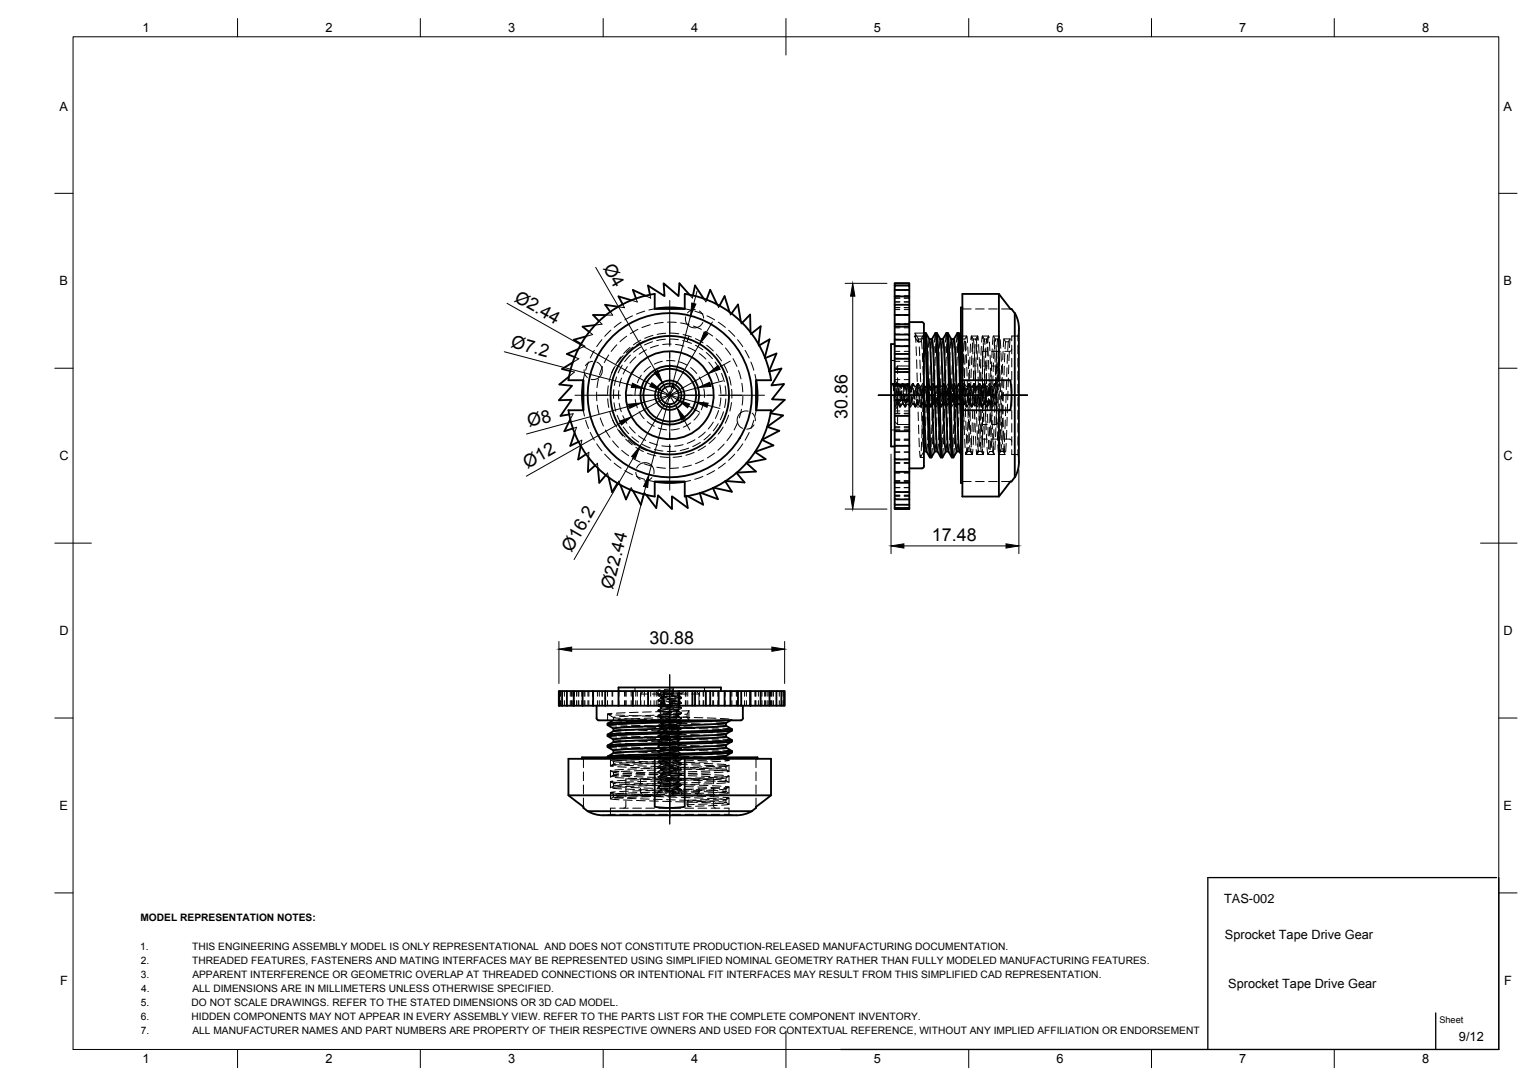
ISO-10303-21;
HEADER;
/* Generated by software containing ST-Developer
 * from STEP Tools, Inc. (www.steptools.com) 
 */

FILE_DESCRIPTION(
/* description */ ('STEP AP214'),
/* implementation_level */ '2;1');

FILE_NAME(
/* name */ 'Sprocket Tape Drive Gear.step',
/* time_stamp */ '2026-11-04T19:38:14-08:00',
/* author */ (''),
/* organization */ (''),
/* preprocessor_version */ 'ST-DEVELOPER v20.2',
/* originating_system */ 'Autodesk Translation Framework v15.17.0.0',
/* authorisation */ '');

FILE_SCHEMA (('AUTOMOTIVE_DESIGN { 1 0 10303 214 3 1 1 }'));
ENDSEC;

DATA;
#10=MECHANICAL_DESIGN_GEOMETRIC_PRESENTATION_REPRESENTATION('',(#476),#36668);
#59=(
BOUNDED_CURVE()
B_SPLINE_CURVE(2,(#28963,#28964,#28965,#28966,#28967,#28968,#28969),
 .UNSPECIFIED.,.F.,.F.)
B_SPLINE_CURVE_WITH_KNOTS((3,2,2,3),(0.975,0.983333333333333,0.991666666666667,
1.),.UNSPECIFIED.)
CURVE()
GEOMETRIC_REPRESENTATION_ITEM()
RATIONAL_B_SPLINE_CURVE((1.,0.866025403784439,1.,0.866025403784439,1.,0.866025403784439,
1.))
REPRESENTATION_ITEM('')
);
#60=(
BOUNDED_CURVE()
B_SPLINE_CURVE(2,(#28975,#28976,#28977,#28978,#28979,#28980,#28981),
 .UNSPECIFIED.,.F.,.F.)
B_SPLINE_CURVE_WITH_KNOTS((3,2,2,3),(0.975,0.983333333333333,0.991666666666667,
1.),.UNSPECIFIED.)
CURVE()
GEOMETRIC_REPRESENTATION_ITEM()
RATIONAL_B_SPLINE_CURVE((1.,0.866025403784439,1.,0.866025403784439,1.,0.866025403784439,
1.))
REPRESENTATION_ITEM('')
);
#61=(
BOUNDED_CURVE()
B_SPLINE_CURVE(2,(#28984,#28985,#28986,#28987,#28988,#28989,#28990),
 .UNSPECIFIED.,.F.,.F.)
B_SPLINE_CURVE_WITH_KNOTS((3,2,2,3),(0.975,0.983333333333333,0.991666666666667,
1.),.UNSPECIFIED.)
CURVE()
GEOMETRIC_REPRESENTATION_ITEM()
RATIONAL_B_SPLINE_CURVE((1.,0.866025403784439,1.,0.866025403784439,1.,0.866025403784439,
1.))
REPRESENTATION_ITEM('')
);
#62=(
BOUNDED_CURVE()
B_SPLINE_CURVE(2,(#28995,#28996,#28997,#28998,#28999,#29000,#29001,#29002,
#29003,#29004,#29005,#29006,#29007),.UNSPECIFIED.,.F.,.F.)
B_SPLINE_CURVE_WITH_KNOTS((3,2,2,2,2,2,3),(0.925,0.933333333333333,0.941666666666667,
0.95,0.958333333333333,0.966666666666667,0.975),.UNSPECIFIED.)
CURVE()
GEOMETRIC_REPRESENTATION_ITEM()
RATIONAL_B_SPLINE_CURVE((1.,0.866025403784439,1.,0.866025403784439,1.,0.866025403784439,
1.,0.866025403784439,1.,0.866025403784439,1.,0.866025403784439,1.))
REPRESENTATION_ITEM('')
);
#63=(
BOUNDED_CURVE()
B_SPLINE_CURVE(2,(#29008,#29009,#29010,#29011,#29012,#29013,#29014,#29015,
#29016,#29017,#29018,#29019,#29020),.UNSPECIFIED.,.F.,.F.)
B_SPLINE_CURVE_WITH_KNOTS((3,2,2,2,2,2,3),(0.925,0.933333333333333,0.941666666666667,
0.95,0.958333333333333,0.966666666666667,0.975),.UNSPECIFIED.)
CURVE()
GEOMETRIC_REPRESENTATION_ITEM()
RATIONAL_B_SPLINE_CURVE((1.,0.866025403784439,1.,0.866025403784439,1.,0.866025403784439,
1.,0.866025403784439,1.,0.866025403784439,1.,0.866025403784439,1.))
REPRESENTATION_ITEM('')
);
#64=(
BOUNDED_CURVE()
B_SPLINE_CURVE(2,(#29025,#29026,#29027,#29028,#29029,#29030,#29031,#29032,
#29033,#29034,#29035,#29036,#29037),.UNSPECIFIED.,.F.,.F.)
B_SPLINE_CURVE_WITH_KNOTS((3,2,2,2,2,2,3),(0.875,0.883333333333333,0.891666666666667,
0.9,0.908333333333333,0.916666666666667,0.925),.UNSPECIFIED.)
CURVE()
GEOMETRIC_REPRESENTATION_ITEM()
RATIONAL_B_SPLINE_CURVE((1.,0.866025403784439,1.,0.866025403784439,1.,0.866025403784439,
1.,0.866025403784439,1.,0.866025403784439,1.,0.866025403784439,1.))
REPRESENTATION_ITEM('')
);
#65=(
BOUNDED_CURVE()
B_SPLINE_CURVE(2,(#29038,#29039,#29040,#29041,#29042,#29043,#29044,#29045,
#29046,#29047,#29048,#29049,#29050),.UNSPECIFIED.,.F.,.F.)
B_SPLINE_CURVE_WITH_KNOTS((3,2,2,2,2,2,3),(0.875,0.883333333333333,0.891666666666667,
0.9,0.908333333333333,0.916666666666667,0.925),.UNSPECIFIED.)
CURVE()
GEOMETRIC_REPRESENTATION_ITEM()
RATIONAL_B_SPLINE_CURVE((1.,0.866025403784439,1.,0.866025403784439,1.,0.866025403784439,
1.,0.866025403784439,1.,0.866025403784439,1.,0.866025403784439,1.))
REPRESENTATION_ITEM('')
);
#66=(
BOUNDED_CURVE()
B_SPLINE_CURVE(2,(#29055,#29056,#29057,#29058,#29059,#29060,#29061,#29062,
#29063,#29064,#29065,#29066,#29067),.UNSPECIFIED.,.F.,.F.)
B_SPLINE_CURVE_WITH_KNOTS((3,2,2,2,2,2,3),(0.825,0.833333333333333,0.841666666666667,
0.85,0.858333333333333,0.866666666666667,0.875),.UNSPECIFIED.)
CURVE()
GEOMETRIC_REPRESENTATION_ITEM()
RATIONAL_B_SPLINE_CURVE((1.,0.866025403784439,1.,0.866025403784439,1.,0.866025403784439,
1.,0.866025403784439,1.,0.866025403784439,1.,0.866025403784439,1.))
REPRESENTATION_ITEM('')
);
#67=(
BOUNDED_CURVE()
B_SPLINE_CURVE(2,(#29068,#29069,#29070,#29071,#29072,#29073,#29074,#29075,
#29076,#29077,#29078,#29079,#29080),.UNSPECIFIED.,.F.,.F.)
B_SPLINE_CURVE_WITH_KNOTS((3,2,2,2,2,2,3),(0.825,0.833333333333333,0.841666666666667,
0.85,0.858333333333333,0.866666666666667,0.875),.UNSPECIFIED.)
CURVE()
GEOMETRIC_REPRESENTATION_ITEM()
RATIONAL_B_SPLINE_CURVE((1.,0.866025403784439,1.,0.866025403784439,1.,0.866025403784439,
1.,0.866025403784439,1.,0.866025403784439,1.,0.866025403784439,1.))
REPRESENTATION_ITEM('')
);
#68=(
BOUNDED_CURVE()
B_SPLINE_CURVE(2,(#29085,#29086,#29087,#29088,#29089,#29090,#29091,#29092,
#29093,#29094,#29095,#29096,#29097),.UNSPECIFIED.,.F.,.F.)
B_SPLINE_CURVE_WITH_KNOTS((3,2,2,2,2,2,3),(0.775,0.783333333333333,0.791666666666667,
0.8,0.808333333333333,0.816666666666667,0.825),.UNSPECIFIED.)
CURVE()
GEOMETRIC_REPRESENTATION_ITEM()
RATIONAL_B_SPLINE_CURVE((1.,0.866025403784439,1.,0.866025403784439,1.,0.866025403784439,
1.,0.866025403784439,1.,0.866025403784439,1.,0.866025403784439,1.))
REPRESENTATION_ITEM('')
);
#69=(
BOUNDED_CURVE()
B_SPLINE_CURVE(2,(#29098,#29099,#29100,#29101,#29102,#29103,#29104,#29105,
#29106,#29107,#29108,#29109,#29110),.UNSPECIFIED.,.F.,.F.)
B_SPLINE_CURVE_WITH_KNOTS((3,2,2,2,2,2,3),(0.775,0.783333333333333,0.791666666666667,
0.8,0.808333333333333,0.816666666666667,0.825),.UNSPECIFIED.)
CURVE()
GEOMETRIC_REPRESENTATION_ITEM()
RATIONAL_B_SPLINE_CURVE((1.,0.866025403784439,1.,0.866025403784439,1.,0.866025403784439,
1.,0.866025403784439,1.,0.866025403784439,1.,0.866025403784439,1.))
REPRESENTATION_ITEM('')
);
#70=(
BOUNDED_CURVE()
B_SPLINE_CURVE(2,(#29115,#29116,#29117,#29118,#29119,#29120,#29121,#29122,
#29123,#29124,#29125,#29126,#29127),.UNSPECIFIED.,.F.,.F.)
B_SPLINE_CURVE_WITH_KNOTS((3,2,2,2,2,2,3),(0.725,0.733333333333333,0.741666666666667,
0.75,0.758333333333333,0.766666666666667,0.775),.UNSPECIFIED.)
CURVE()
GEOMETRIC_REPRESENTATION_ITEM()
RATIONAL_B_SPLINE_CURVE((1.,0.866025403784439,1.,0.866025403784439,1.,0.866025403784439,
1.,0.866025403784439,1.,0.866025403784439,1.,0.866025403784439,1.))
REPRESENTATION_ITEM('')
);
#71=(
BOUNDED_CURVE()
B_SPLINE_CURVE(2,(#29128,#29129,#29130,#29131,#29132,#29133,#29134,#29135,
#29136,#29137,#29138,#29139,#29140),.UNSPECIFIED.,.F.,.F.)
B_SPLINE_CURVE_WITH_KNOTS((3,2,2,2,2,2,3),(0.725,0.733333333333333,0.741666666666667,
0.75,0.758333333333333,0.766666666666667,0.775),.UNSPECIFIED.)
CURVE()
GEOMETRIC_REPRESENTATION_ITEM()
RATIONAL_B_SPLINE_CURVE((1.,0.866025403784439,1.,0.866025403784439,1.,0.866025403784439,
1.,0.866025403784439,1.,0.866025403784439,1.,0.866025403784439,1.))
REPRESENTATION_ITEM('')
);
#72=(
BOUNDED_CURVE()
B_SPLINE_CURVE(2,(#29145,#29146,#29147,#29148,#29149,#29150,#29151,#29152,
#29153,#29154,#29155,#29156,#29157),.UNSPECIFIED.,.F.,.F.)
B_SPLINE_CURVE_WITH_KNOTS((3,2,2,2,2,2,3),(0.675,0.683333333333333,0.691666666666667,
0.7,0.708333333333333,0.716666666666667,0.725),.UNSPECIFIED.)
CURVE()
GEOMETRIC_REPRESENTATION_ITEM()
RATIONAL_B_SPLINE_CURVE((1.,0.866025403784439,1.,0.866025403784439,1.,0.866025403784439,
1.,0.866025403784439,1.,0.866025403784439,1.,0.866025403784439,1.))
REPRESENTATION_ITEM('')
);
#73=(
BOUNDED_CURVE()
B_SPLINE_CURVE(2,(#29158,#29159,#29160,#29161,#29162,#29163,#29164,#29165,
#29166,#29167,#29168,#29169,#29170),.UNSPECIFIED.,.F.,.F.)
B_SPLINE_CURVE_WITH_KNOTS((3,2,2,2,2,2,3),(0.675,0.683333333333333,0.691666666666667,
0.7,0.708333333333333,0.716666666666667,0.725),.UNSPECIFIED.)
CURVE()
GEOMETRIC_REPRESENTATION_ITEM()
RATIONAL_B_SPLINE_CURVE((1.,0.866025403784439,1.,0.866025403784439,1.,0.866025403784439,
1.,0.866025403784439,1.,0.866025403784439,1.,0.866025403784439,1.))
REPRESENTATION_ITEM('')
);
#74=(
BOUNDED_CURVE()
B_SPLINE_CURVE(2,(#29175,#29176,#29177,#29178,#29179,#29180,#29181,#29182,
#29183,#29184,#29185,#29186,#29187),.UNSPECIFIED.,.F.,.F.)
B_SPLINE_CURVE_WITH_KNOTS((3,2,2,2,2,2,3),(0.625,0.633333333333333,0.641666666666667,
0.65,0.658333333333333,0.666666666666667,0.675),.UNSPECIFIED.)
CURVE()
GEOMETRIC_REPRESENTATION_ITEM()
RATIONAL_B_SPLINE_CURVE((1.,0.866025403784439,1.,0.866025403784439,1.,0.866025403784439,
1.,0.866025403784439,1.,0.866025403784439,1.,0.866025403784439,1.))
REPRESENTATION_ITEM('')
);
#75=(
BOUNDED_CURVE()
B_SPLINE_CURVE(2,(#29188,#29189,#29190,#29191,#29192,#29193,#29194,#29195,
#29196,#29197,#29198,#29199,#29200),.UNSPECIFIED.,.F.,.F.)
B_SPLINE_CURVE_WITH_KNOTS((3,2,2,2,2,2,3),(0.625,0.633333333333333,0.641666666666667,
0.65,0.658333333333333,0.666666666666667,0.675),.UNSPECIFIED.)
CURVE()
GEOMETRIC_REPRESENTATION_ITEM()
RATIONAL_B_SPLINE_CURVE((1.,0.866025403784439,1.,0.866025403784439,1.,0.866025403784439,
1.,0.866025403784439,1.,0.866025403784439,1.,0.866025403784439,1.))
REPRESENTATION_ITEM('')
);
#76=(
BOUNDED_CURVE()
B_SPLINE_CURVE(2,(#29205,#29206,#29207,#29208,#29209,#29210,#29211,#29212,
#29213,#29214,#29215,#29216,#29217),.UNSPECIFIED.,.F.,.F.)
B_SPLINE_CURVE_WITH_KNOTS((3,2,2,2,2,2,3),(0.575,0.583333333333333,0.591666666666667,
0.6,0.608333333333333,0.616666666666667,0.625),.UNSPECIFIED.)
CURVE()
GEOMETRIC_REPRESENTATION_ITEM()
RATIONAL_B_SPLINE_CURVE((1.,0.866025403784439,1.,0.866025403784439,1.,0.866025403784439,
1.,0.866025403784439,1.,0.866025403784439,1.,0.866025403784439,1.))
REPRESENTATION_ITEM('')
);
#77=(
BOUNDED_CURVE()
B_SPLINE_CURVE(2,(#29218,#29219,#29220,#29221,#29222,#29223,#29224,#29225,
#29226,#29227,#29228,#29229,#29230),.UNSPECIFIED.,.F.,.F.)
B_SPLINE_CURVE_WITH_KNOTS((3,2,2,2,2,2,3),(0.575,0.583333333333333,0.591666666666667,
0.6,0.608333333333333,0.616666666666667,0.625),.UNSPECIFIED.)
CURVE()
GEOMETRIC_REPRESENTATION_ITEM()
RATIONAL_B_SPLINE_CURVE((1.,0.866025403784439,1.,0.866025403784439,1.,0.866025403784439,
1.,0.866025403784439,1.,0.866025403784439,1.,0.866025403784439,1.))
REPRESENTATION_ITEM('')
);
#78=(
BOUNDED_CURVE()
B_SPLINE_CURVE(2,(#29235,#29236,#29237,#29238,#29239,#29240,#29241,#29242,
#29243,#29244,#29245,#29246,#29247),.UNSPECIFIED.,.F.,.F.)
B_SPLINE_CURVE_WITH_KNOTS((3,2,2,2,2,2,3),(0.525,0.533333333333333,0.541666666666667,
0.55,0.558333333333333,0.566666666666667,0.575),.UNSPECIFIED.)
CURVE()
GEOMETRIC_REPRESENTATION_ITEM()
RATIONAL_B_SPLINE_CURVE((1.,0.866025403784439,1.,0.866025403784439,1.,0.866025403784439,
1.,0.866025403784439,1.,0.866025403784439,1.,0.866025403784439,1.))
REPRESENTATION_ITEM('')
);
#79=(
BOUNDED_CURVE()
B_SPLINE_CURVE(2,(#29248,#29249,#29250,#29251,#29252,#29253,#29254,#29255,
#29256,#29257,#29258,#29259,#29260),.UNSPECIFIED.,.F.,.F.)
B_SPLINE_CURVE_WITH_KNOTS((3,2,2,2,2,2,3),(0.525,0.533333333333333,0.541666666666667,
0.55,0.558333333333333,0.566666666666667,0.575),.UNSPECIFIED.)
CURVE()
GEOMETRIC_REPRESENTATION_ITEM()
RATIONAL_B_SPLINE_CURVE((1.,0.866025403784439,1.,0.866025403784439,1.,0.866025403784439,
1.,0.866025403784439,1.,0.866025403784439,1.,0.866025403784439,1.))
REPRESENTATION_ITEM('')
);
#80=(
BOUNDED_CURVE()
B_SPLINE_CURVE(2,(#29265,#29266,#29267,#29268,#29269,#29270,#29271,#29272,
#29273,#29274,#29275,#29276,#29277),.UNSPECIFIED.,.F.,.F.)
B_SPLINE_CURVE_WITH_KNOTS((3,2,2,2,2,2,3),(0.475,0.483333333333333,0.491666666666667,
0.5,0.508333333333333,0.516666666666667,0.525),.UNSPECIFIED.)
CURVE()
GEOMETRIC_REPRESENTATION_ITEM()
RATIONAL_B_SPLINE_CURVE((1.,0.866025403784439,1.,0.866025403784439,1.,0.866025403784439,
1.,0.866025403784439,1.,0.866025403784439,1.,0.866025403784439,1.))
REPRESENTATION_ITEM('')
);
#81=(
BOUNDED_CURVE()
B_SPLINE_CURVE(2,(#29278,#29279,#29280,#29281,#29282,#29283,#29284,#29285,
#29286,#29287,#29288,#29289,#29290),.UNSPECIFIED.,.F.,.F.)
B_SPLINE_CURVE_WITH_KNOTS((3,2,2,2,2,2,3),(0.475,0.483333333333333,0.491666666666667,
0.5,0.508333333333333,0.516666666666667,0.525),.UNSPECIFIED.)
CURVE()
GEOMETRIC_REPRESENTATION_ITEM()
RATIONAL_B_SPLINE_CURVE((1.,0.866025403784439,1.,0.866025403784439,1.,0.866025403784439,
1.,0.866025403784439,1.,0.866025403784439,1.,0.866025403784439,1.))
REPRESENTATION_ITEM('')
);
#82=(
BOUNDED_CURVE()
B_SPLINE_CURVE(2,(#29295,#29296,#29297,#29298,#29299,#29300,#29301,#29302,
#29303,#29304,#29305,#29306,#29307),.UNSPECIFIED.,.F.,.F.)
B_SPLINE_CURVE_WITH_KNOTS((3,2,2,2,2,2,3),(0.425,0.433333333333334,0.441666666666666,
0.45,0.458333333333333,0.466666666666667,0.475),.UNSPECIFIED.)
CURVE()
GEOMETRIC_REPRESENTATION_ITEM()
RATIONAL_B_SPLINE_CURVE((1.,0.866025403784439,1.,0.866025403784439,1.,0.866025403784439,
1.,0.866025403784439,1.,0.866025403784439,1.,0.866025403784439,1.))
REPRESENTATION_ITEM('')
);
#83=(
BOUNDED_CURVE()
B_SPLINE_CURVE(2,(#29308,#29309,#29310,#29311,#29312,#29313,#29314,#29315,
#29316,#29317,#29318,#29319,#29320),.UNSPECIFIED.,.F.,.F.)
B_SPLINE_CURVE_WITH_KNOTS((3,2,2,2,2,2,3),(0.425,0.433333333333334,0.441666666666666,
0.45,0.458333333333333,0.466666666666667,0.475),.UNSPECIFIED.)
CURVE()
GEOMETRIC_REPRESENTATION_ITEM()
RATIONAL_B_SPLINE_CURVE((1.,0.866025403784439,1.,0.866025403784439,1.,0.866025403784439,
1.,0.866025403784439,1.,0.866025403784439,1.,0.866025403784439,1.))
REPRESENTATION_ITEM('')
);
#84=(
BOUNDED_CURVE()
B_SPLINE_CURVE(2,(#29325,#29326,#29327,#29328,#29329,#29330,#29331,#29332,
#29333,#29334,#29335,#29336,#29337),.UNSPECIFIED.,.F.,.F.)
B_SPLINE_CURVE_WITH_KNOTS((3,2,2,2,2,2,3),(0.375,0.383333333333334,0.391666666666666,
0.4,0.408333333333334,0.416666666666667,0.425),.UNSPECIFIED.)
CURVE()
GEOMETRIC_REPRESENTATION_ITEM()
RATIONAL_B_SPLINE_CURVE((1.,0.866025403784439,1.,0.866025403784439,1.,0.866025403784439,
1.,0.866025403784439,1.,0.866025403784439,1.,0.866025403784439,1.))
REPRESENTATION_ITEM('')
);
#85=(
BOUNDED_CURVE()
B_SPLINE_CURVE(2,(#29338,#29339,#29340,#29341,#29342,#29343,#29344,#29345,
#29346,#29347,#29348,#29349,#29350),.UNSPECIFIED.,.F.,.F.)
B_SPLINE_CURVE_WITH_KNOTS((3,2,2,2,2,2,3),(0.375,0.383333333333334,0.391666666666666,
0.4,0.408333333333334,0.416666666666667,0.425),.UNSPECIFIED.)
CURVE()
GEOMETRIC_REPRESENTATION_ITEM()
RATIONAL_B_SPLINE_CURVE((1.,0.866025403784439,1.,0.866025403784439,1.,0.866025403784439,
1.,0.866025403784439,1.,0.866025403784439,1.,0.866025403784439,1.))
REPRESENTATION_ITEM('')
);
#86=(
BOUNDED_CURVE()
B_SPLINE_CURVE(2,(#29355,#29356,#29357,#29358,#29359,#29360,#29361,#29362,
#29363,#29364,#29365,#29366,#29367),.UNSPECIFIED.,.F.,.F.)
B_SPLINE_CURVE_WITH_KNOTS((3,2,2,2,2,2,3),(0.325,0.333333333333334,0.341666666666667,
0.35,0.358333333333334,0.366666666666666,0.375),.UNSPECIFIED.)
CURVE()
GEOMETRIC_REPRESENTATION_ITEM()
RATIONAL_B_SPLINE_CURVE((1.,0.866025403784439,1.,0.866025403784439,1.,0.866025403784439,
1.,0.866025403784439,1.,0.866025403784439,1.,0.866025403784439,1.))
REPRESENTATION_ITEM('')
);
#87=(
BOUNDED_CURVE()
B_SPLINE_CURVE(2,(#29368,#29369,#29370,#29371,#29372,#29373,#29374,#29375,
#29376,#29377,#29378,#29379,#29380),.UNSPECIFIED.,.F.,.F.)
B_SPLINE_CURVE_WITH_KNOTS((3,2,2,2,2,2,3),(0.325,0.333333333333334,0.341666666666667,
0.35,0.358333333333334,0.366666666666666,0.375),.UNSPECIFIED.)
CURVE()
GEOMETRIC_REPRESENTATION_ITEM()
RATIONAL_B_SPLINE_CURVE((1.,0.866025403784439,1.,0.866025403784439,1.,0.866025403784439,
1.,0.866025403784439,1.,0.866025403784439,1.,0.866025403784439,1.))
REPRESENTATION_ITEM('')
);
#88=(
BOUNDED_CURVE()
B_SPLINE_CURVE(2,(#29385,#29386,#29387,#29388,#29389,#29390,#29391,#29392,
#29393,#29394,#29395,#29396,#29397),.UNSPECIFIED.,.F.,.F.)
B_SPLINE_CURVE_WITH_KNOTS((3,2,2,2,2,2,3),(0.275,0.283333333333334,0.291666666666667,
0.3,0.308333333333334,0.316666666666666,0.325),.UNSPECIFIED.)
CURVE()
GEOMETRIC_REPRESENTATION_ITEM()
RATIONAL_B_SPLINE_CURVE((1.,0.866025403784439,1.,0.866025403784439,1.,0.866025403784439,
1.,0.866025403784439,1.,0.866025403784439,1.,0.866025403784439,1.))
REPRESENTATION_ITEM('')
);
#89=(
BOUNDED_CURVE()
B_SPLINE_CURVE(2,(#29398,#29399,#29400,#29401,#29402,#29403,#29404,#29405,
#29406,#29407,#29408,#29409,#29410),.UNSPECIFIED.,.F.,.F.)
B_SPLINE_CURVE_WITH_KNOTS((3,2,2,2,2,2,3),(0.275,0.283333333333334,0.291666666666667,
0.3,0.308333333333334,0.316666666666666,0.325),.UNSPECIFIED.)
CURVE()
GEOMETRIC_REPRESENTATION_ITEM()
RATIONAL_B_SPLINE_CURVE((1.,0.866025403784439,1.,0.866025403784439,1.,0.866025403784439,
1.,0.866025403784439,1.,0.866025403784439,1.,0.866025403784439,1.))
REPRESENTATION_ITEM('')
);
#90=(
BOUNDED_CURVE()
B_SPLINE_CURVE(2,(#29415,#29416,#29417,#29418,#29419,#29420,#29421,#29422,
#29423,#29424,#29425,#29426,#29427),.UNSPECIFIED.,.F.,.F.)
B_SPLINE_CURVE_WITH_KNOTS((3,2,2,2,2,2,3),(0.225,0.233333333333334,0.241666666666667,
0.25,0.258333333333334,0.266666666666666,0.275),.UNSPECIFIED.)
CURVE()
GEOMETRIC_REPRESENTATION_ITEM()
RATIONAL_B_SPLINE_CURVE((1.,0.866025403784439,1.,0.866025403784439,1.,0.866025403784439,
1.,0.866025403784439,1.,0.866025403784439,1.,0.866025403784439,1.))
REPRESENTATION_ITEM('')
);
#91=(
BOUNDED_CURVE()
B_SPLINE_CURVE(2,(#29428,#29429,#29430,#29431,#29432,#29433,#29434,#29435,
#29436,#29437,#29438,#29439,#29440),.UNSPECIFIED.,.F.,.F.)
B_SPLINE_CURVE_WITH_KNOTS((3,2,2,2,2,2,3),(0.225,0.233333333333334,0.241666666666667,
0.25,0.258333333333334,0.266666666666666,0.275),.UNSPECIFIED.)
CURVE()
GEOMETRIC_REPRESENTATION_ITEM()
RATIONAL_B_SPLINE_CURVE((1.,0.866025403784439,1.,0.866025403784439,1.,0.866025403784439,
1.,0.866025403784439,1.,0.866025403784439,1.,0.866025403784439,1.))
REPRESENTATION_ITEM('')
);
#92=(
BOUNDED_CURVE()
B_SPLINE_CURVE(2,(#29445,#29446,#29447,#29448,#29449,#29450,#29451,#29452,
#29453,#29454,#29455,#29456,#29457),.UNSPECIFIED.,.F.,.F.)
B_SPLINE_CURVE_WITH_KNOTS((3,2,2,2,2,2,3),(0.175,0.183333333333334,0.191666666666667,
0.2,0.208333333333334,0.216666666666667,0.225),.UNSPECIFIED.)
CURVE()
GEOMETRIC_REPRESENTATION_ITEM()
RATIONAL_B_SPLINE_CURVE((1.,0.866025403784439,1.,0.866025403784439,1.,0.866025403784439,
1.,0.866025403784439,1.,0.866025403784439,1.,0.866025403784439,1.))
REPRESENTATION_ITEM('')
);
#93=(
BOUNDED_CURVE()
B_SPLINE_CURVE(2,(#29458,#29459,#29460,#29461,#29462,#29463,#29464,#29465,
#29466,#29467,#29468,#29469,#29470),.UNSPECIFIED.,.F.,.F.)
B_SPLINE_CURVE_WITH_KNOTS((3,2,2,2,2,2,3),(0.175,0.183333333333334,0.191666666666667,
0.2,0.208333333333334,0.216666666666667,0.225),.UNSPECIFIED.)
CURVE()
GEOMETRIC_REPRESENTATION_ITEM()
RATIONAL_B_SPLINE_CURVE((1.,0.866025403784439,1.,0.866025403784439,1.,0.866025403784439,
1.,0.866025403784439,1.,0.866025403784439,1.,0.866025403784439,1.))
REPRESENTATION_ITEM('')
);
#94=(
BOUNDED_CURVE()
B_SPLINE_CURVE(2,(#29475,#29476,#29477,#29478,#29479,#29480,#29481,#29482,
#29483,#29484,#29485,#29486,#29487),.UNSPECIFIED.,.F.,.F.)
B_SPLINE_CURVE_WITH_KNOTS((3,2,2,2,2,2,3),(0.125,0.133333333333333,0.141666666666667,
0.15,0.158333333333333,0.166666666666667,0.175),.UNSPECIFIED.)
CURVE()
GEOMETRIC_REPRESENTATION_ITEM()
RATIONAL_B_SPLINE_CURVE((1.,0.866025403784439,1.,0.866025403784439,1.,0.866025403784439,
1.,0.866025403784439,1.,0.866025403784439,1.,0.866025403784439,1.))
REPRESENTATION_ITEM('')
);
#95=(
BOUNDED_CURVE()
B_SPLINE_CURVE(2,(#29488,#29489,#29490,#29491,#29492,#29493,#29494,#29495,
#29496,#29497,#29498,#29499,#29500),.UNSPECIFIED.,.F.,.F.)
B_SPLINE_CURVE_WITH_KNOTS((3,2,2,2,2,2,3),(0.125,0.133333333333333,0.141666666666667,
0.15,0.158333333333333,0.166666666666667,0.175),.UNSPECIFIED.)
CURVE()
GEOMETRIC_REPRESENTATION_ITEM()
RATIONAL_B_SPLINE_CURVE((1.,0.866025403784439,1.,0.866025403784439,1.,0.866025403784439,
1.,0.866025403784439,1.,0.866025403784439,1.,0.866025403784439,1.))
REPRESENTATION_ITEM('')
);
#96=(
BOUNDED_CURVE()
B_SPLINE_CURVE(2,(#29505,#29506,#29507,#29508,#29509,#29510,#29511,#29512,
#29513,#29514,#29515,#29516,#29517),.UNSPECIFIED.,.F.,.F.)
B_SPLINE_CURVE_WITH_KNOTS((3,2,2,2,2,2,3),(0.075,0.0833333333333333,0.0916666666666667,
0.1,0.108333333333333,0.116666666666667,0.125),.UNSPECIFIED.)
CURVE()
GEOMETRIC_REPRESENTATION_ITEM()
RATIONAL_B_SPLINE_CURVE((1.,0.866025403784439,1.,0.866025403784439,1.,0.866025403784439,
1.,0.866025403784439,1.,0.866025403784439,1.,0.866025403784439,1.))
REPRESENTATION_ITEM('')
);
#97=(
BOUNDED_CURVE()
B_SPLINE_CURVE(2,(#29518,#29519,#29520,#29521,#29522,#29523,#29524,#29525,
#29526,#29527,#29528,#29529,#29530),.UNSPECIFIED.,.F.,.F.)
B_SPLINE_CURVE_WITH_KNOTS((3,2,2,2,2,2,3),(0.075,0.0833333333333333,0.0916666666666667,
0.1,0.108333333333333,0.116666666666667,0.125),.UNSPECIFIED.)
CURVE()
GEOMETRIC_REPRESENTATION_ITEM()
RATIONAL_B_SPLINE_CURVE((1.,0.866025403784439,1.,0.866025403784439,1.,0.866025403784439,
1.,0.866025403784439,1.,0.866025403784439,1.,0.866025403784439,1.))
REPRESENTATION_ITEM('')
);
#98=(
BOUNDED_CURVE()
B_SPLINE_CURVE(2,(#29536,#29537,#29538,#29539,#29540,#29541,#29542),
 .UNSPECIFIED.,.F.,.F.)
B_SPLINE_CURVE_WITH_KNOTS((3,2,2,3),(0.,0.00833333333333333,0.0166666666666666,
0.025),.UNSPECIFIED.)
CURVE()
GEOMETRIC_REPRESENTATION_ITEM()
RATIONAL_B_SPLINE_CURVE((1.,0.866025403784439,1.,0.866025403784439,1.,0.866025403784439,
1.))
REPRESENTATION_ITEM('')
);
#99=(
BOUNDED_CURVE()
B_SPLINE_CURVE(2,(#29545,#29546,#29547,#29548,#29549,#29550,#29551),
 .UNSPECIFIED.,.F.,.F.)
B_SPLINE_CURVE_WITH_KNOTS((3,2,2,3),(0.,0.00833333333333333,0.0166666666666666,
0.025),.UNSPECIFIED.)
CURVE()
GEOMETRIC_REPRESENTATION_ITEM()
RATIONAL_B_SPLINE_CURVE((1.,0.866025403784439,1.,0.866025403784439,1.,0.866025403784439,
1.))
REPRESENTATION_ITEM('')
);
#100=(
BOUNDED_CURVE()
B_SPLINE_CURVE(2,(#29776,#29777,#29778,#29779,#29780,#29781,#29782,#29783,
#29784),.UNSPECIFIED.,.F.,.F.)
B_SPLINE_CURVE_WITH_KNOTS((3,2,2,2,3),(0.9375,0.953125,0.96875,0.984375,
1.),.UNSPECIFIED.)
CURVE()
GEOMETRIC_REPRESENTATION_ITEM()
RATIONAL_B_SPLINE_CURVE((1.,0.923879532511287,1.,0.923879532511287,1.,0.923879532511287,
1.,0.923879532511287,1.))
REPRESENTATION_ITEM('')
);
#101=(
BOUNDED_CURVE()
B_SPLINE_CURVE(2,(#29787,#29788,#29789,#29790,#29791,#29792,#29793,#29794,
#29795),.UNSPECIFIED.,.F.,.F.)
B_SPLINE_CURVE_WITH_KNOTS((3,2,2,2,3),(0.9375,0.953125,0.96875,0.984375,
1.),.UNSPECIFIED.)
CURVE()
GEOMETRIC_REPRESENTATION_ITEM()
RATIONAL_B_SPLINE_CURVE((1.,0.923879532511287,1.,0.923879532511287,1.,0.923879532511287,
1.,0.923879532511287,1.))
REPRESENTATION_ITEM('')
);
#102=(
BOUNDED_CURVE()
B_SPLINE_CURVE(2,(#29800,#29801,#29802,#29803,#29804,#29805,#29806,#29807,
#29808,#29809,#29810,#29811,#29812,#29813,#29814,#29815,#29816),
 .UNSPECIFIED.,.F.,.F.)
B_SPLINE_CURVE_WITH_KNOTS((3,2,2,2,2,2,2,2,3),(0.8125,0.828125,0.84375,
0.859375,0.875,0.890625,0.90625,0.921875,0.9375),.UNSPECIFIED.)
CURVE()
GEOMETRIC_REPRESENTATION_ITEM()
RATIONAL_B_SPLINE_CURVE((1.,0.923879532511287,1.,0.923879532511287,1.,0.923879532511287,
1.,0.923879532511287,1.,0.923879532511287,1.,0.923879532511287,1.,0.923879532511287,
1.,0.923879532511287,1.))
REPRESENTATION_ITEM('')
);
#103=(
BOUNDED_CURVE()
B_SPLINE_CURVE(2,(#29817,#29818,#29819,#29820,#29821,#29822,#29823,#29824,
#29825,#29826,#29827,#29828,#29829,#29830,#29831,#29832,#29833),
 .UNSPECIFIED.,.F.,.F.)
B_SPLINE_CURVE_WITH_KNOTS((3,2,2,2,2,2,2,2,3),(0.8125,0.828125,0.84375,
0.859375,0.875,0.890625,0.90625,0.921875,0.9375),.UNSPECIFIED.)
CURVE()
GEOMETRIC_REPRESENTATION_ITEM()
RATIONAL_B_SPLINE_CURVE((1.,0.923879532511287,1.,0.923879532511287,1.,0.923879532511287,
1.,0.923879532511287,1.,0.923879532511287,1.,0.923879532511287,1.,0.923879532511287,
1.,0.923879532511287,1.))
REPRESENTATION_ITEM('')
);
#104=(
BOUNDED_CURVE()
B_SPLINE_CURVE(2,(#29838,#29839,#29840,#29841,#29842,#29843,#29844,#29845,
#29846,#29847,#29848,#29849,#29850,#29851,#29852,#29853,#29854),
 .UNSPECIFIED.,.F.,.F.)
B_SPLINE_CURVE_WITH_KNOTS((3,2,2,2,2,2,2,2,3),(0.6875,0.703125,0.71875,
0.734375,0.75,0.765625,0.78125,0.796875,0.8125),.UNSPECIFIED.)
CURVE()
GEOMETRIC_REPRESENTATION_ITEM()
RATIONAL_B_SPLINE_CURVE((1.,0.923879532511287,1.,0.923879532511287,1.,0.923879532511287,
1.,0.923879532511287,1.,0.923879532511287,1.,0.923879532511287,1.,0.923879532511287,
1.,0.923879532511287,1.))
REPRESENTATION_ITEM('')
);
#105=(
BOUNDED_CURVE()
B_SPLINE_CURVE(2,(#29855,#29856,#29857,#29858,#29859,#29860,#29861,#29862,
#29863,#29864,#29865,#29866,#29867,#29868,#29869,#29870,#29871),
 .UNSPECIFIED.,.F.,.F.)
B_SPLINE_CURVE_WITH_KNOTS((3,2,2,2,2,2,2,2,3),(0.6875,0.703125,0.71875,
0.734375,0.75,0.765625,0.78125,0.796875,0.8125),.UNSPECIFIED.)
CURVE()
GEOMETRIC_REPRESENTATION_ITEM()
RATIONAL_B_SPLINE_CURVE((1.,0.923879532511287,1.,0.923879532511287,1.,0.923879532511287,
1.,0.923879532511287,1.,0.923879532511287,1.,0.923879532511287,1.,0.923879532511287,
1.,0.923879532511287,1.))
REPRESENTATION_ITEM('')
);
#106=(
BOUNDED_CURVE()
B_SPLINE_CURVE(2,(#29876,#29877,#29878,#29879,#29880,#29881,#29882,#29883,
#29884,#29885,#29886,#29887,#29888,#29889,#29890,#29891,#29892),
 .UNSPECIFIED.,.F.,.F.)
B_SPLINE_CURVE_WITH_KNOTS((3,2,2,2,2,2,2,2,3),(0.5625,0.578125,0.59375,
0.609375,0.625,0.640625,0.65625,0.671875,0.6875),.UNSPECIFIED.)
CURVE()
GEOMETRIC_REPRESENTATION_ITEM()
RATIONAL_B_SPLINE_CURVE((1.,0.923879532511287,1.,0.923879532511287,1.,0.923879532511287,
1.,0.923879532511287,1.,0.923879532511287,1.,0.923879532511287,1.,0.923879532511287,
1.,0.923879532511287,1.))
REPRESENTATION_ITEM('')
);
#107=(
BOUNDED_CURVE()
B_SPLINE_CURVE(2,(#29893,#29894,#29895,#29896,#29897,#29898,#29899,#29900,
#29901,#29902,#29903,#29904,#29905,#29906,#29907,#29908,#29909),
 .UNSPECIFIED.,.F.,.F.)
B_SPLINE_CURVE_WITH_KNOTS((3,2,2,2,2,2,2,2,3),(0.5625,0.578125,0.59375,
0.609375,0.625,0.640625,0.65625,0.671875,0.6875),.UNSPECIFIED.)
CURVE()
GEOMETRIC_REPRESENTATION_ITEM()
RATIONAL_B_SPLINE_CURVE((1.,0.923879532511287,1.,0.923879532511287,1.,0.923879532511287,
1.,0.923879532511287,1.,0.923879532511287,1.,0.923879532511287,1.,0.923879532511287,
1.,0.923879532511287,1.))
REPRESENTATION_ITEM('')
);
#108=(
BOUNDED_CURVE()
B_SPLINE_CURVE(2,(#29914,#29915,#29916,#29917,#29918,#29919,#29920,#29921,
#29922,#29923,#29924,#29925,#29926,#29927,#29928,#29929,#29930),
 .UNSPECIFIED.,.F.,.F.)
B_SPLINE_CURVE_WITH_KNOTS((3,2,2,2,2,2,2,2,3),(0.4375,0.453125,0.46875,
0.484375,0.5,0.515625,0.53125,0.546875,0.5625),.UNSPECIFIED.)
CURVE()
GEOMETRIC_REPRESENTATION_ITEM()
RATIONAL_B_SPLINE_CURVE((1.,0.923879532511287,1.,0.923879532511287,1.,0.923879532511287,
1.,0.923879532511287,1.,0.923879532511287,1.,0.923879532511287,1.,0.923879532511287,
1.,0.923879532511287,1.))
REPRESENTATION_ITEM('')
);
#109=(
BOUNDED_CURVE()
B_SPLINE_CURVE(2,(#29931,#29932,#29933,#29934,#29935,#29936,#29937,#29938,
#29939,#29940,#29941,#29942,#29943,#29944,#29945,#29946,#29947),
 .UNSPECIFIED.,.F.,.F.)
B_SPLINE_CURVE_WITH_KNOTS((3,2,2,2,2,2,2,2,3),(0.4375,0.453125,0.46875,
0.484375,0.5,0.515625,0.53125,0.546875,0.5625),.UNSPECIFIED.)
CURVE()
GEOMETRIC_REPRESENTATION_ITEM()
RATIONAL_B_SPLINE_CURVE((1.,0.923879532511287,1.,0.923879532511287,1.,0.923879532511287,
1.,0.923879532511287,1.,0.923879532511287,1.,0.923879532511287,1.,0.923879532511287,
1.,0.923879532511287,1.))
REPRESENTATION_ITEM('')
);
#110=(
BOUNDED_CURVE()
B_SPLINE_CURVE(2,(#29952,#29953,#29954,#29955,#29956,#29957,#29958,#29959,
#29960,#29961,#29962,#29963,#29964,#29965,#29966,#29967,#29968),
 .UNSPECIFIED.,.F.,.F.)
B_SPLINE_CURVE_WITH_KNOTS((3,2,2,2,2,2,2,2,3),(0.3125,0.328125,0.34375,
0.359375,0.375,0.390625,0.40625,0.421875,0.4375),.UNSPECIFIED.)
CURVE()
GEOMETRIC_REPRESENTATION_ITEM()
RATIONAL_B_SPLINE_CURVE((1.,0.923879532511287,1.,0.923879532511287,1.,0.923879532511287,
1.,0.923879532511287,1.,0.923879532511287,1.,0.923879532511287,1.,0.923879532511287,
1.,0.923879532511287,1.))
REPRESENTATION_ITEM('')
);
#111=(
BOUNDED_CURVE()
B_SPLINE_CURVE(2,(#29969,#29970,#29971,#29972,#29973,#29974,#29975,#29976,
#29977,#29978,#29979,#29980,#29981,#29982,#29983,#29984,#29985),
 .UNSPECIFIED.,.F.,.F.)
B_SPLINE_CURVE_WITH_KNOTS((3,2,2,2,2,2,2,2,3),(0.3125,0.328125,0.34375,
0.359375,0.375,0.390625,0.40625,0.421875,0.4375),.UNSPECIFIED.)
CURVE()
GEOMETRIC_REPRESENTATION_ITEM()
RATIONAL_B_SPLINE_CURVE((1.,0.923879532511287,1.,0.923879532511287,1.,0.923879532511287,
1.,0.923879532511287,1.,0.923879532511287,1.,0.923879532511287,1.,0.923879532511287,
1.,0.923879532511287,1.))
REPRESENTATION_ITEM('')
);
#112=(
BOUNDED_CURVE()
B_SPLINE_CURVE(2,(#29990,#29991,#29992,#29993,#29994,#29995,#29996,#29997,
#29998,#29999,#30000,#30001,#30002,#30003,#30004,#30005,#30006),
 .UNSPECIFIED.,.F.,.F.)
B_SPLINE_CURVE_WITH_KNOTS((3,2,2,2,2,2,2,2,3),(0.1875,0.203125,0.21875,
0.234375,0.25,0.265625,0.28125,0.296875,0.3125),.UNSPECIFIED.)
CURVE()
GEOMETRIC_REPRESENTATION_ITEM()
RATIONAL_B_SPLINE_CURVE((1.,0.923879532511287,1.,0.923879532511287,1.,0.923879532511287,
1.,0.923879532511287,1.,0.923879532511287,1.,0.923879532511287,1.,0.923879532511287,
1.,0.923879532511287,1.))
REPRESENTATION_ITEM('')
);
#113=(
BOUNDED_CURVE()
B_SPLINE_CURVE(2,(#30007,#30008,#30009,#30010,#30011,#30012,#30013,#30014,
#30015,#30016,#30017,#30018,#30019,#30020,#30021,#30022,#30023),
 .UNSPECIFIED.,.F.,.F.)
B_SPLINE_CURVE_WITH_KNOTS((3,2,2,2,2,2,2,2,3),(0.1875,0.203125,0.21875,
0.234375,0.25,0.265625,0.28125,0.296875,0.3125),.UNSPECIFIED.)
CURVE()
GEOMETRIC_REPRESENTATION_ITEM()
RATIONAL_B_SPLINE_CURVE((1.,0.923879532511287,1.,0.923879532511287,1.,0.923879532511287,
1.,0.923879532511287,1.,0.923879532511287,1.,0.923879532511287,1.,0.923879532511287,
1.,0.923879532511287,1.))
REPRESENTATION_ITEM('')
);
#114=(
BOUNDED_CURVE()
B_SPLINE_CURVE(2,(#30028,#30029,#30030,#30031,#30032,#30033,#30034,#30035,
#30036,#30037,#30038,#30039,#30040,#30041,#30042,#30043,#30044),
 .UNSPECIFIED.,.F.,.F.)
B_SPLINE_CURVE_WITH_KNOTS((3,2,2,2,2,2,2,2,3),(0.0625,0.078125,0.09375,
0.109375,0.125,0.140625,0.15625,0.171875,0.1875),.UNSPECIFIED.)
CURVE()
GEOMETRIC_REPRESENTATION_ITEM()
RATIONAL_B_SPLINE_CURVE((1.,0.923879532511287,1.,0.923879532511287,1.,0.923879532511287,
1.,0.923879532511287,1.,0.923879532511287,1.,0.923879532511287,1.,0.923879532511287,
1.,0.923879532511287,1.))
REPRESENTATION_ITEM('')
);
#115=(
BOUNDED_CURVE()
B_SPLINE_CURVE(2,(#30045,#30046,#30047,#30048,#30049,#30050,#30051,#30052,
#30053,#30054,#30055,#30056,#30057,#30058,#30059,#30060,#30061),
 .UNSPECIFIED.,.F.,.F.)
B_SPLINE_CURVE_WITH_KNOTS((3,2,2,2,2,2,2,2,3),(0.0625,0.078125,0.09375,
0.109375,0.125,0.140625,0.15625,0.171875,0.1875),.UNSPECIFIED.)
CURVE()
GEOMETRIC_REPRESENTATION_ITEM()
RATIONAL_B_SPLINE_CURVE((1.,0.923879532511287,1.,0.923879532511287,1.,0.923879532511287,
1.,0.923879532511287,1.,0.923879532511287,1.,0.923879532511287,1.,0.923879532511287,
1.,0.923879532511287,1.))
REPRESENTATION_ITEM('')
);
#116=(
BOUNDED_CURVE()
B_SPLINE_CURVE(2,(#30407,#30408,#30409),.UNSPECIFIED.,.F.,.F.)
B_SPLINE_CURVE_WITH_KNOTS((3,3),(-2.29029703823251,-1.6630480152671),
 .UNSPECIFIED.)
CURVE()
GEOMETRIC_REPRESENTATION_ITEM()
RATIONAL_B_SPLINE_CURVE((1.40847966848734,1.4295768207167,1.40847966848734))
REPRESENTATION_ITEM('')
);
#117=(
BOUNDED_CURVE()
B_SPLINE_CURVE(2,(#30414,#30415,#30416),.UNSPECIFIED.,.F.,.F.)
B_SPLINE_CURVE_WITH_KNOTS((3,3),(-0.660669052460662,-0.357639202089822),
 .UNSPECIFIED.)
CURVE()
GEOMETRIC_REPRESENTATION_ITEM()
RATIONAL_B_SPLINE_CURVE((1.03886559867011,1.03696952671266,1.02863628649672))
REPRESENTATION_ITEM('')
);
#118=(
BOUNDED_CURVE()
B_SPLINE_CURVE(2,(#30422,#30423,#30424),.UNSPECIFIED.,.F.,.F.)
B_SPLINE_CURVE_WITH_KNOTS((3,3),(-1.14221416870175,-0.839184318331155),
 .UNSPECIFIED.)
CURVE()
GEOMETRIC_REPRESENTATION_ITEM()
RATIONAL_B_SPLINE_CURVE((1.02863628649616,1.03696952671193,1.03886559866935))
REPRESENTATION_ITEM('')
);
#119=(
BOUNDED_CURVE()
B_SPLINE_CURVE(2,(#30440,#30441,#30442),.UNSPECIFIED.,.F.,.F.)
B_SPLINE_CURVE_WITH_KNOTS((3,3),(-1.14221416870072,-0.839184318329676),
 .UNSPECIFIED.)
CURVE()
GEOMETRIC_REPRESENTATION_ITEM()
RATIONAL_B_SPLINE_CURVE((1.02863628649697,1.03696952671296,1.0388655986704))
REPRESENTATION_ITEM('')
);
#120=(
BOUNDED_CURVE()
B_SPLINE_CURVE(2,(#30449,#30450,#30451),.UNSPECIFIED.,.F.,.F.)
B_SPLINE_CURVE_WITH_KNOTS((3,3),(-2.29029703823251,-1.6630480152671),
 .UNSPECIFIED.)
CURVE()
GEOMETRIC_REPRESENTATION_ITEM()
RATIONAL_B_SPLINE_CURVE((1.40847966848733,1.4295768207167,1.40847966848733))
REPRESENTATION_ITEM('')
);
#121=(
BOUNDED_CURVE()
B_SPLINE_CURVE(2,(#30455,#30456,#30457),.UNSPECIFIED.,.F.,.F.)
B_SPLINE_CURVE_WITH_KNOTS((3,3),(-0.660669052461382,-0.357639202090536),
 .UNSPECIFIED.)
CURVE()
GEOMETRIC_REPRESENTATION_ITEM()
RATIONAL_B_SPLINE_CURVE((1.03886559866973,1.03696952671232,1.02863628649648))
REPRESENTATION_ITEM('')
);
#122=(
BOUNDED_CURVE()
B_SPLINE_CURVE(2,(#30473,#30474,#30475),.UNSPECIFIED.,.F.,.F.)
B_SPLINE_CURVE_WITH_KNOTS((3,3),(-1.14221416870089,-0.839184318330394),
 .UNSPECIFIED.)
CURVE()
GEOMETRIC_REPRESENTATION_ITEM()
RATIONAL_B_SPLINE_CURVE((1.02863628649558,1.03696952671116,1.03886559866852))
REPRESENTATION_ITEM('')
);
#123=(
BOUNDED_CURVE()
B_SPLINE_CURVE(2,(#30482,#30483,#30484),.UNSPECIFIED.,.F.,.F.)
B_SPLINE_CURVE_WITH_KNOTS((3,3),(-2.29029703823246,-1.66304801526705),
 .UNSPECIFIED.)
CURVE()
GEOMETRIC_REPRESENTATION_ITEM()
RATIONAL_B_SPLINE_CURVE((1.40847966848734,1.4295768207167,1.40847966848733))
REPRESENTATION_ITEM('')
);
#124=(
BOUNDED_CURVE()
B_SPLINE_CURVE(2,(#30488,#30489,#30490),.UNSPECIFIED.,.F.,.F.)
B_SPLINE_CURVE_WITH_KNOTS((3,3),(-0.660669052461842,-0.35763920209058),
 .UNSPECIFIED.)
CURVE()
GEOMETRIC_REPRESENTATION_ITEM()
RATIONAL_B_SPLINE_CURVE((1.03886559867121,1.03696952671373,1.02863628649756))
REPRESENTATION_ITEM('')
);
#125=(
BOUNDED_CURVE()
B_SPLINE_CURVE(2,(#30508,#30509,#30510),.UNSPECIFIED.,.F.,.F.)
B_SPLINE_CURVE_WITH_KNOTS((3,3),(-1.14221416870064,-0.839184318329342),
 .UNSPECIFIED.)
CURVE()
GEOMETRIC_REPRESENTATION_ITEM()
RATIONAL_B_SPLINE_CURVE((1.0286362864976,1.03696952671377,1.03886559867125))
REPRESENTATION_ITEM('')
);
#126=(
BOUNDED_CURVE()
B_SPLINE_CURVE(2,(#30518,#30519,#30520),.UNSPECIFIED.,.F.,.F.)
B_SPLINE_CURVE_WITH_KNOTS((3,3),(-2.29029703823249,-1.97667252674982),
 .UNSPECIFIED.)
CURVE()
GEOMETRIC_REPRESENTATION_ITEM()
RATIONAL_B_SPLINE_CURVE((1.40847966848735,1.41902824460203,1.41902824460203))
REPRESENTATION_ITEM('')
);
#127=(
BOUNDED_CURVE()
B_SPLINE_CURVE(2,(#30521,#30522,#30523),.UNSPECIFIED.,.F.,.F.)
B_SPLINE_CURVE_WITH_KNOTS((3,3),(-1.97667252674982,-1.66304801526709),
 .UNSPECIFIED.)
CURVE()
GEOMETRIC_REPRESENTATION_ITEM()
RATIONAL_B_SPLINE_CURVE((1.41902824460203,1.41902824460203,1.40847966848735))
REPRESENTATION_ITEM('')
);
#128=(
BOUNDED_CURVE()
B_SPLINE_CURVE(2,(#30527,#30528,#30529),.UNSPECIFIED.,.F.,.F.)
B_SPLINE_CURVE_WITH_KNOTS((3,3),(-0.660669052460473,-0.357639202089695),
 .UNSPECIFIED.)
CURVE()
GEOMETRIC_REPRESENTATION_ITEM()
RATIONAL_B_SPLINE_CURVE((1.03886559866983,1.03696952671239,1.02863628649651))
REPRESENTATION_ITEM('')
);
#129=(
BOUNDED_CURVE()
B_SPLINE_CURVE(2,(#30852,#30853,#30854,#30855,#30856,#30857,#30858,#30859,
#30860),.UNSPECIFIED.,.F.,.F.)
B_SPLINE_CURVE_WITH_KNOTS((3,2,2,2,3),(0.,0.015625,0.03125,0.046875,0.0625),
 .UNSPECIFIED.)
CURVE()
GEOMETRIC_REPRESENTATION_ITEM()
RATIONAL_B_SPLINE_CURVE((1.,0.923879532511287,1.,0.923879532511287,1.,0.923879532511287,
1.,0.923879532511287,1.))
REPRESENTATION_ITEM('')
);
#130=(
BOUNDED_CURVE()
B_SPLINE_CURVE(2,(#30864,#30865,#30866,#30867,#30868,#30869,#30870,#30871,
#30872,#30873,#30874,#30875,#30876,#30877,#30878),.UNSPECIFIED.,.F.,.F.)
B_SPLINE_CURVE_WITH_KNOTS((3,2,2,2,2,2,2,3),(0.890625000369527,0.90625,
0.921875,0.9375,0.953125,0.96875,0.984375,1.),.UNSPECIFIED.)
CURVE()
GEOMETRIC_REPRESENTATION_ITEM()
RATIONAL_B_SPLINE_CURVE((0.999999996399544,0.923879534311515,1.,0.923879532511287,
1.,0.923879532511287,1.,0.923879532511287,1.,0.923879532511287,1.,0.923879532511287,
1.,0.923879532511287,1.))
REPRESENTATION_ITEM('')
);
#131=(
BOUNDED_CURVE()
B_SPLINE_CURVE(2,(#31184,#31185,#31186,#31187,#31188,#31189,#31190,#31191,
#31192),.UNSPECIFIED.,.F.,.F.)
B_SPLINE_CURVE_WITH_KNOTS((3,2,2,2,3),(0.,0.015625,0.03125,0.046875,0.0625),
 .UNSPECIFIED.)
CURVE()
GEOMETRIC_REPRESENTATION_ITEM()
RATIONAL_B_SPLINE_CURVE((1.,0.923879532511287,1.,0.923879532511287,1.,0.923879532511287,
1.,0.923879532511287,1.))
REPRESENTATION_ITEM('')
);
#132=(
BOUNDED_CURVE()
B_SPLINE_CURVE(2,(#32374,#32375,#32376,#32377,#32378,#32379,#32380,#32381,
#32382),.UNSPECIFIED.,.F.,.F.)
B_SPLINE_CURVE_WITH_KNOTS((3,2,2,2,3),(0.949015774239672,0.95,0.958333333333333,
0.966666666666667,0.975),.UNSPECIFIED.)
CURVE()
GEOMETRIC_REPRESENTATION_ITEM()
RATIONAL_B_SPLINE_CURVE((0.972090999933038,0.984176650141011,1.,0.866025403784439,
1.,0.866025403784439,1.,0.866025403784439,1.))
REPRESENTATION_ITEM('')
);
#133=(
BOUNDED_CURVE()
B_SPLINE_CURVE(2,(#32384,#32385,#32386,#32387,#32388,#32389,#32390,#32391,
#32392,#32393,#32394,#32395,#32396),.UNSPECIFIED.,.F.,.F.)
B_SPLINE_CURVE_WITH_KNOTS((3,2,2,2,2,2,3),(0.025,0.0333333333333333,0.0416666666666667,
0.05,0.0583333333333333,0.0666666666666667,0.075),.UNSPECIFIED.)
CURVE()
GEOMETRIC_REPRESENTATION_ITEM()
RATIONAL_B_SPLINE_CURVE((1.,0.866025403784439,1.,0.866025403784439,1.,0.866025403784439,
1.,0.866025403784439,1.,0.866025403784439,1.,0.866025403784439,1.))
REPRESENTATION_ITEM('')
);
#134=(
BOUNDED_CURVE()
B_SPLINE_CURVE(2,(#32398,#32399,#32400,#32401,#32402,#32403,#32404,#32405,
#32406,#32407,#32408,#32409,#32410),.UNSPECIFIED.,.F.,.F.)
B_SPLINE_CURVE_WITH_KNOTS((3,2,2,2,2,2,3),(0.025,0.0333333333333333,0.0416666666666667,
0.05,0.0583333333333333,0.0666666666666667,0.075),.UNSPECIFIED.)
CURVE()
GEOMETRIC_REPRESENTATION_ITEM()
RATIONAL_B_SPLINE_CURVE((1.,0.866025403784439,1.,0.866025403784439,1.,0.866025403784439,
1.,0.866025403784439,1.,0.866025403784439,1.,0.866025403784439,1.))
REPRESENTATION_ITEM('')
);
#135=(
BOUNDED_CURVE()
B_SPLINE_CURVE(2,(#32932,#32933,#32934,#32935,#32936,#32937,#32938,#32939,
#32940),.UNSPECIFIED.,.F.,.F.)
B_SPLINE_CURVE_WITH_KNOTS((3,2,2,2,3),(0.,0.00833333333333333,0.0166666666666666,
0.025,0.0286105917769561),.UNSPECIFIED.)
CURVE()
GEOMETRIC_REPRESENTATION_ITEM()
RATIONAL_B_SPLINE_CURVE((1.,0.866025403784439,1.,0.866025403784439,1.,0.866025403784439,
1.,0.941952690949969,0.934205814715252))
REPRESENTATION_ITEM('')
);
#184=CONICAL_SURFACE('',#18888,14.,0.908165646210649);
#185=CONICAL_SURFACE('',#19072,1.60000000000001,0.785398163397451);
#186=CONICAL_SURFACE('',#19074,2.,0.785398163397449);
#187=CONICAL_SURFACE('',#19076,3.99999999999999,0.785398163397452);
#188=CONICAL_SURFACE('',#19078,3.6,0.785398163397448);
#227=TOROIDAL_SURFACE('',#18885,9.1242968857267,4.22441061393973);
#228=TOROIDAL_SURFACE('',#18911,6.3,0.3);
#229=TOROIDAL_SURFACE('',#18913,9.7,0.3);
#286=B_SPLINE_CURVE_WITH_KNOTS('',3,(#27563,#27564,#27565,#27566,#27567,
#27568,#27569,#27570,#27571,#27572,#27573,#27574,#27575,#27576,#27577,#27578,
#27579,#27580),.UNSPECIFIED.,.F.,.F.,(4,2,2,2,2,2,2,2,4),(-0.43274489877026,
-0.430566610808932,-0.366750838333452,-0.304029800566765,-0.242875294955372,
-0.178422965186677,-0.116422491534204,-0.0594147705022417,-1.00000014308099E-6),
 .UNSPECIFIED.);
#287=B_SPLINE_CURVE_WITH_KNOTS('',3,(#27585,#27586,#27587,#27588,#27589,
#27590,#27591,#27592,#27593,#27594,#27595,#27596,#27597,#27598,#27599,#27600,
#27601,#27602,#27603,#27604,#27605,#27606,#27607,#27608,#27609,#27610,#27611,
#27612,#27613,#27614,#27615,#27616,#27617,#27618,#27619,#27620),
 .UNSPECIFIED.,.F.,.F.,(4,2,2,2,2,2,2,2,2,2,2,2,2,2,2,2,2,4),(-19.2450053801115,
-19.2031768304234,-19.1598456798386,-19.0949006094766,-19.0334251672637,
-18.9702316873635,-18.9060263489697,-18.8445259693451,-18.7806926247621,
-18.7178014261615,-18.6556018787519,-18.5909471802907,-18.5294501788449,
-18.4665257879972,-18.402418282567,-18.3411369020005,-18.2775557826221,
-18.2291330230763),.UNSPECIFIED.);
#288=B_SPLINE_CURVE_WITH_KNOTS('',3,(#27621,#27622,#27623,#27624,#27625,
#27626,#27627,#27628,#27629,#27630,#27631,#27632,#27633,#27634,#27635,#27636,
#27637,#27638,#27639,#27640,#27641,#27642,#27643,#27644,#27645,#27646,#27647,
#27648,#27649,#27650,#27651,#27652,#27653,#27654,#27655,#27656),
 .UNSPECIFIED.,.F.,.F.,(4,2,2,2,2,2,2,2,2,2,2,2,2,2,2,2,2,4),(-1.44203697926293,
-1.4313638992077,-1.36763608561743,-1.30534850184486,-1.24392281733326,
-1.17994358039373,-1.11838123753809,-1.05518319144789,-0.992043251713187,
-0.931149897187872,-0.867403341159369,-0.804924419349115,-0.743688850259094,
-0.679499044411844,-0.617742148113744,-0.554989179996601,-0.491622357088245,
-0.43274489877026),.UNSPECIFIED.);
#289=B_SPLINE_CURVE_WITH_KNOTS('',3,(#27661,#27662,#27663,#27664,#27665,
#27666,#27667,#27668,#27669,#27670,#27671,#27672,#27673,#27674,#27675,#27676,
#27677,#27678,#27679,#27680,#27681,#27682,#27683,#27684,#27685,#27686,#27687,
#27688,#27689,#27690,#27691,#27692,#27693,#27694,#27695,#27696),
 .UNSPECIFIED.,.F.,.F.,(4,2,2,2,2,2,2,2,2,2,2,2,2,2,2,2,2,4),(-18.2291330230763,
-18.2142764734255,-18.1522985596194,-18.0878831874444,-18.0262511910666,
-17.9635462256414,-17.8994836443016,-17.8383136315764,-17.7749377886959,
-17.7111621363704,-17.6493553372961,-17.5851256348085,-17.523253667619,
-17.460715475918,-17.3966486756835,-17.3354834665992,-17.2722627022774,
-17.2148871211445),.UNSPECIFIED.);
#290=B_SPLINE_CURVE_WITH_KNOTS('',3,(#27697,#27698,#27699,#27700,#27701,
#27702,#27703,#27704,#27705,#27706,#27707,#27708,#27709,#27710,#27711,#27712,
#27713,#27714,#27715,#27716,#27717,#27718,#27719,#27720,#27721,#27722,#27723,
#27724,#27725,#27726,#27727,#27728,#27729,#27730,#27731,#27732),
 .UNSPECIFIED.,.F.,.F.,(4,2,2,2,2,2,2,2,2,2,2,2,2,2,2,2,2,4),(-2.45150341078276,
-2.43286047511311,-2.36903133970015,-2.30696197397495,-2.24488499218074,
-2.18116000510695,-2.11982988395945,-2.05548507244458,-1.99265052578627,
-1.93176465691352,-1.86800840567019,-1.80585819717295,-1.74414477494485,
-1.6803213060518,-1.61890199565926,-1.55516382793806,-1.49220248568474,
-1.44203697926293),.UNSPECIFIED.);
#291=B_SPLINE_CURVE_WITH_KNOTS('',3,(#27737,#27738,#27739,#27740,#27741,
#27742,#27743,#27744,#27745,#27746,#27747,#27748,#27749,#27750,#27751,#27752,
#27753,#27754,#27755,#27756,#27757,#27758,#27759,#27760,#27761,#27762,#27763,
#27764,#27765,#27766,#27767,#27768,#27769,#27770,#27771,#27772,#27773,#27774),
 .UNSPECIFIED.,.F.,.F.,(4,2,2,2,2,2,2,2,2,2,2,2,2,2,2,2,2,2,4),(-17.2148871211445,
-17.2079083714811,-17.1462197339146,-17.0821193488849,-17.019918692549,
-16.9574916802273,-16.8933746296132,-16.8321170763526,-16.7689976469936,
-16.7048985425935,-16.6433013614118,-16.5793023952618,-16.5166170188716,
-16.4542691805168,-16.3894540991377,-16.3280048025785,-16.2649330315475,
-16.2007900611284,-16.1993047752053),.UNSPECIFIED.);
#292=B_SPLINE_CURVE_WITH_KNOTS('',3,(#27775,#27776,#27777,#27778,#27779,
#27780,#27781,#27782,#27783,#27784,#27785,#27786,#27787,#27788,#27789,#27790,
#27791,#27792,#27793,#27794,#27795,#27796,#27797,#27798,#27799,#27800,#27801,
#27802,#27803,#27804,#27805,#27806,#27807,#27808,#27809,#27810),
 .UNSPECIFIED.,.F.,.F.,(4,2,2,2,2,2,2,2,2,2,2,2,2,2,2,2,2,4),(-3.46293164573458,
-3.43582224646228,-3.37160540074597,-3.30981966037079,-3.24682737909425,
-3.18343959020337,-3.12235170905143,-3.05846173865086,-2.99572612090002,
-2.93445791446144,-2.86999522889465,-2.80798169069714,-2.74535920823371,
-2.68171365556681,-2.62045422247672,-2.5566456545727,-2.49388282097086,
-2.45150341078276),.UNSPECIFIED.);
#293=B_SPLINE_CURVE_WITH_KNOTS('',3,(#27815,#27816,#27817,#27818,#27819,
#27820,#27821,#27822,#27823,#27824,#27825,#27826,#27827,#27828,#27829,#27830,
#27831,#27832,#27833,#27834,#27835,#27836,#27837,#27838,#27839,#27840,#27841,
#27842,#27843,#27844,#27845,#27846,#27847,#27848,#27849,#27850),
 .UNSPECIFIED.,.F.,.F.,(4,2,2,2,2,2,2,2,2,2,2,2,2,2,2,2,2,4),(-16.1993047752053,
-16.139399623149,-16.0756819505149,-16.0126884662279,-15.9505936606462,
-15.8860511093153,-15.8245397396625,-15.7617197496252,-15.6976554447056,
-15.636446366356,-15.5729645605997,-15.5095423831343,-15.4476515691147,
-15.3833296291909,-15.3216449938471,-15.2590261184408,-15.1949889672839,
-15.1849810020995),.UNSPECIFIED.);
#294=B_SPLINE_CURVE_WITH_KNOTS('',3,(#27851,#27852,#27853,#27854,#27855,
#27856,#27857,#27858,#27859,#27860,#27861,#27862,#27863,#27864,#27865,#27866,
#27867,#27868,#27869,#27870,#27871,#27872,#27873,#27874,#27875,#27876,#27877,
#27878,#27879,#27880,#27881,#27882,#27883,#27884,#27885,#27886),
 .UNSPECIFIED.,.F.,.F.,(4,2,2,2,2,2,2,2,2,2,2,2,2,2,2,2,2,4),(-4.47360893918925,
-4.43794954459914,-4.37406242834937,-4.31257984542803,-4.24854010296684,
-4.18552550866014,-4.12458339993076,-4.06074796570392,-3.99841199290557,
-3.93680004026492,-3.87277595257713,-3.81116800361354,-3.74769502592802,
-3.68451859179219,-3.62355703375697,-3.55971906533952,-3.49720928424716,
-3.46293164573458),.UNSPECIFIED.);
#295=B_SPLINE_CURVE_WITH_KNOTS('',3,(#27891,#27892,#27893,#27894,#27895,
#27896,#27897,#27898,#27899,#27900,#27901,#27902,#27903,#27904,#27905,#27906,
#27907,#27908,#27909,#27910,#27911,#27912,#27913,#27914,#27915,#27916,#27917,
#27918,#27919,#27920,#27921,#27922,#27923,#27924,#27925,#27926),
 .UNSPECIFIED.,.F.,.F.,(4,2,2,2,2,2,2,2,2,2,2,2,2,2,2,2,2,4),(-15.1849810020995,
-15.1338530100102,-15.070559094631,-15.0066083905476,-14.9448702116096,
-14.880714276949,-14.8187558459082,-14.7562843671171,-14.6922264280455,
-14.6310595201955,-14.5679020497222,-14.5033508992441,-14.4417116096791,
-14.3776644891707,-14.3153519312524,-14.2529714041824,-14.1888475931021,
-14.1707416963743),.UNSPECIFIED.);
#296=B_SPLINE_CURVE_WITH_KNOTS('',3,(#27927,#27928,#27929,#27930,#27931,
#27932,#27933,#27934,#27935,#27936,#27937,#27938,#27939,#27940,#27941,#27942,
#27943,#27944,#27945,#27946,#27947,#27948,#27949,#27950,#27951,#27952,#27953,
#27954,#27955,#27956,#27957,#27958,#27959,#27960,#27961,#27962),
 .UNSPECIFIED.,.F.,.F.,(4,2,2,2,2,2,2,2,2,2,2,2,2,2,2,2,2,4),(-5.48535228916885,
-5.44066073025292,-5.37716695179706,-5.31599374200483,-5.25209855020388,
-5.18924548417807,-5.12804829157604,-5.06345594395374,-5.00132373767058,
-4.93893004537637,-4.87514967405474,-4.81376360203583,-4.74990140251206,
-4.68699557761332,-4.62597435119929,-4.5620951884975,-4.49987800983087,
-4.47360893918925),.UNSPECIFIED.);
#297=B_SPLINE_CURVE_WITH_KNOTS('',3,(#27967,#27968,#27969,#27970,#27971,
#27972,#27973,#27974,#27975,#27976,#27977,#27978,#27979,#27980,#27981,#27982,
#27983,#27984,#27985,#27986,#27987,#27988,#27989,#27990,#27991,#27992,#27993,
#27994,#27995,#27996,#27997,#27998,#27999,#28000,#28001,#28002),
 .UNSPECIFIED.,.F.,.F.,(4,2,2,2,2,2,2,2,2,2,2,2,2,2,2,2,2,4),(-14.1707416963743,
-14.1275575364455,-14.0644816493245,-14.0003777496193,-13.9388161694758,
-13.8748559310113,-13.8120154097725,-13.7496985264462,-13.6849190009467,
-13.6233996931089,-13.5603578496633,-13.4961841329855,-13.4348074482046,
-13.3711132207576,-13.3079206564436,-13.2458402648998,-13.1813158002758,
-13.154780839114),.UNSPECIFIED.);
#298=B_SPLINE_CURVE_WITH_KNOTS('',3,(#28003,#28004,#28005,#28006,#28007,
#28008,#28009,#28010,#28011,#28012,#28013,#28014,#28015,#28016,#28017,#28018,
#28019,#28020,#28021,#28022,#28023,#28024,#28025,#28026,#28027,#28028,#28029,
#28030,#28031,#28032,#28033,#28034,#28035,#28036,#28037,#28038),
 .UNSPECIFIED.,.F.,.F.,(4,2,2,2,2,2,2,2,2,2,2,2,2,2,2,2,2,4),(-6.49539175200228,
-6.44175461758173,-6.37869675301284,-6.31780818618473,-6.25403343173878,
-6.19164606426418,-6.13024672738864,-6.06616052832269,-6.00449767885634,
-5.94140530906691,-5.87815315446652,-5.81717609779043,-5.75336705637975,
-5.69077185590904,-5.62952948385544,-5.56521587780421,-5.50334261762044,
-5.48535228916885),.UNSPECIFIED.);
#299=B_SPLINE_CURVE_WITH_KNOTS('',3,(#28043,#28044,#28045,#28046,#28047,
#28048,#28049,#28050,#28051,#28052,#28053,#28054,#28055,#28056,#28057,#28058,
#28059,#28060,#28061,#28062,#28063,#28064,#28065,#28066,#28067,#28068,#28069,
#28070,#28071,#28072,#28073,#28074,#28075,#28076,#28077,#28078),
 .UNSPECIFIED.,.F.,.F.,(4,2,2,2,2,2,2,2,2,2,2,2,2,2,2,2,2,4),(-13.154780839114,
-13.1196948938244,-13.0568878202012,-12.9927745160496,-12.9315418600343,
-12.868067425228,-12.8044082571734,-12.7425145031164,-12.6781922176648,
-12.6163617176352,-12.5537376505848,-12.4896345068317,-12.4284379893464,
-12.3651341760799,-12.3009175828982,-12.2391582045385,-12.1749824942442,
-12.1398252878704),.UNSPECIFIED.);
#300=B_SPLINE_CURVE_WITH_KNOTS('',3,(#28079,#28080,#28081,#28082,#28083,
#28084,#28085,#28086,#28087,#28088,#28089,#28090,#28091,#28092,#28093,#28094,
#28095,#28096,#28097,#28098,#28099,#28100,#28101,#28102,#28103,#28104,#28105,
#28106,#28107,#28108,#28109,#28110,#28111,#28112,#28113,#28114),
 .UNSPECIFIED.,.F.,.F.,(4,2,2,2,2,2,2,2,2,2,2,2,2,2,2,2,2,4),(-7.50558706522749,
-7.4434856273175,-7.38066073607584,-7.31964567117951,-7.25579777663904,
-7.19366409555753,-7.13166323964892,-7.06786727378737,-7.00647046448262,
-6.94227522225779,-6.87936093702994,-6.81845608236433,-6.75466739446041,
-6.69243480618895,-6.63077645718591,-6.56686368184471,-6.50536045230073,
-6.49539175200228),.UNSPECIFIED.);
#301=B_SPLINE_CURVE_WITH_KNOTS('',3,(#28119,#28120,#28121,#28122,#28123,
#28124,#28125,#28126,#28127,#28128,#28129,#28130,#28131,#28132,#28133,#28134,
#28135,#28136,#28137,#28138,#28139,#28140,#28141,#28142,#28143,#28144,#28145,
#28146,#28147,#28148,#28149,#28150,#28151,#28152,#28153,#28154),
 .UNSPECIFIED.,.F.,.F.,(4,2,2,2,2,2,2,2,2,2,2,2,2,2,2,2,2,4),(-12.1398252878704,
-12.1128469838547,-12.0503511223232,-11.9862112217519,-11.9249500379598,
-11.861764103918,-11.7976401351988,-11.73598361746,-11.6719213824629,-11.6093387981136,
-11.5469349800063,-11.4820586087665,-11.4206376040574,-11.3575104256224,
-11.2933655333597,-11.2292834427868,-11.1662639105294,-11.1240342053348),
 .UNSPECIFIED.);
#302=B_SPLINE_CURVE_WITH_KNOTS('',3,(#28155,#28156,#28157,#28158,#28159,
#28160,#28161,#28162,#28163,#28164,#28165,#28166,#28167,#28168,#28169,#28170,
#28171,#28172,#28173,#28174,#28175,#28176,#28177,#28178,#28179,#28180,#28181,
#28182,#28183,#28184,#28185,#28186,#28187,#28188,#28189,#28190,#28191,#28192),
 .UNSPECIFIED.,.F.,.F.,(4,2,2,2,2,2,2,2,2,2,2,2,2,2,2,2,2,2,4),(-8.51705611258781,
-8.51047438623768,-8.44665403963334,-8.38410939297357,-8.32279614319828,
-8.25853933422636,-8.19671765139568,-8.13387567283019,-8.07044331417221,
-8.00932342898535,-7.94543561802143,-7.88265029342846,-7.82142233119061,
-7.75690445982659,-7.69484058642041,-7.63233160620855,-7.56862817681911,
-7.5073144426173,-7.50558706522749),.UNSPECIFIED.);
#303=B_SPLINE_CURVE_WITH_KNOTS('',3,(#28197,#28198,#28199,#28200,#28201,
#28202,#28203,#28204,#28205,#28206,#28207,#28208,#28209,#28210,#28211,#28212,
#28213,#28214,#28215,#28216,#28217,#28218,#28219,#28220,#28221,#28222,#28223,
#28224,#28225,#28226,#28227,#28228,#28229,#28230,#28231,#28232),
 .UNSPECIFIED.,.F.,.F.,(4,2,2,2,2,2,2,2,2,2,2,2,2,2,2,2,2,4),(-11.1240342053348,
-11.1049715007544,-11.0408683970359,-10.9785460178958,-10.9161742311307,
-10.85219096625,-10.7906118138308,-10.7259407224929,-10.6628544690203,-10.6017066275169,
-10.5376807557104,-10.4752825869107,-10.4132817799571,-10.3492050927119,
-10.2875415246768,-10.2234842795807,-10.1602757416615,-10.1102965696432),
 .UNSPECIFIED.);
#304=B_SPLINE_CURVE_WITH_KNOTS('',3,(#28233,#28234,#28235,#28236,#28237,
#28238,#28239,#28240,#28241,#28242,#28243,#28244,#28245,#28246,#28247,#28248,
#28249,#28250,#28251,#28252,#28253,#28254,#28255,#28256,#28257,#28258,#28259,
#28260,#28261,#28262,#28263,#28264,#28265,#28266,#28267,#28268),
 .UNSPECIFIED.,.F.,.F.,(4,2,2,2,2,2,2,2,2,2,2,2,2,2,2,2,2,4),(-9.52725242033231,
-9.51228710180808,-9.44845348442619,-9.38623386265022,-9.32443494998258,
-9.26054076930463,-9.19905317665517,-9.13521773232532,-9.07218767679157,
-9.01127714224445,-8.94747372038282,-8.88511865511398,-8.82361115858219,
-8.75956314764917,-8.6979343471348,-8.63464271854794,-8.57143574519437,
-8.51705611258781),.UNSPECIFIED.);
#305=B_SPLINE_CURVE_WITH_KNOTS('',3,(#28273,#28274,#28275,#28276,#28277,
#28278,#28279,#28280,#28281,#28282,#28283,#28284,#28285,#28286,#28287,#28288,
#28289,#28290,#28291,#28292,#28293,#28294,#28295,#28296,#28297,#28298,#28299,
#28300,#28301,#28302,#28303,#28304,#28305,#28306,#28307,#28308),
 .UNSPECIFIED.,.F.,.F.,(4,2,2,2,2,2,2,2,2,2,2,2,2,2,2,2,2,4),(-10.1102965696432,
-10.0991843775796,-10.0351913345793,-9.97266042570376,-9.91095678307518,
-9.84672895535158,-9.78492671650828,-9.72141934320778,-9.6580361697458,
-9.59689974457259,-9.53289243950799,-9.47017432877619,-9.40867125058455,
-9.3442370011338,-9.28224412700868,-9.21919366214322,-9.15558705531007,
-9.09687640456266),.UNSPECIFIED.);
#306=B_SPLINE_CURVE_WITH_KNOTS('',3,(#28309,#28310,#28311,#28312,#28313,
#28314,#28315,#28316,#28317,#28318,#28319,#28320,#28321,#28322,#28323,#28324,
#28325,#28326,#28327,#28328,#28329,#28330,#28331,#28332,#28333,#28334,#28335,
#28336,#28337,#28338,#28339,#28340,#28341,#28342,#28343,#28344),
 .UNSPECIFIED.,.F.,.F.,(4,2,2,2,2,2,2,2,2,2,2,2,2,2,2,2,2,4),(-10.5381172670408,
-10.512455978803,-10.4503254341735,-10.386510740348,-10.3255411450287,-10.2627213346113,
-10.1989245869234,-10.1376195399027,-10.0739241689982,-10.0115286955865,
-9.94947636117586,-9.88735421108905,-9.82512831769023,-9.76135256505236,
-9.69997254252333,-9.63615374965774,-9.57324861389179,-9.52725242033231),
 .UNSPECIFIED.);
#307=B_SPLINE_CURVE_WITH_KNOTS('',3,(#28349,#28350,#28351,#28352,#28353,
#28354,#28355,#28356,#28357,#28358,#28359,#28360,#28361,#28362,#28363,#28364,
#28365,#28366,#28367,#28368,#28369,#28370,#28371,#28372,#28373,#28374,#28375,
#28376,#28377,#28378,#28379,#28380,#28381,#28382,#28383,#28384,#28385,#28386),
 .UNSPECIFIED.,.F.,.F.,(4,2,2,2,2,2,2,2,2,2,2,2,2,2,2,2,2,2,4),(-9.09687640456266,
-9.09429765138321,-9.0302256031248,-8.96726887397095,-8.9058576390194,-8.84116440171671,
-8.77893131411787,-8.71622177873111,-8.65234579423566,-8.59086571160834,
-8.52685699401383,-8.46386280799012,-8.40267113289702,-8.33864297752146,
-8.27634241271939,-8.2141493879631,-8.15018297227031,-8.08862181773403,
-8.08262706977625),.UNSPECIFIED.);
#308=B_SPLINE_CURVE_WITH_KNOTS('',3,(#28387,#28388,#28389,#28390,#28391,
#28392,#28393,#28394,#28395,#28396,#28397,#28398,#28399,#28400,#28401,#28402,
#28403,#28404,#28405,#28406,#28407,#28408,#28409,#28410,#28411,#28412,#28413,
#28414,#28415,#28416,#28417,#28418,#28419,#28420,#28421,#28422),
 .UNSPECIFIED.,.F.,.F.,(4,2,2,2,2,2,2,2,2,2,2,2,2,2,2,2,2,4),(-11.5476264878665,
-11.5140365460968,-11.4516308740854,-11.3878716449922,-11.3269918026019,
-11.2639182524274,-11.2004369463522,-11.1389245305944,-11.07500084939,-11.013417671742,
-10.9511772470223,-10.8874131737632,-10.8265367108085,-10.7636167982201,
-10.6995586349995,-10.6381630855281,-10.5743673266148,-10.5381172670408),
 .UNSPECIFIED.);
#309=B_SPLINE_CURVE_WITH_KNOTS('',3,(#28427,#28428,#28429,#28430,#28431,
#28432,#28433,#28434,#28435,#28436,#28437,#28438,#28439,#28440,#28441,#28442,
#28443,#28444,#28445,#28446,#28447,#28448,#28449,#28450,#28451,#28452,#28453,
#28454,#28455,#28456,#28457,#28458,#28459,#28460,#28461,#28462),
 .UNSPECIFIED.,.F.,.F.,(4,2,2,2,2,2,2,2,2,2,2,2,2,2,2,2,2,4),(-8.08262706977625,
-8.02421455182451,-7.96113392805235,-7.90005770458101,-7.83609144286503,
-7.77369497498638,-7.71184945932058,-7.64776923316301,-7.58610448703455,
-7.52229170167221,-7.45907012529655,-7.39801598821222,-7.33406637134758,
-7.27151783754628,-7.20993747384233,-7.14568653069794,-7.08386471745399,
-7.07010568792935),.UNSPECIFIED.);
#310=B_SPLINE_CURVE_WITH_KNOTS('',3,(#28463,#28464,#28465,#28466,#28467,
#28468,#28469,#28470,#28471,#28472,#28473,#28474,#28475,#28476,#28477,#28478,
#28479,#28480,#28481,#28482,#28483,#28484,#28485,#28486,#28487,#28488,#28489,
#28490,#28491,#28492,#28493,#28494,#28495,#28496,#28497,#28498),
 .UNSPECIFIED.,.F.,.F.,(4,2,2,2,2,2,2,2,2,2,2,2,2,2,2,2,2,4),(-12.5583011318705,
-12.5164244272338,-12.453533904535,-12.3896340325225,-12.3284282946859,
-12.2649006882095,-12.202302571561,-12.1404006409781,-12.0760554349159,
-12.0148482976973,-11.9522249338035,-11.8884216857418,-11.8274324792701,
-11.7641552830532,-11.701169280429,-11.6394872633689,-11.5753795396612,
-11.5476264878665),.UNSPECIFIED.);
#311=B_SPLINE_CURVE_WITH_KNOTS('',3,(#28503,#28504,#28505,#28506,#28507,
#28508,#28509,#28510,#28511,#28512,#28513,#28514,#28515,#28516,#28517,#28518,
#28519,#28520,#28521,#28522,#28523,#28524,#28525,#28526,#28527,#28528,#28529,
#28530,#28531,#28532,#28533,#28534,#28535,#28536,#28537,#28538),
 .UNSPECIFIED.,.F.,.F.,(4,2,2,2,2,2,2,2,2,2,2,2,2,2,2,2,2,4),(-7.07010568792935,
-7.02057195526808,-6.95715837040495,-6.89602168015075,-6.83204054447954,
-6.76928656991371,-6.7078697716623,-6.64339382293125,-6.58136387292713,
-6.51848925069081,-6.45483602060775,-6.3935087439113,-6.32944430613884,
-6.26643455412798,-6.20506961813476,-6.14031704292197,-6.07803016863274,
-6.05626210410768),.UNSPECIFIED.);
#312=B_SPLINE_CURVE_WITH_KNOTS('',3,(#28539,#28540,#28541,#28542,#28543,
#28544,#28545,#28546,#28547,#28548,#28549,#28550,#28551,#28552,#28553,#28554,
#28555,#28556,#28557,#28558,#28559,#28560,#28561,#28562,#28563,#28564,#28565,
#28566,#28567,#28568,#28569,#28570,#28571,#28572,#28573,#28574),
 .UNSPECIFIED.,.F.,.F.,(4,2,2,2,2,2,2,2,2,2,2,2,2,2,2,2,2,4),(-13.5700232395142,
-13.5204005870663,-13.4573318747156,-13.3933719339399,-13.3318427510029,
-13.2679060883571,-13.2060132812835,-13.1437505760427,-13.0798539406011,
-13.0188264204508,-12.9558764789665,-12.8919955376263,-12.8305697425558,
-12.766747094191,-12.7044120458901,-12.6422420703319,-12.5776085442114,
-12.5583011318705),.UNSPECIFIED.);
#313=B_SPLINE_CURVE_WITH_KNOTS('',3,(#28579,#28580,#28581,#28582,#28583,
#28584,#28585,#28586,#28587,#28588,#28589,#28590,#28591,#28592,#28593,#28594,
#28595,#28596,#28597,#28598,#28599,#28600,#28601,#28602,#28603,#28604,#28605,
#28606,#28607,#28608,#28609,#28610,#28611,#28612,#28613,#28614),
 .UNSPECIFIED.,.F.,.F.,(4,2,2,2,2,2,2,2,2,2,2,2,2,2,2,2,2,4),(-6.05626210410768,
-6.0154519013265,-5.9515138295235,-5.88997569337269,-5.82594853894846,-5.7628879405073,
-5.70170531265335,-5.63766078512489,-5.57529108892424,-5.51318619075399,
-5.44914331646863,-5.38751051846565,-5.32327540580219,-5.26010879987577,
-5.19901056374118,-5.13501235853817,-5.07252669067762,-5.04250930940443),
 .UNSPECIFIED.);
#314=B_SPLINE_CURVE_WITH_KNOTS('',3,(#28615,#28616,#28617,#28618,#28619,
#28620,#28621,#28622,#28623,#28624,#28625,#28626,#28627,#28628,#28629,#28630,
#28631,#28632,#28633,#28634,#28635,#28636,#28637,#28638,#28639,#28640,#28641,
#28642,#28643,#28644,#28645,#28646,#28647,#28648,#28649,#28650),
 .UNSPECIFIED.,.F.,.F.,(4,2,2,2,2,2,2,2,2,2,2,2,2,2,2,2,2,4),(-14.5813080464973,
-14.5229842167791,-14.459524148473,-14.3965799254724,-14.3347283766724,
-14.2704415484857,-14.2090567993869,-14.1464813701105,-14.0826089233366,
-14.0216048982894,-13.9583649586076,-13.8949584508584,-13.8332940872334,
-13.769210006081,-13.7076189535549,-13.6452271481187,-13.5813660136001,
-13.5700232395142),.UNSPECIFIED.);
#315=B_SPLINE_CURVE_WITH_KNOTS('',3,(#28655,#28656,#28657,#28658,#28659,
#28660,#28661,#28662,#28663,#28664,#28665,#28666,#28667,#28668,#28669,#28670,
#28671,#28672,#28673,#28674,#28675,#28676,#28677,#28678,#28679,#28680,#28681,
#28682,#28683,#28684,#28685,#28686,#28687,#28688,#28689,#28690),
 .UNSPECIFIED.,.F.,.F.,(4,2,2,2,2,2,2,2,2,2,2,2,2,2,2,2,2,4),(-5.04250930940443,
-5.01074345740576,-4.94656642853249,-4.88481091988587,-4.82114792736413,
-4.75782191979311,-4.69670993316011,-4.63271182641902,-4.57005488216266,
-4.50850272047019,-4.4441354654514,-4.38220455481827,-4.31902895774606,
-4.25549371142046,-4.19426107834615,-4.13021367387332,-4.06733312302916,
-4.02900754571855),.UNSPECIFIED.);
#316=B_SPLINE_CURVE_WITH_KNOTS('',3,(#28691,#28692,#28693,#28694,#28695,
#28696,#28697,#28698,#28699,#28700,#28701,#28702,#28703,#28704,#28705,#28706,
#28707,#28708,#28709,#28710,#28711,#28712,#28713,#28714,#28715,#28716,#28717,
#28718,#28719,#28720,#28721,#28722,#28723,#28724,#28725,#28726,#28727,#28728),
 .UNSPECIFIED.,.F.,.F.,(4,2,2,2,2,2,2,2,2,2,2,2,2,2,2,2,2,2,4),(-15.5933221971989,
-15.5875677904679,-15.5261531677509,-15.4623393509046,-15.400265719406,
-15.3381128208409,-15.2742269043841,-15.2131662822886,-15.1503208065578,
-15.0864546018284,-15.0251184153014,-14.9613922317184,-14.8987956903211,
-14.8367073456883,-14.7721651536426,-14.7108788500126,-14.6480683038418,
-14.5841343915024,-14.5813080464973),.UNSPECIFIED.);
#317=B_SPLINE_CURVE_WITH_KNOTS('',3,(#28733,#28734,#28735,#28736,#28737,
#28738,#28739,#28740,#28741,#28742,#28743,#28744,#28745,#28746,#28747,#28748,
#28749,#28750,#28751,#28752,#28753,#28754,#28755,#28756,#28757,#28758,#28759,
#28760,#28761,#28762,#28763,#28764,#28765,#28766,#28767,#28768),
 .UNSPECIFIED.,.F.,.F.,(4,2,2,2,2,2,2,2,2,2,2,2,2,2,2,2,2,4),(-4.02900754571855,
-4.0059062389982,-3.94129539215301,-3.87913881741449,-3.81634060720317,
-3.75254945348995,-3.69114962308604,-3.62718800769495,-3.56428259058608,
-3.50310844301288,-3.43912597478557,-3.37691614892503,-3.31467179696546,
-3.25080355834965,-3.18933527194429,-3.12480362707408,-3.06182973481643,
-3.01586943876209),.UNSPECIFIED.);
#318=B_SPLINE_CURVE_WITH_KNOTS('',3,(#28769,#28770,#28771,#28772,#28773,
#28774,#28775,#28776,#28777,#28778,#28779,#28780,#28781,#28782,#28783,#28784,
#28785,#28786,#28787,#28788,#28789,#28790,#28791,#28792,#28793,#28794,#28795,
#28796,#28797,#28798,#28799,#28800,#28801,#28802,#28803,#28804),
 .UNSPECIFIED.,.F.,.F.,(4,2,2,2,2,2,2,2,2,2,2,2,2,2,2,2,2,4),(-16.6035198604699,
-16.5900454824747,-16.52837749622,-16.4642869299382,-16.4028347554628,-16.3404414845704,
-16.2766395839102,-16.2157277579415,-16.152662237515,-16.0889611903744,
-16.0274466316654,-15.9635229009172,-15.9018003282277,-15.8395553329516,
-15.7757339163795,-15.71479381237,-15.6518656052688,-15.5933221971989),
 .UNSPECIFIED.);
#319=B_SPLINE_CURVE_WITH_KNOTS('',3,(#28809,#28810,#28811,#28812,#28813,
#28814,#28815,#28816,#28817,#28818,#28819,#28820,#28821,#28822,#28823,#28824,
#28825,#28826,#28827,#28828,#28829,#28830,#28831,#28832,#28833,#28834,#28835,
#28836,#28837,#28838,#28839,#28840,#28841,#28842,#28843,#28844),
 .UNSPECIFIED.,.F.,.F.,(4,2,2,2,2,2,2,2,2,2,2,2,2,2,2,2,2,4),(-3.01586943876209,
-3.00079724181661,-2.93689043293634,-2.8746030456085,-2.81272692241491,
-2.74876349342228,-2.68720912181028,-2.62328856932311,-2.56019082819264,
-2.49921153393853,-2.43533598225039,-2.37291425081546,-2.31133185138697,
-2.24721568730844,-2.18552114055543,-2.12214682151061,-2.05887309443656,
-2.00453087624746),.UNSPECIFIED.);
#320=B_SPLINE_CURVE_WITH_KNOTS('',3,(#28845,#28846,#28847,#28848,#28849,
#28850,#28851,#28852,#28853,#28854,#28855,#28856,#28857,#28858,#28859,#28860,
#28861,#28862,#28863,#28864,#28865,#28866,#28867,#28868,#28869,#28870,#28871,
#28872,#28873,#28874,#28875,#28876,#28877,#28878,#28879,#28880),
 .UNSPECIFIED.,.F.,.F.,(4,2,2,2,2,2,2,2,2,2,2,2,2,2,2,2,2,4),(-17.614935493873,
-17.5934598904259,-17.53133403337,-17.4667494645793,-17.4055260732277,-17.3426789621963,
-17.2787689742008,-17.2175980676138,-17.1541078739038,-17.0913554027581,
-17.0294828842969,-16.9651711475964,-16.9038888570392,-16.8412938681442,
-16.7774636347221,-16.7164761842175,-16.653222186963,-16.6035198604699),
 .UNSPECIFIED.);
#321=B_SPLINE_CURVE_WITH_KNOTS('',3,(#28886,#28887,#28888,#28889,#28890,
#28891,#28892,#28893,#28894,#28895,#28896,#28897,#28898,#28899,#28900,#28901,
#28902,#28903,#28904,#28905,#28906,#28907,#28908,#28909,#28910,#28911,#28912,
#28913,#28914,#28915,#28916,#28917),.UNSPECIFIED.,.F.,.F.,(4,2,2,2,2,2,
2,2,2,2,2,2,2,2,2,4),(-19.4936808899958,-19.4531550473275,-19.4114253894815,
-19.3480658590082,-19.2850241322855,-19.2232628932131,-19.159072502976,
-19.0976657032011,-19.0351800920759,-18.9713461232385,-18.910393411917,
-18.8472396492887,-18.7837058034619,-18.7221163760458,-18.6581123837969,
-18.6261649225256),.UNSPECIFIED.);
#322=B_SPLINE_CURVE_WITH_KNOTS('',3,(#28920,#28921,#28922,#28923,#28924,
#28925,#28926,#28927,#28928,#28929,#28930,#28931,#28932,#28933,#28934,#28935,
#28936,#28937,#28938,#28939,#28940,#28941,#28942,#28943,#28944,#28945,#28946,
#28947,#28948,#28949,#28950,#28951,#28952,#28953),.UNSPECIFIED.,.F.,.F.,
(4,2,2,2,2,2,2,2,2,2,2,2,2,2,2,2,4),(-0.991954268502835,-0.92969776175528,
-0.866808936262966,-0.805726881798867,-0.741810702793368,-0.679614012179091,
-0.617539964427152,-0.553679664627321,-0.49222081736718,-0.427944533954764,
-0.364967508943842,-0.303997772933001,-0.240141878760337,-0.177847495603767,
-0.116117953761281,-0.0578271827732781,-9.99999998252399E-7),
 .UNSPECIFIED.);
#323=B_SPLINE_CURVE_WITH_KNOTS('',3,(#29557,#29558,#29559,#29560,#29561,
#29562,#29563,#29564,#29565,#29566,#29567,#29568,#29569,#29570,#29571,#29572,
#29573,#29574,#29575,#29576,#29577,#29578,#29579,#29580,#29581,#29582,#29583,
#29584,#29585,#29586,#29587,#29588),.UNSPECIFIED.,.F.,.F.,(4,2,2,2,2,2,
2,2,2,2,2,2,2,2,2,4),(1.0000000159313E-6,0.184001326101672,0.37041664464277,
0.703290139702188,1.03440506548376,1.36773974881136,1.69865455171767,2.03244840671975,
2.36317397254373,2.6974230132541,3.02797037146041,3.3626688271678,3.69304907229932,
4.02818958292247,4.35841380142651,4.64135684187533),.UNSPECIFIED.);
#324=B_SPLINE_CURVE_WITH_KNOTS('',3,(#29591,#29592,#29593,#29594,#29595,
#29596,#29597,#29598,#29599,#29600,#29601,#29602,#29603,#29604,#29605,#29606,
#29607,#29608,#29609,#29610,#29611,#29612,#29613,#29614,#29615,#29616,#29617,
#29618),.UNSPECIFIED.,.F.,.F.,(4,2,2,2,2,2,2,2,2,2,2,2,2,4),(14.0669063991451,
14.1284264825117,14.4671173829221,14.7937484791654,15.1326547393244,15.4593625495219,
15.7984769197192,16.1252697919598,16.4645851145556,16.7914700330379,17.1309792827163,
17.4579619797361,17.7485763441689,18.0394413523531),.UNSPECIFIED.);
#325=B_SPLINE_CURVE_WITH_KNOTS('',3,(#29623,#29624,#29625,#29626,#29627,
#29628,#29629,#29630,#29631,#29632,#29633,#29634,#29635,#29636,#29637,#29638,
#29639,#29640,#29641,#29642,#29643,#29644,#29645,#29646,#29647,#29648,#29649,
#29650,#29651,#29652,#29653,#29654,#29655,#29656,#29657,#29658),
 .UNSPECIFIED.,.F.,.F.,(4,2,2,2,2,2,2,2,2,2,2,2,2,2,2,2,2,4),(4.64135684187533,
4.69398762946712,5.02406690378143,5.36006416228109,5.6900092970561,6.0264189975231,
6.35624067954145,6.69305109308465,7.02275977360977,7.35995854918521,7.68956440436171,
8.02713873558435,8.35665163351959,8.69458841162062,9.02401788581675,9.35169718603101,
9.69247573073726,10.0050542561348),.UNSPECIFIED.);
#326=B_SPLINE_CURVE_WITH_KNOTS('',3,(#29659,#29660,#29661,#29662,#29663,
#29664,#29665,#29666,#29667,#29668,#29669,#29670,#29671,#29672,#29673,#29674,
#29675,#29676,#29677,#29678,#29679,#29680,#29681,#29682,#29683,#29684,#29685,
#29686,#29687,#29688,#29689,#29690,#29691,#29692,#29693,#29694),
 .UNSPECIFIED.,.F.,.F.,(4,2,2,2,2,2,2,2,2,2,2,2,2,2,2,2,2,4),(8.70719789233371,
8.81570165061824,9.1524157175717,9.47892443720727,9.81590840352668,10.1423689843966,
10.4796170049242,10.8060509235,11.1435567243114,11.4699838356931,11.8077407934984,
12.1341792602608,12.4721804795241,12.7986467381769,13.1368851247795,13.4633938864294,
13.8018622169238,14.0669063991451),.UNSPECIFIED.);
#327=B_SPLINE_CURVE_WITH_KNOTS('',3,(#29699,#29700,#29701,#29702,#29703,
#29704,#29705,#29706,#29707,#29708,#29709,#29710,#29711,#29712,#29713,#29714,
#29715,#29716,#29717,#29718,#29719,#29720,#29721,#29722,#29723,#29724,#29725,
#29726,#29727,#29728,#29729,#29730,#29731,#29732,#29733,#29734),
 .UNSPECIFIED.,.F.,.F.,(4,2,2,2,2,2,2,2,2,2,2,2,2,2,2,2,2,4),(10.0050542561348,
10.0202666236202,10.361182715358,10.6890843397369,11.0301335185425,11.358144772174,
11.6993228356638,12.0274424289947,12.3687454254136,12.696971928326,13.0383961484681,
13.3667280305269,13.7082699987937,14.0367056635557,14.3783621283825,14.7068999423348,
15.0486678661882,15.3747761103741),.UNSPECIFIED.);
#328=B_SPLINE_CURVE_WITH_KNOTS('',3,(#29735,#29736,#29737,#29738,#29739,
#29740,#29741,#29742,#29743,#29744,#29745,#29746,#29747,#29748,#29749,#29750,
#29751,#29752,#29753,#29754,#29755,#29756,#29757,#29758,#29759,#29760,#29761,
#29762,#29763,#29764,#29765,#29766,#29767,#29768,#29769,#29770),
 .UNSPECIFIED.,.F.,.F.,(4,2,2,2,2,2,2,2,2,2,2,2,2,2,2,2,2,4),(3.34852080740999,
3.51541382366282,3.84983510106026,4.1776416565033,4.51235510680904,4.83990488875393,
5.17491070933339,5.50223095942833,5.83752839411276,6.16464663854683,6.50023401625068,
6.82717773172898,7.16305251610975,7.48984881036069,7.82600765901454,8.15268297405058,
8.48912180554802,8.70719789233371),.UNSPECIFIED.);
#329=B_SPLINE_CURVE_WITH_KNOTS('',3,(#30067,#30068,#30069,#30070,#30071,
#30072,#30073,#30074,#30075,#30076),.UNSPECIFIED.,.F.,.F.,(4,2,2,2,4),(-1.08763065698974,
-0.805155960498027,-0.481178691573332,-0.239177070179376,-1.00000002545286E-6),
 .UNSPECIFIED.);
#330=B_SPLINE_CURVE_WITH_KNOTS('',3,(#30079,#30080,#30081,#30082,#30083,
#30084,#30085,#30086,#30087,#30088,#30089,#30090,#30091,#30092,#30093,#30094,
#30095,#30096,#30097,#30098,#30099,#30100,#30101,#30102,#30103,#30104,#30105,
#30106,#30107,#30108),.UNSPECIFIED.,.F.,.F.,(4,2,2,2,2,2,2,2,2,2,2,2,2,
2,4),(-22.8315979776072,-22.6468550995409,-22.4614144304526,-22.1495542369066,
-21.8319967613863,-21.5198417749621,-21.2025574749825,-20.8900847176457,
-20.5730704622723,-20.2602584541901,-19.9435101871991,-19.6303391935868,
-19.3138519590932,-19.0003042009862,-18.8651569875978),.UNSPECIFIED.);
#331=B_SPLINE_CURVE_WITH_KNOTS('',3,(#30113,#30114,#30115,#30116,#30117,
#30118,#30119,#30120,#30121,#30122,#30123,#30124,#30125,#30126,#30127,#30128,
#30129,#30130,#30131,#30132,#30133,#30134,#30135,#30136,#30137,#30138,#30139,
#30140,#30141,#30142,#30143,#30144,#30145,#30146,#30147,#30148,#30149,#30150),
 .UNSPECIFIED.,.F.,.F.,(4,2,2,2,2,2,2,2,2,2,2,2,2,2,2,2,2,2,4),(-6.19306152073892,
-6.19215501284973,-5.88122082091077,-5.558699659647,-5.24769703205706,-4.92497158059589,
-4.61389148723222,-4.29096837903147,-3.9798031422975,-3.65668890928387,
-3.34543210441171,-3.02213314223365,-2.71077949168461,-2.38730203042346,
-2.07584729564655,-1.75219737570318,-1.44063824902751,-1.11682170183935,
-1.08763065698974),.UNSPECIFIED.);
#332=B_SPLINE_CURVE_WITH_KNOTS('',3,(#30151,#30152,#30153,#30154,#30155,
#30156,#30157,#30158,#30159,#30160,#30161,#30162,#30163,#30164,#30165,#30166,
#30167,#30168,#30169,#30170,#30171,#30172,#30173,#30174,#30175,#30176,#30177,
#30178,#30179,#30180,#30181,#30182,#30183,#30184,#30185,#30186),
 .UNSPECIFIED.,.F.,.F.,(4,2,2,2,2,2,2,2,2,2,2,2,2,2,2,2,2,4),(-18.8651569875978,
-18.6840721358553,-18.3701318810007,-18.0541483667636,-17.7398022919276,
-17.424059979304,-17.1092970137406,-16.7937878340886,-16.4785992730197,
-16.1633145468654,-15.84769404259,-15.5326245591325,-15.2165680717643,-14.9017041714821,
-14.5852098835831,-14.2705415421437,-13.9536097423191,-13.7714023393986),
 .UNSPECIFIED.);
#333=B_SPLINE_CURVE_WITH_KNOTS('',3,(#30191,#30192,#30193,#30194,#30195,
#30196,#30197,#30198,#30199,#30200,#30201,#30202,#30203,#30204,#30205,#30206,
#30207,#30208,#30209,#30210,#30211,#30212,#30213,#30214,#30215,#30216,#30217,
#30218,#30219,#30220,#30221,#30222,#30223,#30224,#30225,#30226),
 .UNSPECIFIED.,.F.,.F.,(4,2,2,2,2,2,2,2,2,2,2,2,2,2,2,2,2,4),(-11.2955132668756,
-11.2499663755103,-10.9350810181394,-10.618816702694,-10.3035134580392,
-9.98748241249118,-9.6766841977884,-9.35552796049665,-9.04474773802309,
-8.72334793560915,-8.4125672990213,-8.09093012940668,-7.78013227347285,
-7.45826415837377,-7.14743390049163,-6.82534141835785,-6.51446518933045,
-6.19306152073892),.UNSPECIFIED.);
#334=B_SPLINE_CURVE_WITH_KNOTS('',3,(#30227,#30228,#30229,#30230,#30231,
#30232,#30233,#30234,#30235,#30236,#30237,#30238,#30239,#30240,#30241,#30242,
#30243,#30244,#30245,#30246,#30247,#30248,#30249,#30250,#30251,#30252,#30253,
#30254,#30255,#30256,#30257,#30258,#30259,#30260,#30261,#30262),
 .UNSPECIFIED.,.F.,.F.,(4,2,2,2,2,2,2,2,2,2,2,2,2,2,2,2,2,4),(-13.7714023393986,
-13.6391266540991,-13.321759595108,-13.0074512547913,-12.6896529919331,
-12.375508772851,-12.0572849883311,-11.7432942164274,-11.4246520351327,
-11.1024784175165,-10.7919151734175,-10.469543341878,-10.1588960412222,
-9.83633253271426,-9.52559460027536,-9.20284582000664,-8.89201184020883,
-8.67522927952334),.UNSPECIFIED.);
#335=B_SPLINE_CURVE_WITH_KNOTS('',3,(#30268,#30269,#30270,#30271,#30272,
#30273,#30274,#30275,#30276,#30277,#30278,#30279,#30280,#30281,#30282,#30283,
#30284,#30285,#30286,#30287,#30288,#30289,#30290,#30291,#30292,#30293),
 .UNSPECIFIED.,.F.,.F.,(4,2,2,2,2,2,2,2,2,2,2,2,4),(-3.57460038523497,-3.48941625606424,
-3.17761372514257,-2.85332018035678,-2.54140882943066,-2.21698644756211,
-1.90496726499796,-1.5804197501514,-1.26829388464313,-0.943624715683776,
-0.631393435474488,-0.306605874008126,0.),.UNSPECIFIED.);
#336=B_SPLINE_CURVE_WITH_KNOTS('',3,(#30296,#30297,#30298,#30299,#30300,
#30301,#30302,#30303,#30304,#30305,#30306,#30307,#30308,#30309,#30310,#30311,
#30312,#30313,#30314,#30315,#30316,#30317,#30318,#30319,#30320,#30321),
 .UNSPECIFIED.,.F.,.F.,(4,2,2,2,2,2,2,2,2,2,2,2,4),(-19.9682012621818,-19.7098781597989,
-19.4484728160962,-19.1373255636262,-18.8175881446957,-18.5062982349599,
-18.1868340849252,-17.8753757400517,-17.5561870800245,-17.2445342177348,
-16.9256224526336,-16.613748987607,-16.3969931861447),.UNSPECIFIED.);
#337=B_SPLINE_CURVE_WITH_KNOTS('',3,(#30323,#30324,#30325,#30326,#30327,
#30328,#30329,#30330,#30331,#30332,#30333,#30334,#30335,#30336,#30337,#30338,
#30339,#30340,#30341,#30342,#30343,#30344,#30345,#30346,#30347,#30348,#30349,
#30350,#30351,#30352,#30353,#30354,#30355,#30356,#30357,#30358),
 .UNSPECIFIED.,.F.,.F.,(4,2,2,2,2,2,2,2,2,2,2,2,2,2,2,2,2,4),(-16.3969931861447,
-16.2951146586955,-15.9829948163869,-15.6646375641271,-15.3522460653515,
-15.0341645906407,-14.7214770909201,-14.4036691687269,-14.0906626928763,
-13.7731251587965,-13.4597782402757,-13.1425070036526,-12.8287999308234,
-12.5117900008011,-12.1977050268771,-11.8809505507568,-11.5664720626041,
-11.2955132668756),.UNSPECIFIED.);
#338=B_SPLINE_CURVE_WITH_KNOTS('',3,(#30359,#30360,#30361,#30362,#30363,
#30364,#30365,#30366,#30367,#30368,#30369,#30370,#30371,#30372,#30373,#30374,
#30375,#30376,#30377,#30378,#30379,#30380,#30381,#30382,#30383,#30384,#30385,
#30386,#30387,#30388,#30389,#30390,#30391,#30392,#30393,#30394),
 .UNSPECIFIED.,.F.,.F.,(4,2,2,2,2,2,2,2,2,2,2,2,2,2,2,2,2,4),(-8.67522927952334,
-8.56908403168542,-8.258149640719,-7.93504886100084,-7.6240106387303,-7.30074273855771,
-6.98959810256552,-6.6661687109744,-6.35491581460173,-6.03133032761751,
-5.71996796341123,-5.39623153639831,-5.08475904596485,-4.76087658920983,
-4.44929378011827,-4.1252699572342,-3.81357702730685,-3.57460038523497),
 .UNSPECIFIED.);
#339=B_SPLINE_CURVE_WITH_KNOTS('',3,(#30546,#30547,#30548,#30549,#30550,
#30551,#30552,#30553,#30554,#30555,#30556,#30557),.UNSPECIFIED.,.F.,.F.,
(4,2,2,2,2,4),(-0.792142372778785,-0.591597628920338,-0.397953596192907,
-0.200017601361334,-0.098121308975255,-1.00000001490574E-6),
 .UNSPECIFIED.);
#340=B_SPLINE_CURVE_WITH_KNOTS('',3,(#30558,#30559,#30560,#30561,#30562,
#30563,#30564,#30565,#30566,#30567),.UNSPECIFIED.,.F.,.F.,(4,2,2,2,4),(-0.755948032479872,
-0.604406814456052,-0.40541099667635,-0.208806710351552,0.),
 .UNSPECIFIED.);
#341=B_SPLINE_CURVE_WITH_KNOTS('',3,(#30879,#30880,#30881,#30882,#30883,
#30884,#30885,#30886,#30887,#30888,#30889,#30890,#30891,#30892,#30893,#30894,
#30895,#30896,#30897,#30898,#30899,#30900,#30901,#30902),.UNSPECIFIED.,
 .F.,.F.,(4,2,2,2,2,2,2,2,2,2,2,4),(1.0000000253329E-6,0.266750129365986,
0.536833672900569,0.866300625148748,1.19957484557901,1.52866431091697,1.8622200413073,
2.19095299525438,2.5247943758972,2.8531936331742,3.18732382651167,3.34852080740999),
 .UNSPECIFIED.);
#342=B_SPLINE_CURVE_WITH_KNOTS('',3,(#31162,#31163,#31164,#31165,#31166,
#31167,#31168,#31169,#31170,#31171,#31172,#31173,#31174,#31175,#31176,#31177,
#31178,#31179,#31180,#31181),.UNSPECIFIED.,.F.,.F.,(4,2,2,2,2,2,2,2,2,4),
(15.3747761103741,15.3773061828803,15.7191827319993,16.0479199119144,16.3899024459424,
16.7187368726242,17.060822934254,17.3897234764764,17.7317277368266,18.062135331452),
 .UNSPECIFIED.);
#343=B_SPLINE_CURVE_WITH_KNOTS('',3,(#32336,#32337,#32338,#32339,#32340,
#32341,#32342,#32343,#32344,#32345,#32346,#32347,#32348,#32349,#32350,#32351,
#32352,#32353,#32354,#32355,#32356,#32357,#32358,#32359,#32360,#32361,#32362,
#32363,#32364,#32365,#32366,#32367,#32368,#32369,#32370,#32371,#32372,#32373),
 .UNSPECIFIED.,.F.,.F.,(4,2,2,2,2,2,2,2,2,2,2,2,2,2,2,2,2,2,4),(-2.00453087624746,
-1.99784530757748,-1.9339539081977,-1.87134356757002,-1.80995795666769,
-1.74563396690078,-1.68374745704052,-1.6208256951135,-1.55732738492814,
-1.49614332060061,-1.43218556118532,-1.3693353892712,-1.30803770782599,
-1.24345350991551,-1.18132562328791,-1.11874004258405,-1.05497136296553,
-0.99359471855428,-0.991954268502835),.UNSPECIFIED.);
#344=B_SPLINE_CURVE_WITH_KNOTS('',3,(#32896,#32897,#32898,#32899,#32900,
#32901,#32902,#32903,#32904,#32905,#32906,#32907,#32908,#32909,#32910,#32911,
#32912,#32913,#32914,#32915,#32916,#32917,#32918,#32919,#32920,#32921,#32922,
#32923,#32924,#32925,#32926,#32927,#32928,#32929,#32930,#32931),
 .UNSPECIFIED.,.F.,.F.,(4,2,2,2,2,2,2,2,2,2,2,2,2,2,2,2,2,4),(-18.6261649225256,
-18.5964689905192,-18.5341509277396,-18.4703139576672,-18.4093686462651,
-18.346370722227,-18.2822619886212,-18.2207916693756,-18.1569179891035,
-18.0949490218438,-18.0327431791459,-17.9688572712294,-17.9078222340396,
-17.8449266834194,-17.7810584978724,-17.7196802765616,-17.6559086764456,
-17.614935493873),.UNSPECIFIED.);
#411=(
BOUNDED_SURFACE()
B_SPLINE_SURFACE(1,2,((#30592,#30593,#30594,#30595,#30596,#30597,#30598,
#30599,#30600,#30601,#30602,#30603,#30604,#30605,#30606,#30607,#30608,#30609,
#30610,#30611,#30612,#30613,#30614,#30615,#30616,#30617,#30618,#30619,#30620,
#30621,#30622,#30623,#30624,#30625,#30626,#30627,#30628,#30629,#30630,#30631,
#30632,#30633,#30634,#30635,#30636,#30637,#30638,#30639,#30640,#30641,#30642,
#30643,#30644,#30645,#30646,#30647,#30648,#30649,#30650,#30651,#30652,#30653,
#30654,#30655,#30656,#30657,#30658,#30659,#30660,#30661,#30662,#30663,#30664,
#30665,#30666,#30667,#30668,#30669,#30670,#30671,#30672,#30673,#30674,#30675,
#30676,#30677,#30678,#30679,#30680,#30681,#30682,#30683,#30684,#30685,#30686,
#30687,#30688,#30689,#30690,#30691,#30692,#30693,#30694,#30695,#30696,#30697,
#30698,#30699,#30700,#30701,#30702,#30703,#30704,#30705,#30706,#30707,#30708,
#30709,#30710,#30711,#30712,#30713,#30714,#30715,#30716,#30717,#30718,#30719,
#30720),(#30721,#30722,#30723,#30724,#30725,#30726,#30727,#30728,#30729,
#30730,#30731,#30732,#30733,#30734,#30735,#30736,#30737,#30738,#30739,#30740,
#30741,#30742,#30743,#30744,#30745,#30746,#30747,#30748,#30749,#30750,#30751,
#30752,#30753,#30754,#30755,#30756,#30757,#30758,#30759,#30760,#30761,#30762,
#30763,#30764,#30765,#30766,#30767,#30768,#30769,#30770,#30771,#30772,#30773,
#30774,#30775,#30776,#30777,#30778,#30779,#30780,#30781,#30782,#30783,#30784,
#30785,#30786,#30787,#30788,#30789,#30790,#30791,#30792,#30793,#30794,#30795,
#30796,#30797,#30798,#30799,#30800,#30801,#30802,#30803,#30804,#30805,#30806,
#30807,#30808,#30809,#30810,#30811,#30812,#30813,#30814,#30815,#30816,#30817,
#30818,#30819,#30820,#30821,#30822,#30823,#30824,#30825,#30826,#30827,#30828,
#30829,#30830,#30831,#30832,#30833,#30834,#30835,#30836,#30837,#30838,#30839,
#30840,#30841,#30842,#30843,#30844,#30845,#30846,#30847,#30848,#30849)),
 .UNSPECIFIED.,.F.,.F.,.F.)
B_SPLINE_SURFACE_WITH_KNOTS((2,2),(3,2,2,2,2,2,2,2,2,2,2,2,2,2,2,2,2,2,
2,2,2,2,2,2,2,2,2,2,2,2,2,2,2,2,2,2,2,2,2,2,2,2,2,2,2,2,2,2,2,2,2,2,2,2,
2,2,2,2,2,2,2,2,2,2,3),(-1.70594514575571E-6,1.),(0.,0.015625,0.03125,0.046875,
0.0625,0.078125,0.09375,0.109375,0.125,0.140625,0.15625,0.171875,0.1875,
0.203125,0.21875,0.234375,0.25,0.265625,0.28125,0.296875,0.3125,0.328125,
0.34375,0.359375,0.375,0.390625,0.40625,0.421875,0.4375,0.453125,0.46875,
0.484375,0.5,0.515625,0.53125,0.546875,0.5625,0.578125,0.59375,0.609375,
0.625,0.640625,0.65625,0.671875,0.6875,0.703125,0.71875,0.734375,0.75,0.765625,
0.78125,0.796875,0.8125,0.828125,0.84375,0.859375,0.875,0.890625,0.90625,
0.921875,0.9375,0.953125,0.96875,0.984375,1.),.UNSPECIFIED.)
GEOMETRIC_REPRESENTATION_ITEM()
RATIONAL_B_SPLINE_SURFACE(((1.,0.923879532511287,1.,0.923879532511287,1.,
0.923879532511287,1.,0.923879532511287,1.,0.923879532511287,1.,0.923879532511287,
1.,0.923879532511287,1.,0.923879532511287,1.,0.923879532511287,1.,0.923879532511287,
1.,0.923879532511287,1.,0.923879532511287,1.,0.923879532511287,1.,0.923879532511287,
1.,0.923879532511287,1.,0.923879532511287,1.,0.923879532511287,1.,0.923879532511287,
1.,0.923879532511287,1.,0.923879532511287,1.,0.923879532511287,1.,0.923879532511287,
1.,0.923879532511287,1.,0.923879532511287,1.,0.923879532511287,1.,0.923879532511287,
1.,0.923879532511287,1.,0.923879532511287,1.,0.923879532511287,1.,0.923879532511287,
1.,0.923879532511287,1.,0.923879532511287,1.,0.923879532511287,1.,0.923879532511287,
1.,0.923879532511287,1.,0.923879532511287,1.,0.923879532511287,1.,0.923879532511287,
1.,0.923879532511287,1.,0.923879532511287,1.,0.923879532511287,1.,0.923879532511287,
1.,0.923879532511287,1.,0.923879532511287,1.,0.923879532511287,1.,0.923879532511287,
1.,0.923879532511287,1.,0.923879532511287,1.,0.923879532511287,1.,0.923879532511287,
1.,0.923879532511287,1.,0.923879532511287,1.,0.923879532511287,1.,0.923879532511287,
1.,0.923879532511287,1.,0.923879532511287,1.,0.923879532511287,1.,0.923879532511287,
1.,0.923879532511287,1.,0.923879532511287,1.,0.923879532511287,1.,0.923879532511287,
1.,0.923879532511287,1.,0.923879532511287,1.),(1.,0.923879532511287,1.,
0.923879532511287,1.,0.923879532511287,1.,0.923879532511287,1.,0.923879532511287,
1.,0.923879532511287,1.,0.923879532511287,1.,0.923879532511287,1.,0.923879532511287,
1.,0.923879532511287,1.,0.923879532511287,1.,0.923879532511287,1.,0.923879532511287,
1.,0.923879532511287,1.,0.923879532511287,1.,0.923879532511287,1.,0.923879532511287,
1.,0.923879532511287,1.,0.923879532511287,1.,0.923879532511287,1.,0.923879532511287,
1.,0.923879532511287,1.,0.923879532511287,1.,0.923879532511287,1.,0.923879532511287,
1.,0.923879532511287,1.,0.923879532511287,1.,0.923879532511287,1.,0.923879532511287,
1.,0.923879532511287,1.,0.923879532511287,1.,0.923879532511287,1.,0.923879532511287,
1.,0.923879532511287,1.,0.923879532511287,1.,0.923879532511287,1.,0.923879532511287,
1.,0.923879532511287,1.,0.923879532511287,1.,0.923879532511287,1.,0.923879532511287,
1.,0.923879532511287,1.,0.923879532511287,1.,0.923879532511287,1.,0.923879532511287,
1.,0.923879532511287,1.,0.923879532511287,1.,0.923879532511287,1.,0.923879532511287,
1.,0.923879532511287,1.,0.923879532511287,1.,0.923879532511287,1.,0.923879532511287,
1.,0.923879532511287,1.,0.923879532511287,1.,0.923879532511287,1.,0.923879532511287,
1.,0.923879532511287,1.,0.923879532511287,1.,0.923879532511287,1.,0.923879532511287,
1.,0.923879532511287,1.,0.923879532511287,1.,0.923879532511287,1.)))
REPRESENTATION_ITEM('')
SURFACE()
);
#412=(
BOUNDED_SURFACE()
B_SPLINE_SURFACE(1,2,((#30903,#30904,#30905,#30906,#30907,#30908,#30909,
#30910,#30911,#30912,#30913,#30914,#30915,#30916,#30917,#30918,#30919,#30920,
#30921,#30922,#30923,#30924,#30925,#30926,#30927,#30928,#30929,#30930,#30931,
#30932,#30933,#30934,#30935,#30936,#30937,#30938,#30939,#30940,#30941,#30942,
#30943,#30944,#30945,#30946,#30947,#30948,#30949,#30950,#30951,#30952,#30953,
#30954,#30955,#30956,#30957,#30958,#30959,#30960,#30961,#30962,#30963,#30964,
#30965,#30966,#30967,#30968,#30969,#30970,#30971,#30972,#30973,#30974,#30975,
#30976,#30977,#30978,#30979,#30980,#30981,#30982,#30983,#30984,#30985,#30986,
#30987,#30988,#30989,#30990,#30991,#30992,#30993,#30994,#30995,#30996,#30997,
#30998,#30999,#31000,#31001,#31002,#31003,#31004,#31005,#31006,#31007,#31008,
#31009,#31010,#31011,#31012,#31013,#31014,#31015,#31016,#31017,#31018,#31019,
#31020,#31021,#31022,#31023,#31024,#31025,#31026,#31027,#31028,#31029,#31030,
#31031),(#31032,#31033,#31034,#31035,#31036,#31037,#31038,#31039,#31040,
#31041,#31042,#31043,#31044,#31045,#31046,#31047,#31048,#31049,#31050,#31051,
#31052,#31053,#31054,#31055,#31056,#31057,#31058,#31059,#31060,#31061,#31062,
#31063,#31064,#31065,#31066,#31067,#31068,#31069,#31070,#31071,#31072,#31073,
#31074,#31075,#31076,#31077,#31078,#31079,#31080,#31081,#31082,#31083,#31084,
#31085,#31086,#31087,#31088,#31089,#31090,#31091,#31092,#31093,#31094,#31095,
#31096,#31097,#31098,#31099,#31100,#31101,#31102,#31103,#31104,#31105,#31106,
#31107,#31108,#31109,#31110,#31111,#31112,#31113,#31114,#31115,#31116,#31117,
#31118,#31119,#31120,#31121,#31122,#31123,#31124,#31125,#31126,#31127,#31128,
#31129,#31130,#31131,#31132,#31133,#31134,#31135,#31136,#31137,#31138,#31139,
#31140,#31141,#31142,#31143,#31144,#31145,#31146,#31147,#31148,#31149,#31150,
#31151,#31152,#31153,#31154,#31155,#31156,#31157,#31158,#31159,#31160)),
 .UNSPECIFIED.,.F.,.F.,.F.)
B_SPLINE_SURFACE_WITH_KNOTS((2,2),(3,2,2,2,2,2,2,2,2,2,2,2,2,2,2,2,2,2,
2,2,2,2,2,2,2,2,2,2,2,2,2,2,2,2,2,2,2,2,2,2,2,2,2,2,2,2,2,2,2,2,2,2,2,2,
2,2,2,2,2,2,2,2,2,2,3),(0.,1.00002504461482),(0.,0.015625,0.03125,0.046875,
0.0625,0.078125,0.09375,0.109375,0.125,0.140625,0.15625,0.171875,0.1875,
0.203125,0.21875,0.234375,0.25,0.265625,0.28125,0.296875,0.3125,0.328125,
0.34375,0.359375,0.375,0.390625,0.40625,0.421875,0.4375,0.453125,0.46875,
0.484375,0.5,0.515625,0.53125,0.546875,0.5625,0.578125,0.59375,0.609375,
0.625,0.640625,0.65625,0.671875,0.6875,0.703125,0.71875,0.734375,0.75,0.765625,
0.78125,0.796875,0.8125,0.828125,0.84375,0.859375,0.875,0.890625,0.90625,
0.921875,0.9375,0.953125,0.96875,0.984375,1.),.UNSPECIFIED.)
GEOMETRIC_REPRESENTATION_ITEM()
RATIONAL_B_SPLINE_SURFACE(((1.,0.923879532511287,1.,0.923879532511287,1.,
0.923879532511287,1.,0.923879532511287,1.,0.923879532511287,1.,0.923879532511287,
1.,0.923879532511287,1.,0.923879532511287,1.,0.923879532511287,1.,0.923879532511287,
1.,0.923879532511287,1.,0.923879532511287,1.,0.923879532511287,1.,0.923879532511287,
1.,0.923879532511287,1.,0.923879532511287,1.,0.923879532511287,1.,0.923879532511287,
1.,0.923879532511287,1.,0.923879532511287,1.,0.923879532511287,1.,0.923879532511287,
1.,0.923879532511287,1.,0.923879532511287,1.,0.923879532511287,1.,0.923879532511287,
1.,0.923879532511287,1.,0.923879532511287,1.,0.923879532511287,1.,0.923879532511287,
1.,0.923879532511287,1.,0.923879532511287,1.,0.923879532511287,1.,0.923879532511287,
1.,0.923879532511287,1.,0.923879532511287,1.,0.923879532511287,1.,0.923879532511287,
1.,0.923879532511287,1.,0.923879532511287,1.,0.923879532511287,1.,0.923879532511287,
1.,0.923879532511287,1.,0.923879532511287,1.,0.923879532511287,1.,0.923879532511287,
1.,0.923879532511287,1.,0.923879532511287,1.,0.923879532511287,1.,0.923879532511287,
1.,0.923879532511287,1.,0.923879532511287,1.,0.923879532511287,1.,0.923879532511287,
1.,0.923879532511287,1.,0.923879532511287,1.,0.923879532511287,1.,0.923879532511287,
1.,0.923879532511287,1.,0.923879532511287,1.,0.923879532511287,1.,0.923879532511287,
1.,0.923879532511287,1.,0.923879532511287,1.),(1.,0.923879532511287,1.,
0.923879532511287,1.,0.923879532511287,1.,0.923879532511287,1.,0.923879532511287,
1.,0.923879532511287,1.,0.923879532511287,1.,0.923879532511287,1.,0.923879532511287,
1.,0.923879532511287,1.,0.923879532511287,1.,0.923879532511287,1.,0.923879532511287,
1.,0.923879532511287,1.,0.923879532511287,1.,0.923879532511287,1.,0.923879532511287,
1.,0.923879532511287,1.,0.923879532511287,1.,0.923879532511287,1.,0.923879532511287,
1.,0.923879532511287,1.,0.923879532511287,1.,0.923879532511287,1.,0.923879532511287,
1.,0.923879532511287,1.,0.923879532511287,1.,0.923879532511287,1.,0.923879532511287,
1.,0.923879532511287,1.,0.923879532511287,1.,0.923879532511287,1.,0.923879532511287,
1.,0.923879532511287,1.,0.923879532511287,1.,0.923879532511287,1.,0.923879532511287,
1.,0.923879532511287,1.,0.923879532511287,1.,0.923879532511287,1.,0.923879532511287,
1.,0.923879532511287,1.,0.923879532511287,1.,0.923879532511287,1.,0.923879532511287,
1.,0.923879532511287,1.,0.923879532511287,1.,0.923879532511287,1.,0.923879532511287,
1.,0.923879532511287,1.,0.923879532511287,1.,0.923879532511287,1.,0.923879532511287,
1.,0.923879532511287,1.,0.923879532511287,1.,0.923879532511287,1.,0.923879532511287,
1.,0.923879532511287,1.,0.923879532511287,1.,0.923879532511287,1.,0.923879532511287,
1.,0.923879532511287,1.,0.923879532511287,1.,0.923879532511287,1.)))
REPRESENTATION_ITEM('')
SURFACE()
);
#413=(
BOUNDED_SURFACE()
B_SPLINE_SURFACE(1,2,((#31853,#31854,#31855,#31856,#31857,#31858,#31859,
#31860,#31861,#31862,#31863,#31864,#31865,#31866,#31867,#31868,#31869,#31870,
#31871,#31872,#31873,#31874,#31875,#31876,#31877,#31878,#31879,#31880,#31881,
#31882,#31883,#31884,#31885,#31886,#31887,#31888,#31889,#31890,#31891,#31892,
#31893,#31894,#31895,#31896,#31897,#31898,#31899,#31900,#31901,#31902,#31903,
#31904,#31905,#31906,#31907,#31908,#31909,#31910,#31911,#31912,#31913,#31914,
#31915,#31916,#31917,#31918,#31919,#31920,#31921,#31922,#31923,#31924,#31925,
#31926,#31927,#31928,#31929,#31930,#31931,#31932,#31933,#31934,#31935,#31936,
#31937,#31938,#31939,#31940,#31941,#31942,#31943,#31944,#31945,#31946,#31947,
#31948,#31949,#31950,#31951,#31952,#31953,#31954,#31955,#31956,#31957,#31958,
#31959,#31960,#31961,#31962,#31963,#31964,#31965,#31966,#31967,#31968,#31969,
#31970,#31971,#31972,#31973,#31974,#31975,#31976,#31977,#31978,#31979,#31980,
#31981,#31982,#31983,#31984,#31985,#31986,#31987,#31988,#31989,#31990,#31991,
#31992,#31993,#31994,#31995,#31996,#31997,#31998,#31999,#32000,#32001,#32002,
#32003,#32004,#32005,#32006,#32007,#32008,#32009,#32010,#32011,#32012,#32013,
#32014,#32015,#32016,#32017,#32018,#32019,#32020,#32021,#32022,#32023,#32024,
#32025,#32026,#32027,#32028,#32029,#32030,#32031,#32032,#32033,#32034,#32035,
#32036,#32037,#32038,#32039,#32040,#32041,#32042,#32043,#32044,#32045,#32046,
#32047,#32048,#32049,#32050,#32051,#32052,#32053,#32054,#32055,#32056,#32057,
#32058,#32059,#32060,#32061,#32062,#32063,#32064,#32065,#32066,#32067,#32068,
#32069,#32070,#32071,#32072,#32073,#32074,#32075,#32076,#32077,#32078,#32079,
#32080,#32081,#32082,#32083,#32084,#32085,#32086,#32087,#32088,#32089,#32090,
#32091,#32092,#32093),(#32094,#32095,#32096,#32097,#32098,#32099,#32100,
#32101,#32102,#32103,#32104,#32105,#32106,#32107,#32108,#32109,#32110,#32111,
#32112,#32113,#32114,#32115,#32116,#32117,#32118,#32119,#32120,#32121,#32122,
#32123,#32124,#32125,#32126,#32127,#32128,#32129,#32130,#32131,#32132,#32133,
#32134,#32135,#32136,#32137,#32138,#32139,#32140,#32141,#32142,#32143,#32144,
#32145,#32146,#32147,#32148,#32149,#32150,#32151,#32152,#32153,#32154,#32155,
#32156,#32157,#32158,#32159,#32160,#32161,#32162,#32163,#32164,#32165,#32166,
#32167,#32168,#32169,#32170,#32171,#32172,#32173,#32174,#32175,#32176,#32177,
#32178,#32179,#32180,#32181,#32182,#32183,#32184,#32185,#32186,#32187,#32188,
#32189,#32190,#32191,#32192,#32193,#32194,#32195,#32196,#32197,#32198,#32199,
#32200,#32201,#32202,#32203,#32204,#32205,#32206,#32207,#32208,#32209,#32210,
#32211,#32212,#32213,#32214,#32215,#32216,#32217,#32218,#32219,#32220,#32221,
#32222,#32223,#32224,#32225,#32226,#32227,#32228,#32229,#32230,#32231,#32232,
#32233,#32234,#32235,#32236,#32237,#32238,#32239,#32240,#32241,#32242,#32243,
#32244,#32245,#32246,#32247,#32248,#32249,#32250,#32251,#32252,#32253,#32254,
#32255,#32256,#32257,#32258,#32259,#32260,#32261,#32262,#32263,#32264,#32265,
#32266,#32267,#32268,#32269,#32270,#32271,#32272,#32273,#32274,#32275,#32276,
#32277,#32278,#32279,#32280,#32281,#32282,#32283,#32284,#32285,#32286,#32287,
#32288,#32289,#32290,#32291,#32292,#32293,#32294,#32295,#32296,#32297,#32298,
#32299,#32300,#32301,#32302,#32303,#32304,#32305,#32306,#32307,#32308,#32309,
#32310,#32311,#32312,#32313,#32314,#32315,#32316,#32317,#32318,#32319,#32320,
#32321,#32322,#32323,#32324,#32325,#32326,#32327,#32328,#32329,#32330,#32331,
#32332,#32333,#32334)),.UNSPECIFIED.,.F.,.F.,.F.)
B_SPLINE_SURFACE_WITH_KNOTS((2,2),(3,2,2,2,2,2,2,2,2,2,2,2,2,2,2,2,2,2,
2,2,2,2,2,2,2,2,2,2,2,2,2,2,2,2,2,2,2,2,2,2,2,2,2,2,2,2,2,2,2,2,2,2,2,2,
2,2,2,2,2,2,2,2,2,2,2,2,2,2,2,2,2,2,2,2,2,2,2,2,2,2,2,2,2,2,2,2,2,2,2,2,
2,2,2,2,2,2,2,2,2,2,2,2,2,2,2,2,2,2,2,2,2,2,2,2,2,2,2,2,2,2,3),(0.,1.),
(0.,0.00833333333333333,0.0166666666666666,0.025,0.0333333333333333,0.0416666666666667,
0.05,0.0583333333333333,0.0666666666666667,0.075,0.0833333333333333,0.0916666666666667,
0.1,0.108333333333333,0.116666666666667,0.125,0.133333333333333,0.141666666666667,
0.15,0.158333333333333,0.166666666666667,0.175,0.183333333333334,0.191666666666667,
0.2,0.208333333333334,0.216666666666667,0.225,0.233333333333334,0.241666666666667,
0.25,0.258333333333334,0.266666666666666,0.275,0.283333333333334,0.291666666666667,
0.3,0.308333333333334,0.316666666666666,0.325,0.333333333333334,0.341666666666667,
0.35,0.358333333333334,0.366666666666666,0.375,0.383333333333334,0.391666666666666,
0.4,0.408333333333334,0.416666666666667,0.425,0.433333333333334,0.441666666666666,
0.45,0.458333333333333,0.466666666666667,0.475,0.483333333333333,0.491666666666667,
0.5,0.508333333333333,0.516666666666667,0.525,0.533333333333333,0.541666666666667,
0.55,0.558333333333333,0.566666666666667,0.575,0.583333333333333,0.591666666666667,
0.6,0.608333333333333,0.616666666666667,0.625,0.633333333333333,0.641666666666667,
0.65,0.658333333333333,0.666666666666667,0.675,0.683333333333333,0.691666666666667,
0.7,0.708333333333333,0.716666666666667,0.725,0.733333333333333,0.741666666666667,
0.75,0.758333333333333,0.766666666666667,0.775,0.783333333333333,0.791666666666667,
0.8,0.808333333333333,0.816666666666667,0.825,0.833333333333333,0.841666666666667,
0.85,0.858333333333333,0.866666666666667,0.875,0.883333333333333,0.891666666666667,
0.9,0.908333333333333,0.916666666666667,0.925,0.933333333333333,0.941666666666667,
0.95,0.958333333333333,0.966666666666667,0.975,0.983333333333333,0.991666666666667,
1.),.UNSPECIFIED.)
GEOMETRIC_REPRESENTATION_ITEM()
RATIONAL_B_SPLINE_SURFACE(((1.,0.866025403784439,1.,0.866025403784439,1.,
0.866025403784439,1.,0.866025403784439,1.,0.866025403784439,1.,0.866025403784439,
1.,0.866025403784439,1.,0.866025403784439,1.,0.866025403784439,1.,0.866025403784439,
1.,0.866025403784439,1.,0.866025403784439,1.,0.866025403784439,1.,0.866025403784439,
1.,0.866025403784439,1.,0.866025403784439,1.,0.866025403784439,1.,0.866025403784439,
1.,0.866025403784439,1.,0.866025403784439,1.,0.866025403784439,1.,0.866025403784439,
1.,0.866025403784439,1.,0.866025403784439,1.,0.866025403784439,1.,0.866025403784439,
1.,0.866025403784439,1.,0.866025403784439,1.,0.866025403784439,1.,0.866025403784439,
1.,0.866025403784439,1.,0.866025403784439,1.,0.866025403784439,1.,0.866025403784439,
1.,0.866025403784439,1.,0.866025403784439,1.,0.866025403784439,1.,0.866025403784439,
1.,0.866025403784439,1.,0.866025403784439,1.,0.866025403784439,1.,0.866025403784439,
1.,0.866025403784439,1.,0.866025403784439,1.,0.866025403784439,1.,0.866025403784439,
1.,0.866025403784439,1.,0.866025403784439,1.,0.866025403784439,1.,0.866025403784439,
1.,0.866025403784439,1.,0.866025403784439,1.,0.866025403784439,1.,0.866025403784439,
1.,0.866025403784439,1.,0.866025403784439,1.,0.866025403784439,1.,0.866025403784439,
1.,0.866025403784439,1.,0.866025403784439,1.,0.866025403784439,1.,0.866025403784439,
1.,0.866025403784439,1.,0.866025403784439,1.,0.866025403784439,1.,0.866025403784439,
1.,0.866025403784439,1.,0.866025403784439,1.,0.866025403784439,1.,0.866025403784439,
1.,0.866025403784439,1.,0.866025403784439,1.,0.866025403784439,1.,0.866025403784439,
1.,0.866025403784439,1.,0.866025403784439,1.,0.866025403784439,1.,0.866025403784439,
1.,0.866025403784439,1.,0.866025403784439,1.,0.866025403784439,1.,0.866025403784439,
1.,0.866025403784439,1.,0.866025403784439,1.,0.866025403784439,1.,0.866025403784439,
1.,0.866025403784439,1.,0.866025403784439,1.,0.866025403784439,1.,0.866025403784439,
1.,0.866025403784439,1.,0.866025403784439,1.,0.866025403784439,1.,0.866025403784439,
1.,0.866025403784439,1.,0.866025403784439,1.,0.866025403784439,1.,0.866025403784439,
1.,0.866025403784439,1.,0.866025403784439,1.,0.866025403784439,1.,0.866025403784439,
1.,0.866025403784439,1.,0.866025403784439,1.,0.866025403784439,1.,0.866025403784439,
1.,0.866025403784439,1.,0.866025403784439,1.,0.866025403784439,1.,0.866025403784439,
1.,0.866025403784439,1.,0.866025403784439,1.,0.866025403784439,1.,0.866025403784439,
1.,0.866025403784439,1.,0.866025403784439,1.,0.866025403784439,1.,0.866025403784439,
1.,0.866025403784439,1.,0.866025403784439,1.),(1.,0.866025403784439,1.,
0.866025403784439,1.,0.866025403784439,1.,0.866025403784439,1.,0.866025403784439,
1.,0.866025403784439,1.,0.866025403784439,1.,0.866025403784439,1.,0.866025403784439,
1.,0.866025403784439,1.,0.866025403784439,1.,0.866025403784439,1.,0.866025403784439,
1.,0.866025403784439,1.,0.866025403784439,1.,0.866025403784439,1.,0.866025403784439,
1.,0.866025403784439,1.,0.866025403784439,1.,0.866025403784439,1.,0.866025403784439,
1.,0.866025403784439,1.,0.866025403784439,1.,0.866025403784439,1.,0.866025403784439,
1.,0.866025403784439,1.,0.866025403784439,1.,0.866025403784439,1.,0.866025403784439,
1.,0.866025403784439,1.,0.866025403784439,1.,0.866025403784439,1.,0.866025403784439,
1.,0.866025403784439,1.,0.866025403784439,1.,0.866025403784439,1.,0.866025403784439,
1.,0.866025403784439,1.,0.866025403784439,1.,0.866025403784439,1.,0.866025403784439,
1.,0.866025403784439,1.,0.866025403784439,1.,0.866025403784439,1.,0.866025403784439,
1.,0.866025403784439,1.,0.866025403784439,1.,0.866025403784439,1.,0.866025403784439,
1.,0.866025403784439,1.,0.866025403784439,1.,0.866025403784439,1.,0.866025403784439,
1.,0.866025403784439,1.,0.866025403784439,1.,0.866025403784439,1.,0.866025403784439,
1.,0.866025403784439,1.,0.866025403784439,1.,0.866025403784439,1.,0.866025403784439,
1.,0.866025403784439,1.,0.866025403784439,1.,0.866025403784439,1.,0.866025403784439,
1.,0.866025403784439,1.,0.866025403784439,1.,0.866025403784439,1.,0.866025403784439,
1.,0.866025403784439,1.,0.866025403784439,1.,0.866025403784439,1.,0.866025403784439,
1.,0.866025403784439,1.,0.866025403784439,1.,0.866025403784439,1.,0.866025403784439,
1.,0.866025403784439,1.,0.866025403784439,1.,0.866025403784439,1.,0.866025403784439,
1.,0.866025403784439,1.,0.866025403784439,1.,0.866025403784439,1.,0.866025403784439,
1.,0.866025403784439,1.,0.866025403784439,1.,0.866025403784439,1.,0.866025403784439,
1.,0.866025403784439,1.,0.866025403784439,1.,0.866025403784439,1.,0.866025403784439,
1.,0.866025403784439,1.,0.866025403784439,1.,0.866025403784439,1.,0.866025403784439,
1.,0.866025403784439,1.,0.866025403784439,1.,0.866025403784439,1.,0.866025403784439,
1.,0.866025403784439,1.,0.866025403784439,1.,0.866025403784439,1.,0.866025403784439,
1.,0.866025403784439,1.,0.866025403784439,1.,0.866025403784439,1.,0.866025403784439,
1.,0.866025403784439,1.,0.866025403784439,1.,0.866025403784439,1.,0.866025403784439,
1.,0.866025403784439,1.,0.866025403784439,1.,0.866025403784439,1.,0.866025403784439,
1.,0.866025403784439,1.,0.866025403784439,1.,0.866025403784439,1.)))
REPRESENTATION_ITEM('')
SURFACE()
);
#414=(
BOUNDED_SURFACE()
B_SPLINE_SURFACE(1,2,((#32411,#32412,#32413,#32414,#32415,#32416,#32417,
#32418,#32419,#32420,#32421,#32422,#32423,#32424,#32425,#32426,#32427,#32428,
#32429,#32430,#32431,#32432,#32433,#32434,#32435,#32436,#32437,#32438,#32439,
#32440,#32441,#32442,#32443,#32444,#32445,#32446,#32447,#32448,#32449,#32450,
#32451,#32452,#32453,#32454,#32455,#32456,#32457,#32458,#32459,#32460,#32461,
#32462,#32463,#32464,#32465,#32466,#32467,#32468,#32469,#32470,#32471,#32472,
#32473,#32474,#32475,#32476,#32477,#32478,#32479,#32480,#32481,#32482,#32483,
#32484,#32485,#32486,#32487,#32488,#32489,#32490,#32491,#32492,#32493,#32494,
#32495,#32496,#32497,#32498,#32499,#32500,#32501,#32502,#32503,#32504,#32505,
#32506,#32507,#32508,#32509,#32510,#32511,#32512,#32513,#32514,#32515,#32516,
#32517,#32518,#32519,#32520,#32521,#32522,#32523,#32524,#32525,#32526,#32527,
#32528,#32529,#32530,#32531,#32532,#32533,#32534,#32535,#32536,#32537,#32538,
#32539,#32540,#32541,#32542,#32543,#32544,#32545,#32546,#32547,#32548,#32549,
#32550,#32551,#32552,#32553,#32554,#32555,#32556,#32557,#32558,#32559,#32560,
#32561,#32562,#32563,#32564,#32565,#32566,#32567,#32568,#32569,#32570,#32571,
#32572,#32573,#32574,#32575,#32576,#32577,#32578,#32579,#32580,#32581,#32582,
#32583,#32584,#32585,#32586,#32587,#32588,#32589,#32590,#32591,#32592,#32593,
#32594,#32595,#32596,#32597,#32598,#32599,#32600,#32601,#32602,#32603,#32604,
#32605,#32606,#32607,#32608,#32609,#32610,#32611,#32612,#32613,#32614,#32615,
#32616,#32617,#32618,#32619,#32620,#32621,#32622,#32623,#32624,#32625,#32626,
#32627,#32628,#32629,#32630,#32631,#32632,#32633,#32634,#32635,#32636,#32637,
#32638,#32639,#32640,#32641,#32642,#32643,#32644,#32645,#32646,#32647,#32648,
#32649,#32650,#32651),(#32652,#32653,#32654,#32655,#32656,#32657,#32658,
#32659,#32660,#32661,#32662,#32663,#32664,#32665,#32666,#32667,#32668,#32669,
#32670,#32671,#32672,#32673,#32674,#32675,#32676,#32677,#32678,#32679,#32680,
#32681,#32682,#32683,#32684,#32685,#32686,#32687,#32688,#32689,#32690,#32691,
#32692,#32693,#32694,#32695,#32696,#32697,#32698,#32699,#32700,#32701,#32702,
#32703,#32704,#32705,#32706,#32707,#32708,#32709,#32710,#32711,#32712,#32713,
#32714,#32715,#32716,#32717,#32718,#32719,#32720,#32721,#32722,#32723,#32724,
#32725,#32726,#32727,#32728,#32729,#32730,#32731,#32732,#32733,#32734,#32735,
#32736,#32737,#32738,#32739,#32740,#32741,#32742,#32743,#32744,#32745,#32746,
#32747,#32748,#32749,#32750,#32751,#32752,#32753,#32754,#32755,#32756,#32757,
#32758,#32759,#32760,#32761,#32762,#32763,#32764,#32765,#32766,#32767,#32768,
#32769,#32770,#32771,#32772,#32773,#32774,#32775,#32776,#32777,#32778,#32779,
#32780,#32781,#32782,#32783,#32784,#32785,#32786,#32787,#32788,#32789,#32790,
#32791,#32792,#32793,#32794,#32795,#32796,#32797,#32798,#32799,#32800,#32801,
#32802,#32803,#32804,#32805,#32806,#32807,#32808,#32809,#32810,#32811,#32812,
#32813,#32814,#32815,#32816,#32817,#32818,#32819,#32820,#32821,#32822,#32823,
#32824,#32825,#32826,#32827,#32828,#32829,#32830,#32831,#32832,#32833,#32834,
#32835,#32836,#32837,#32838,#32839,#32840,#32841,#32842,#32843,#32844,#32845,
#32846,#32847,#32848,#32849,#32850,#32851,#32852,#32853,#32854,#32855,#32856,
#32857,#32858,#32859,#32860,#32861,#32862,#32863,#32864,#32865,#32866,#32867,
#32868,#32869,#32870,#32871,#32872,#32873,#32874,#32875,#32876,#32877,#32878,
#32879,#32880,#32881,#32882,#32883,#32884,#32885,#32886,#32887,#32888,#32889,
#32890,#32891,#32892)),.UNSPECIFIED.,.F.,.F.,.F.)
B_SPLINE_SURFACE_WITH_KNOTS((2,2),(3,2,2,2,2,2,2,2,2,2,2,2,2,2,2,2,2,2,
2,2,2,2,2,2,2,2,2,2,2,2,2,2,2,2,2,2,2,2,2,2,2,2,2,2,2,2,2,2,2,2,2,2,2,2,
2,2,2,2,2,2,2,2,2,2,2,2,2,2,2,2,2,2,2,2,2,2,2,2,2,2,2,2,2,2,2,2,2,2,2,2,
2,2,2,2,2,2,2,2,2,2,2,2,2,2,2,2,2,2,2,2,2,2,2,2,2,2,2,2,2,2,3),(0.,1.),
(0.,0.00833333333333333,0.0166666666666666,0.025,0.0333333333333333,0.0416666666666667,
0.05,0.0583333333333333,0.0666666666666667,0.075,0.0833333333333333,0.0916666666666667,
0.1,0.108333333333333,0.116666666666667,0.125,0.133333333333333,0.141666666666667,
0.15,0.158333333333333,0.166666666666667,0.175,0.183333333333334,0.191666666666667,
0.2,0.208333333333334,0.216666666666667,0.225,0.233333333333334,0.241666666666667,
0.25,0.258333333333334,0.266666666666666,0.275,0.283333333333334,0.291666666666667,
0.3,0.308333333333334,0.316666666666666,0.325,0.333333333333334,0.341666666666667,
0.35,0.358333333333334,0.366666666666666,0.375,0.383333333333334,0.391666666666666,
0.4,0.408333333333334,0.416666666666667,0.425,0.433333333333334,0.441666666666666,
0.45,0.458333333333333,0.466666666666667,0.475,0.483333333333333,0.491666666666667,
0.5,0.508333333333333,0.516666666666667,0.525,0.533333333333333,0.541666666666667,
0.55,0.558333333333333,0.566666666666667,0.575,0.583333333333333,0.591666666666667,
0.6,0.608333333333333,0.616666666666667,0.625,0.633333333333333,0.641666666666667,
0.65,0.658333333333333,0.666666666666667,0.675,0.683333333333333,0.691666666666667,
0.7,0.708333333333333,0.716666666666667,0.725,0.733333333333333,0.741666666666667,
0.75,0.758333333333333,0.766666666666667,0.775,0.783333333333333,0.791666666666667,
0.8,0.808333333333333,0.816666666666667,0.825,0.833333333333333,0.841666666666667,
0.85,0.858333333333333,0.866666666666667,0.875,0.883333333333333,0.891666666666667,
0.9,0.908333333333333,0.916666666666667,0.925,0.933333333333333,0.941666666666667,
0.95,0.958333333333333,0.966666666666667,0.975,0.983333333333333,0.991666666666667,
1.),.UNSPECIFIED.)
GEOMETRIC_REPRESENTATION_ITEM()
RATIONAL_B_SPLINE_SURFACE(((1.,0.866025403784439,1.,0.866025403784439,1.,
0.866025403784439,1.,0.866025403784439,1.,0.866025403784439,1.,0.866025403784439,
1.,0.866025403784439,1.,0.866025403784439,1.,0.866025403784439,1.,0.866025403784439,
1.,0.866025403784439,1.,0.866025403784439,1.,0.866025403784439,1.,0.866025403784439,
1.,0.866025403784439,1.,0.866025403784439,1.,0.866025403784439,1.,0.866025403784439,
1.,0.866025403784439,1.,0.866025403784439,1.,0.866025403784439,1.,0.866025403784439,
1.,0.866025403784439,1.,0.866025403784439,1.,0.866025403784439,1.,0.866025403784439,
1.,0.866025403784439,1.,0.866025403784439,1.,0.866025403784439,1.,0.866025403784439,
1.,0.866025403784439,1.,0.866025403784439,1.,0.866025403784439,1.,0.866025403784439,
1.,0.866025403784439,1.,0.866025403784439,1.,0.866025403784439,1.,0.866025403784439,
1.,0.866025403784439,1.,0.866025403784439,1.,0.866025403784439,1.,0.866025403784439,
1.,0.866025403784439,1.,0.866025403784439,1.,0.866025403784439,1.,0.866025403784439,
1.,0.866025403784439,1.,0.866025403784439,1.,0.866025403784439,1.,0.866025403784439,
1.,0.866025403784439,1.,0.866025403784439,1.,0.866025403784439,1.,0.866025403784439,
1.,0.866025403784439,1.,0.866025403784439,1.,0.866025403784439,1.,0.866025403784439,
1.,0.866025403784439,1.,0.866025403784439,1.,0.866025403784439,1.,0.866025403784439,
1.,0.866025403784439,1.,0.866025403784439,1.,0.866025403784439,1.,0.866025403784439,
1.,0.866025403784439,1.,0.866025403784439,1.,0.866025403784439,1.,0.866025403784439,
1.,0.866025403784439,1.,0.866025403784439,1.,0.866025403784439,1.,0.866025403784439,
1.,0.866025403784439,1.,0.866025403784439,1.,0.866025403784439,1.,0.866025403784439,
1.,0.866025403784439,1.,0.866025403784439,1.,0.866025403784439,1.,0.866025403784439,
1.,0.866025403784439,1.,0.866025403784439,1.,0.866025403784439,1.,0.866025403784439,
1.,0.866025403784439,1.,0.866025403784439,1.,0.866025403784439,1.,0.866025403784439,
1.,0.866025403784439,1.,0.866025403784439,1.,0.866025403784439,1.,0.866025403784439,
1.,0.866025403784439,1.,0.866025403784439,1.,0.866025403784439,1.,0.866025403784439,
1.,0.866025403784439,1.,0.866025403784439,1.,0.866025403784439,1.,0.866025403784439,
1.,0.866025403784439,1.,0.866025403784439,1.,0.866025403784439,1.,0.866025403784439,
1.,0.866025403784439,1.,0.866025403784439,1.,0.866025403784439,1.,0.866025403784439,
1.,0.866025403784439,1.,0.866025403784439,1.,0.866025403784439,1.,0.866025403784439,
1.,0.866025403784439,1.,0.866025403784439,1.,0.866025403784439,1.,0.866025403784439,
1.,0.866025403784439,1.,0.866025403784439,1.),(1.,0.866025403784439,1.,
0.866025403784439,1.,0.866025403784439,1.,0.866025403784439,1.,0.866025403784439,
1.,0.866025403784439,1.,0.866025403784439,1.,0.866025403784439,1.,0.866025403784439,
1.,0.866025403784439,1.,0.866025403784439,1.,0.866025403784439,1.,0.866025403784439,
1.,0.866025403784439,1.,0.866025403784439,1.,0.866025403784439,1.,0.866025403784439,
1.,0.866025403784439,1.,0.866025403784439,1.,0.866025403784439,1.,0.866025403784439,
1.,0.866025403784439,1.,0.866025403784439,1.,0.866025403784439,1.,0.866025403784439,
1.,0.866025403784439,1.,0.866025403784439,1.,0.866025403784439,1.,0.866025403784439,
1.,0.866025403784439,1.,0.866025403784439,1.,0.866025403784439,1.,0.866025403784439,
1.,0.866025403784439,1.,0.866025403784439,1.,0.866025403784439,1.,0.866025403784439,
1.,0.866025403784439,1.,0.866025403784439,1.,0.866025403784439,1.,0.866025403784439,
1.,0.866025403784439,1.,0.866025403784439,1.,0.866025403784439,1.,0.866025403784439,
1.,0.866025403784439,1.,0.866025403784439,1.,0.866025403784439,1.,0.866025403784439,
1.,0.866025403784439,1.,0.866025403784439,1.,0.866025403784439,1.,0.866025403784439,
1.,0.866025403784439,1.,0.866025403784439,1.,0.866025403784439,1.,0.866025403784439,
1.,0.866025403784439,1.,0.866025403784439,1.,0.866025403784439,1.,0.866025403784439,
1.,0.866025403784439,1.,0.866025403784439,1.,0.866025403784439,1.,0.866025403784439,
1.,0.866025403784439,1.,0.866025403784439,1.,0.866025403784439,1.,0.866025403784439,
1.,0.866025403784439,1.,0.866025403784439,1.,0.866025403784439,1.,0.866025403784439,
1.,0.866025403784439,1.,0.866025403784439,1.,0.866025403784439,1.,0.866025403784439,
1.,0.866025403784439,1.,0.866025403784439,1.,0.866025403784439,1.,0.866025403784439,
1.,0.866025403784439,1.,0.866025403784439,1.,0.866025403784439,1.,0.866025403784439,
1.,0.866025403784439,1.,0.866025403784439,1.,0.866025403784439,1.,0.866025403784439,
1.,0.866025403784439,1.,0.866025403784439,1.,0.866025403784439,1.,0.866025403784439,
1.,0.866025403784439,1.,0.866025403784439,1.,0.866025403784439,1.,0.866025403784439,
1.,0.866025403784439,1.,0.866025403784439,1.,0.866025403784439,1.,0.866025403784439,
1.,0.866025403784439,1.,0.866025403784439,1.,0.866025403784439,1.,0.866025403784439,
1.,0.866025403784439,1.,0.866025403784439,1.,0.866025403784439,1.,0.866025403784439,
1.,0.866025403784439,1.,0.866025403784439,1.,0.866025403784439,1.,0.866025403784439,
1.,0.866025403784439,1.,0.866025403784439,1.,0.866025403784439,1.,0.866025403784439,
1.,0.866025403784439,1.,0.866025403784439,1.,0.866025403784439,1.)))
REPRESENTATION_ITEM('')
SURFACE()
);
#429=ELLIPSE('',#18811,1.60424783344755,1.60000000000667);
#456=SHAPE_REPRESENTATION_RELATIONSHIP('SRR','None',#36712,#466);
#466=ADVANCED_BREP_SHAPE_REPRESENTATION('',(#486),#36664);
#476=STYLED_ITEM('',(#36765),#486);
#486=MANIFOLD_SOLID_BREP('Body1',#17799);
#622=CYLINDRICAL_SURFACE('',#18788,1.60000000000001);
#623=CYLINDRICAL_SURFACE('',#18790,1.60000000000001);
#624=CYLINDRICAL_SURFACE('',#18791,1.60000000000001);
#625=CYLINDRICAL_SURFACE('',#18792,1.60000000000001);
#626=CYLINDRICAL_SURFACE('',#18793,1.60000000000001);
#627=CYLINDRICAL_SURFACE('',#18794,1.60000000000001);
#628=CYLINDRICAL_SURFACE('',#18795,1.60000000000001);
#629=CYLINDRICAL_SURFACE('',#18796,1.60000000000001);
#630=CYLINDRICAL_SURFACE('',#18797,1.60000000000001);
#631=CYLINDRICAL_SURFACE('',#18798,1.60000000000001);
#632=CYLINDRICAL_SURFACE('',#18799,1.60000000000001);
#633=CYLINDRICAL_SURFACE('',#18800,1.60000000000001);
#634=CYLINDRICAL_SURFACE('',#18801,1.60000000000001);
#635=CYLINDRICAL_SURFACE('',#18802,1.60000000000001);
#636=CYLINDRICAL_SURFACE('',#18803,1.60000000000001);
#637=CYLINDRICAL_SURFACE('',#18804,1.60000000000001);
#638=CYLINDRICAL_SURFACE('',#18805,1.60000000000001);
#639=CYLINDRICAL_SURFACE('',#18806,1.60000000000001);
#640=CYLINDRICAL_SURFACE('',#18807,1.60000000000001);
#641=CYLINDRICAL_SURFACE('',#18809,1.59999999999791);
#642=CYLINDRICAL_SURFACE('',#18812,1.22111388749974);
#643=CYLINDRICAL_SURFACE('',#18813,1.22111388749974);
#644=CYLINDRICAL_SURFACE('',#18814,1.22111388749974);
#645=CYLINDRICAL_SURFACE('',#18815,1.22111388749974);
#646=CYLINDRICAL_SURFACE('',#18816,1.22111388749974);
#647=CYLINDRICAL_SURFACE('',#18817,1.22111388749974);
#648=CYLINDRICAL_SURFACE('',#18818,1.22111388749974);
#649=CYLINDRICAL_SURFACE('',#18819,1.22111388749974);
#650=CYLINDRICAL_SURFACE('',#18820,1.22111388749974);
#651=CYLINDRICAL_SURFACE('',#18821,1.22111388749974);
#652=CYLINDRICAL_SURFACE('',#18822,1.22111388749974);
#653=CYLINDRICAL_SURFACE('',#18823,1.22111388749974);
#654=CYLINDRICAL_SURFACE('',#18824,1.22111388749974);
#655=CYLINDRICAL_SURFACE('',#18825,1.22111388749974);
#656=CYLINDRICAL_SURFACE('',#18826,1.22111388749974);
#657=CYLINDRICAL_SURFACE('',#18827,1.22111388749974);
#658=CYLINDRICAL_SURFACE('',#18828,1.22111388749974);
#659=CYLINDRICAL_SURFACE('',#18829,1.22111388749974);
#660=CYLINDRICAL_SURFACE('',#18830,1.22111388749974);
#661=CYLINDRICAL_SURFACE('',#18831,1.22111388749974);
#662=CYLINDRICAL_SURFACE('',#18832,8.49999999999999);
#663=CYLINDRICAL_SURFACE('',#18834,8.49999999999999);
#664=CYLINDRICAL_SURFACE('',#18835,8.49999999999999);
#665=CYLINDRICAL_SURFACE('',#18836,7.68810118749996);
#666=CYLINDRICAL_SURFACE('',#18837,7.68810118749996);
#667=CYLINDRICAL_SURFACE('',#18838,7.68810118749996);
#668=CYLINDRICAL_SURFACE('',#18839,7.68810118749996);
#669=CYLINDRICAL_SURFACE('',#18840,7.68810118749996);
#670=CYLINDRICAL_SURFACE('',#18841,7.68810118749996);
#671=CYLINDRICAL_SURFACE('',#18842,7.68810118749996);
#672=CYLINDRICAL_SURFACE('',#18843,7.68810118749996);
#673=CYLINDRICAL_SURFACE('',#18844,8.1);
#674=CYLINDRICAL_SURFACE('',#18846,8.1);
#675=CYLINDRICAL_SURFACE('',#18847,8.1);
#676=CYLINDRICAL_SURFACE('',#18848,8.1);
#677=CYLINDRICAL_SURFACE('',#18849,8.1);
#678=CYLINDRICAL_SURFACE('',#18871,14.);
#679=CYLINDRICAL_SURFACE('',#18876,12.);
#680=CYLINDRICAL_SURFACE('',#18882,8.1);
#681=CYLINDRICAL_SURFACE('',#18892,14.);
#682=CYLINDRICAL_SURFACE('',#18894,14.);
#683=CYLINDRICAL_SURFACE('',#18896,14.);
#684=CYLINDRICAL_SURFACE('',#18904,6.00000000000001);
#685=CYLINDRICAL_SURFACE('',#18907,8.49999999999999);
#686=CYLINDRICAL_SURFACE('',#18909,7.68810118749996);
#687=CYLINDRICAL_SURFACE('',#18918,4.75);
#688=CYLINDRICAL_SURFACE('',#18921,7.00000000000001);
#689=CYLINDRICAL_SURFACE('',#18927,10.);
#690=CYLINDRICAL_SURFACE('',#18948,1.2500000000005);
#691=CYLINDRICAL_SURFACE('',#18951,1.25000000000059);
#692=CYLINDRICAL_SURFACE('',#18955,1.25000000000024);
#693=CYLINDRICAL_SURFACE('',#18959,1.24999999999999);
#694=CYLINDRICAL_SURFACE('',#18963,6.00000000000001);
#695=CYLINDRICAL_SURFACE('',#19057,8.49999999999999);
#696=CYLINDRICAL_SURFACE('',#19062,3.99999999999999);
#697=CYLINDRICAL_SURFACE('',#19065,1.22111388749974);
#698=CYLINDRICAL_SURFACE('',#19068,1.59999999999791);
#699=CYLINDRICAL_SURFACE('',#19070,1.59999999999791);
#700=CYLINDRICAL_SURFACE('',#19081,3.99999999999999);
#701=CYLINDRICAL_SURFACE('',#19084,1.60000000000001);
#927=FACE_BOUND('',#3154,.T.);
#928=FACE_BOUND('',#3168,.T.);
#929=FACE_BOUND('',#3178,.T.);
#930=FACE_BOUND('',#3180,.T.);
#931=FACE_BOUND('',#3183,.T.);
#932=FACE_BOUND('',#3284,.T.);
#933=FACE_BOUND('',#3285,.T.);
#934=FACE_BOUND('',#3286,.T.);
#935=FACE_BOUND('',#3287,.T.);
#936=FACE_BOUND('',#3288,.T.);
#937=FACE_BOUND('',#3290,.T.);
#938=FACE_BOUND('',#3293,.T.);
#939=FACE_BOUND('',#3295,.T.);
#940=FACE_BOUND('',#3310,.T.);
#941=FACE_BOUND('',#3312,.T.);
#1361=CIRCLE('',#18789,1.60000000000001);
#1362=CIRCLE('',#18808,1.60000000000001);
#1363=CIRCLE('',#18810,1.60000000000001);
#1364=CIRCLE('',#18833,8.50000000000001);
#1365=CIRCLE('',#18845,8.1);
#1366=CIRCLE('',#18851,12.);
#1367=CIRCLE('',#18856,12.);
#1368=CIRCLE('',#18861,12.);
#1369=CIRCLE('',#18866,12.);
#1370=CIRCLE('',#18867,12.);
#1371=CIRCLE('',#18872,14.);
#1372=CIRCLE('',#18873,14.);
#1373=CIRCLE('',#18875,12.);
#1374=CIRCLE('',#18877,12.);
#1375=CIRCLE('',#18878,12.);
#1376=CIRCLE('',#18879,12.);
#1377=CIRCLE('',#18880,12.);
#1378=CIRCLE('',#18883,8.1);
#1379=CIRCLE('',#18884,8.1);
#1380=CIRCLE('',#18886,11.2187458390495);
#1381=CIRCLE('',#18887,4.22441061393973);
#1382=CIRCLE('',#18889,14.);
#1383=CIRCLE('',#18890,14.);
#1384=CIRCLE('',#18891,14.);
#1385=CIRCLE('',#18893,14.);
#1386=CIRCLE('',#18895,14.);
#1387=CIRCLE('',#18897,14.);
#1388=CIRCLE('',#18903,6.29999999999999);
#1389=CIRCLE('',#18905,6.00000000000001);
#1390=CIRCLE('',#18906,6.00000000000001);
#1391=CIRCLE('',#18908,8.49999999999999);
#1392=CIRCLE('',#18912,0.3);
#1393=CIRCLE('',#18914,9.7);
#1394=CIRCLE('',#18915,0.3);
#1395=CIRCLE('',#18916,10.);
#1396=CIRCLE('',#18917,10.);
#1397=CIRCLE('',#18919,4.75);
#1398=CIRCLE('',#18920,4.75);
#1399=CIRCLE('',#18922,7.00000000000001);
#1400=CIRCLE('',#18923,7.00000000000001);
#1401=CIRCLE('',#18926,6.00000000000001);
#1402=CIRCLE('',#18928,10.);
#1403=CIRCLE('',#18929,10.);
#1404=CIRCLE('',#18930,10.);
#1405=CIRCLE('',#18931,10.);
#1406=CIRCLE('',#18932,10.);
#1407=CIRCLE('',#18933,10.);
#1408=CIRCLE('',#18934,10.);
#1409=CIRCLE('',#18935,10.);
#1410=CIRCLE('',#18936,10.);
#1411=CIRCLE('',#18938,8.49999999999999);
#1412=CIRCLE('',#18940,1.2500000000005);
#1413=CIRCLE('',#18941,1.2500000000005);
#1414=CIRCLE('',#18943,1.25000000000059);
#1415=CIRCLE('',#18945,1.25000000000024);
#1416=CIRCLE('',#18947,1.24999999999999);
#1417=CIRCLE('',#18949,1.2500000000005);
#1418=CIRCLE('',#18950,1.2500000000005);
#1419=CIRCLE('',#18952,1.25000000000059);
#1420=CIRCLE('',#18953,1.25000000000059);
#1421=CIRCLE('',#18954,1.25000000000059);
#1422=CIRCLE('',#18956,1.25000000000024);
#1423=CIRCLE('',#18957,1.25000000000024);
#1424=CIRCLE('',#18958,1.25000000000024);
#1425=CIRCLE('',#18960,1.24999999999999);
#1426=CIRCLE('',#18961,1.24999999999999);
#1427=CIRCLE('',#18962,1.24999999999999);
#1428=CIRCLE('',#18964,6.00000000000001);
#1429=CIRCLE('',#19059,4.);
#1430=CIRCLE('',#19061,4.);
#1431=CIRCLE('',#19063,3.99999999999999);
#1432=CIRCLE('',#19064,3.99999999999999);
#1433=CIRCLE('',#19069,1.60000000000001);
#1434=CIRCLE('',#19071,1.60000000000001);
#1435=CIRCLE('',#19073,2.);
#1436=CIRCLE('',#19075,2.);
#1437=CIRCLE('',#19077,3.6);
#1438=CIRCLE('',#19079,3.99999999999999);
#1439=CIRCLE('',#19080,3.6);
#1996=FACE_OUTER_BOUND('',#3078,.T.);
#1997=FACE_OUTER_BOUND('',#3079,.T.);
#1998=FACE_OUTER_BOUND('',#3080,.T.);
#1999=FACE_OUTER_BOUND('',#3081,.T.);
#2000=FACE_OUTER_BOUND('',#3082,.T.);
#2001=FACE_OUTER_BOUND('',#3083,.T.);
#2002=FACE_OUTER_BOUND('',#3084,.T.);
#2003=FACE_OUTER_BOUND('',#3085,.T.);
#2004=FACE_OUTER_BOUND('',#3086,.T.);
#2005=FACE_OUTER_BOUND('',#3087,.T.);
#2006=FACE_OUTER_BOUND('',#3088,.T.);
#2007=FACE_OUTER_BOUND('',#3089,.T.);
#2008=FACE_OUTER_BOUND('',#3090,.T.);
#2009=FACE_OUTER_BOUND('',#3091,.T.);
#2010=FACE_OUTER_BOUND('',#3092,.T.);
#2011=FACE_OUTER_BOUND('',#3093,.T.);
#2012=FACE_OUTER_BOUND('',#3094,.T.);
#2013=FACE_OUTER_BOUND('',#3095,.T.);
#2014=FACE_OUTER_BOUND('',#3096,.T.);
#2015=FACE_OUTER_BOUND('',#3097,.T.);
#2016=FACE_OUTER_BOUND('',#3098,.T.);
#2017=FACE_OUTER_BOUND('',#3099,.T.);
#2018=FACE_OUTER_BOUND('',#3100,.T.);
#2019=FACE_OUTER_BOUND('',#3101,.T.);
#2020=FACE_OUTER_BOUND('',#3102,.T.);
#2021=FACE_OUTER_BOUND('',#3103,.T.);
#2022=FACE_OUTER_BOUND('',#3104,.T.);
#2023=FACE_OUTER_BOUND('',#3105,.T.);
#2024=FACE_OUTER_BOUND('',#3106,.T.);
#2025=FACE_OUTER_BOUND('',#3107,.T.);
#2026=FACE_OUTER_BOUND('',#3108,.T.);
#2027=FACE_OUTER_BOUND('',#3109,.T.);
#2028=FACE_OUTER_BOUND('',#3110,.T.);
#2029=FACE_OUTER_BOUND('',#3111,.T.);
#2030=FACE_OUTER_BOUND('',#3112,.T.);
#2031=FACE_OUTER_BOUND('',#3113,.T.);
#2032=FACE_OUTER_BOUND('',#3114,.T.);
#2033=FACE_OUTER_BOUND('',#3115,.T.);
#2034=FACE_OUTER_BOUND('',#3116,.T.);
#2035=FACE_OUTER_BOUND('',#3117,.T.);
#2036=FACE_OUTER_BOUND('',#3118,.T.);
#2037=FACE_OUTER_BOUND('',#3119,.T.);
#2038=FACE_OUTER_BOUND('',#3120,.T.);
#2039=FACE_OUTER_BOUND('',#3121,.T.);
#2040=FACE_OUTER_BOUND('',#3122,.T.);
#2041=FACE_OUTER_BOUND('',#3123,.T.);
#2042=FACE_OUTER_BOUND('',#3124,.T.);
#2043=FACE_OUTER_BOUND('',#3125,.T.);
#2044=FACE_OUTER_BOUND('',#3126,.T.);
#2045=FACE_OUTER_BOUND('',#3127,.T.);
#2046=FACE_OUTER_BOUND('',#3128,.T.);
#2047=FACE_OUTER_BOUND('',#3129,.T.);
#2048=FACE_OUTER_BOUND('',#3130,.T.);
#2049=FACE_OUTER_BOUND('',#3131,.T.);
#2050=FACE_OUTER_BOUND('',#3132,.T.);
#2051=FACE_OUTER_BOUND('',#3133,.T.);
#2052=FACE_OUTER_BOUND('',#3134,.T.);
#2053=FACE_OUTER_BOUND('',#3135,.T.);
#2054=FACE_OUTER_BOUND('',#3136,.T.);
#2055=FACE_OUTER_BOUND('',#3137,.T.);
#2056=FACE_OUTER_BOUND('',#3138,.T.);
#2057=FACE_OUTER_BOUND('',#3139,.T.);
#2058=FACE_OUTER_BOUND('',#3140,.T.);
#2059=FACE_OUTER_BOUND('',#3141,.T.);
#2060=FACE_OUTER_BOUND('',#3142,.T.);
#2061=FACE_OUTER_BOUND('',#3143,.T.);
#2062=FACE_OUTER_BOUND('',#3144,.T.);
#2063=FACE_OUTER_BOUND('',#3145,.T.);
#2064=FACE_OUTER_BOUND('',#3146,.T.);
#2065=FACE_OUTER_BOUND('',#3147,.T.);
#2066=FACE_OUTER_BOUND('',#3148,.T.);
#2067=FACE_OUTER_BOUND('',#3149,.T.);
#2068=FACE_OUTER_BOUND('',#3150,.T.);
#2069=FACE_OUTER_BOUND('',#3151,.T.);
#2070=FACE_OUTER_BOUND('',#3152,.T.);
#2071=FACE_OUTER_BOUND('',#3153,.T.);
#2072=FACE_OUTER_BOUND('',#3155,.T.);
#2073=FACE_OUTER_BOUND('',#3156,.T.);
#2074=FACE_OUTER_BOUND('',#3157,.T.);
#2075=FACE_OUTER_BOUND('',#3158,.T.);
#2076=FACE_OUTER_BOUND('',#3159,.T.);
#2077=FACE_OUTER_BOUND('',#3160,.T.);
#2078=FACE_OUTER_BOUND('',#3161,.T.);
#2079=FACE_OUTER_BOUND('',#3162,.T.);
#2080=FACE_OUTER_BOUND('',#3163,.T.);
#2081=FACE_OUTER_BOUND('',#3164,.T.);
#2082=FACE_OUTER_BOUND('',#3165,.T.);
#2083=FACE_OUTER_BOUND('',#3166,.T.);
#2084=FACE_OUTER_BOUND('',#3167,.T.);
#2085=FACE_OUTER_BOUND('',#3169,.T.);
#2086=FACE_OUTER_BOUND('',#3170,.T.);
#2087=FACE_OUTER_BOUND('',#3171,.T.);
#2088=FACE_OUTER_BOUND('',#3172,.T.);
#2089=FACE_OUTER_BOUND('',#3173,.T.);
#2090=FACE_OUTER_BOUND('',#3174,.T.);
#2091=FACE_OUTER_BOUND('',#3175,.T.);
#2092=FACE_OUTER_BOUND('',#3176,.T.);
#2093=FACE_OUTER_BOUND('',#3177,.T.);
#2094=FACE_OUTER_BOUND('',#3179,.T.);
#2095=FACE_OUTER_BOUND('',#3181,.T.);
#2096=FACE_OUTER_BOUND('',#3182,.T.);
#2097=FACE_OUTER_BOUND('',#3184,.T.);
#2098=FACE_OUTER_BOUND('',#3185,.T.);
#2099=FACE_OUTER_BOUND('',#3186,.T.);
#2100=FACE_OUTER_BOUND('',#3187,.T.);
#2101=FACE_OUTER_BOUND('',#3188,.T.);
#2102=FACE_OUTER_BOUND('',#3189,.T.);
#2103=FACE_OUTER_BOUND('',#3190,.T.);
#2104=FACE_OUTER_BOUND('',#3191,.T.);
#2105=FACE_OUTER_BOUND('',#3192,.T.);
#2106=FACE_OUTER_BOUND('',#3193,.T.);
#2107=FACE_OUTER_BOUND('',#3194,.T.);
#2108=FACE_OUTER_BOUND('',#3195,.T.);
#2109=FACE_OUTER_BOUND('',#3196,.T.);
#2110=FACE_OUTER_BOUND('',#3197,.T.);
#2111=FACE_OUTER_BOUND('',#3198,.T.);
#2112=FACE_OUTER_BOUND('',#3199,.T.);
#2113=FACE_OUTER_BOUND('',#3200,.T.);
#2114=FACE_OUTER_BOUND('',#3201,.T.);
#2115=FACE_OUTER_BOUND('',#3202,.T.);
#2116=FACE_OUTER_BOUND('',#3203,.T.);
#2117=FACE_OUTER_BOUND('',#3204,.T.);
#2118=FACE_OUTER_BOUND('',#3205,.T.);
#2119=FACE_OUTER_BOUND('',#3206,.T.);
#2120=FACE_OUTER_BOUND('',#3207,.T.);
#2121=FACE_OUTER_BOUND('',#3208,.T.);
#2122=FACE_OUTER_BOUND('',#3209,.T.);
#2123=FACE_OUTER_BOUND('',#3210,.T.);
#2124=FACE_OUTER_BOUND('',#3211,.T.);
#2125=FACE_OUTER_BOUND('',#3212,.T.);
#2126=FACE_OUTER_BOUND('',#3213,.T.);
#2127=FACE_OUTER_BOUND('',#3214,.T.);
#2128=FACE_OUTER_BOUND('',#3215,.T.);
#2129=FACE_OUTER_BOUND('',#3216,.T.);
#2130=FACE_OUTER_BOUND('',#3217,.T.);
#2131=FACE_OUTER_BOUND('',#3218,.T.);
#2132=FACE_OUTER_BOUND('',#3219,.T.);
#2133=FACE_OUTER_BOUND('',#3220,.T.);
#2134=FACE_OUTER_BOUND('',#3221,.T.);
#2135=FACE_OUTER_BOUND('',#3222,.T.);
#2136=FACE_OUTER_BOUND('',#3223,.T.);
#2137=FACE_OUTER_BOUND('',#3224,.T.);
#2138=FACE_OUTER_BOUND('',#3225,.T.);
#2139=FACE_OUTER_BOUND('',#3226,.T.);
#2140=FACE_OUTER_BOUND('',#3227,.T.);
#2141=FACE_OUTER_BOUND('',#3228,.T.);
#2142=FACE_OUTER_BOUND('',#3229,.T.);
#2143=FACE_OUTER_BOUND('',#3230,.T.);
#2144=FACE_OUTER_BOUND('',#3231,.T.);
#2145=FACE_OUTER_BOUND('',#3232,.T.);
#2146=FACE_OUTER_BOUND('',#3233,.T.);
#2147=FACE_OUTER_BOUND('',#3234,.T.);
#2148=FACE_OUTER_BOUND('',#3235,.T.);
#2149=FACE_OUTER_BOUND('',#3236,.T.);
#2150=FACE_OUTER_BOUND('',#3237,.T.);
#2151=FACE_OUTER_BOUND('',#3238,.T.);
#2152=FACE_OUTER_BOUND('',#3239,.T.);
#2153=FACE_OUTER_BOUND('',#3240,.T.);
#2154=FACE_OUTER_BOUND('',#3241,.T.);
#2155=FACE_OUTER_BOUND('',#3242,.T.);
#2156=FACE_OUTER_BOUND('',#3243,.T.);
#2157=FACE_OUTER_BOUND('',#3244,.T.);
#2158=FACE_OUTER_BOUND('',#3245,.T.);
#2159=FACE_OUTER_BOUND('',#3246,.T.);
#2160=FACE_OUTER_BOUND('',#3247,.T.);
#2161=FACE_OUTER_BOUND('',#3248,.T.);
#2162=FACE_OUTER_BOUND('',#3249,.T.);
#2163=FACE_OUTER_BOUND('',#3250,.T.);
#2164=FACE_OUTER_BOUND('',#3251,.T.);
#2165=FACE_OUTER_BOUND('',#3252,.T.);
#2166=FACE_OUTER_BOUND('',#3253,.T.);
#2167=FACE_OUTER_BOUND('',#3254,.T.);
#2168=FACE_OUTER_BOUND('',#3255,.T.);
#2169=FACE_OUTER_BOUND('',#3256,.T.);
#2170=FACE_OUTER_BOUND('',#3257,.T.);
#2171=FACE_OUTER_BOUND('',#3258,.T.);
#2172=FACE_OUTER_BOUND('',#3259,.T.);
#2173=FACE_OUTER_BOUND('',#3260,.T.);
#2174=FACE_OUTER_BOUND('',#3261,.T.);
#2175=FACE_OUTER_BOUND('',#3262,.T.);
#2176=FACE_OUTER_BOUND('',#3263,.T.);
#2177=FACE_OUTER_BOUND('',#3264,.T.);
#2178=FACE_OUTER_BOUND('',#3265,.T.);
#2179=FACE_OUTER_BOUND('',#3266,.T.);
#2180=FACE_OUTER_BOUND('',#3267,.T.);
#2181=FACE_OUTER_BOUND('',#3268,.T.);
#2182=FACE_OUTER_BOUND('',#3269,.T.);
#2183=FACE_OUTER_BOUND('',#3270,.T.);
#2184=FACE_OUTER_BOUND('',#3271,.T.);
#2185=FACE_OUTER_BOUND('',#3272,.T.);
#2186=FACE_OUTER_BOUND('',#3273,.T.);
#2187=FACE_OUTER_BOUND('',#3274,.T.);
#2188=FACE_OUTER_BOUND('',#3275,.T.);
#2189=FACE_OUTER_BOUND('',#3276,.T.);
#2190=FACE_OUTER_BOUND('',#3277,.T.);
#2191=FACE_OUTER_BOUND('',#3278,.T.);
#2192=FACE_OUTER_BOUND('',#3279,.T.);
#2193=FACE_OUTER_BOUND('',#3280,.T.);
#2194=FACE_OUTER_BOUND('',#3281,.T.);
#2195=FACE_OUTER_BOUND('',#3282,.T.);
#2196=FACE_OUTER_BOUND('',#3283,.T.);
#2197=FACE_OUTER_BOUND('',#3289,.T.);
#2198=FACE_OUTER_BOUND('',#3291,.T.);
#2199=FACE_OUTER_BOUND('',#3292,.T.);
#2200=FACE_OUTER_BOUND('',#3294,.T.);
#2201=FACE_OUTER_BOUND('',#3296,.T.);
#2202=FACE_OUTER_BOUND('',#3297,.T.);
#2203=FACE_OUTER_BOUND('',#3298,.T.);
#2204=FACE_OUTER_BOUND('',#3299,.T.);
#2205=FACE_OUTER_BOUND('',#3300,.T.);
#2206=FACE_OUTER_BOUND('',#3301,.T.);
#2207=FACE_OUTER_BOUND('',#3302,.T.);
#2208=FACE_OUTER_BOUND('',#3303,.T.);
#2209=FACE_OUTER_BOUND('',#3304,.T.);
#2210=FACE_OUTER_BOUND('',#3305,.T.);
#2211=FACE_OUTER_BOUND('',#3306,.T.);
#2212=FACE_OUTER_BOUND('',#3307,.T.);
#2213=FACE_OUTER_BOUND('',#3308,.T.);
#2214=FACE_OUTER_BOUND('',#3309,.T.);
#2215=FACE_OUTER_BOUND('',#3311,.T.);
#2216=FACE_OUTER_BOUND('',#3313,.T.);
#3078=EDGE_LOOP('',(#13840,#13841,#13842,#13843));
#3079=EDGE_LOOP('',(#13844,#13845,#13846,#13847));
#3080=EDGE_LOOP('',(#13848,#13849,#13850,#13851));
#3081=EDGE_LOOP('',(#13852,#13853,#13854,#13855));
#3082=EDGE_LOOP('',(#13856,#13857,#13858,#13859));
#3083=EDGE_LOOP('',(#13860,#13861,#13862,#13863));
#3084=EDGE_LOOP('',(#13864,#13865,#13866,#13867));
#3085=EDGE_LOOP('',(#13868,#13869,#13870,#13871));
#3086=EDGE_LOOP('',(#13872,#13873,#13874,#13875));
#3087=EDGE_LOOP('',(#13876,#13877,#13878,#13879));
#3088=EDGE_LOOP('',(#13880,#13881,#13882,#13883));
#3089=EDGE_LOOP('',(#13884,#13885,#13886,#13887));
#3090=EDGE_LOOP('',(#13888,#13889,#13890,#13891));
#3091=EDGE_LOOP('',(#13892,#13893,#13894,#13895));
#3092=EDGE_LOOP('',(#13896,#13897,#13898,#13899));
#3093=EDGE_LOOP('',(#13900,#13901,#13902,#13903));
#3094=EDGE_LOOP('',(#13904,#13905,#13906,#13907));
#3095=EDGE_LOOP('',(#13908,#13909,#13910,#13911));
#3096=EDGE_LOOP('',(#13912,#13913,#13914,#13915));
#3097=EDGE_LOOP('',(#13916,#13917,#13918,#13919,#13920));
#3098=EDGE_LOOP('',(#13921,#13922,#13923,#13924));
#3099=EDGE_LOOP('',(#13925,#13926,#13927,#13928));
#3100=EDGE_LOOP('',(#13929,#13930,#13931,#13932));
#3101=EDGE_LOOP('',(#13933,#13934,#13935,#13936));
#3102=EDGE_LOOP('',(#13937,#13938,#13939,#13940));
#3103=EDGE_LOOP('',(#13941,#13942,#13943,#13944));
#3104=EDGE_LOOP('',(#13945,#13946,#13947,#13948));
#3105=EDGE_LOOP('',(#13949,#13950,#13951,#13952));
#3106=EDGE_LOOP('',(#13953,#13954,#13955,#13956));
#3107=EDGE_LOOP('',(#13957,#13958,#13959,#13960));
#3108=EDGE_LOOP('',(#13961,#13962,#13963,#13964));
#3109=EDGE_LOOP('',(#13965,#13966,#13967,#13968));
#3110=EDGE_LOOP('',(#13969,#13970,#13971,#13972));
#3111=EDGE_LOOP('',(#13973,#13974,#13975,#13976));
#3112=EDGE_LOOP('',(#13977,#13978,#13979,#13980));
#3113=EDGE_LOOP('',(#13981,#13982,#13983,#13984));
#3114=EDGE_LOOP('',(#13985,#13986,#13987,#13988));
#3115=EDGE_LOOP('',(#13989,#13990,#13991,#13992));
#3116=EDGE_LOOP('',(#13993,#13994,#13995,#13996));
#3117=EDGE_LOOP('',(#13997,#13998,#13999,#14000));
#3118=EDGE_LOOP('',(#14001,#14002,#14003,#14004));
#3119=EDGE_LOOP('',(#14005,#14006,#14007,#14008));
#3120=EDGE_LOOP('',(#14009,#14010,#14011,#14012));
#3121=EDGE_LOOP('',(#14013,#14014,#14015,#14016));
#3122=EDGE_LOOP('',(#14017,#14018,#14019,#14020));
#3123=EDGE_LOOP('',(#14021,#14022,#14023,#14024));
#3124=EDGE_LOOP('',(#14025,#14026,#14027,#14028));
#3125=EDGE_LOOP('',(#14029,#14030,#14031,#14032));
#3126=EDGE_LOOP('',(#14033,#14034,#14035,#14036));
#3127=EDGE_LOOP('',(#14037,#14038,#14039,#14040));
#3128=EDGE_LOOP('',(#14041,#14042,#14043,#14044));
#3129=EDGE_LOOP('',(#14045,#14046,#14047,#14048));
#3130=EDGE_LOOP('',(#14049,#14050,#14051,#14052));
#3131=EDGE_LOOP('',(#14053,#14054,#14055,#14056));
#3132=EDGE_LOOP('',(#14057,#14058,#14059,#14060));
#3133=EDGE_LOOP('',(#14061,#14062,#14063,#14064));
#3134=EDGE_LOOP('',(#14065,#14066,#14067,#14068));
#3135=EDGE_LOOP('',(#14069,#14070,#14071,#14072));
#3136=EDGE_LOOP('',(#14073,#14074,#14075,#14076,#14077));
#3137=EDGE_LOOP('',(#14078,#14079,#14080,#14081,#14082));
#3138=EDGE_LOOP('',(#14083,#14084,#14085,#14086));
#3139=EDGE_LOOP('',(#14087,#14088,#14089,#14090,#14091));
#3140=EDGE_LOOP('',(#14092,#14093,#14094,#14095));
#3141=EDGE_LOOP('',(#14096,#14097,#14098,#14099,#14100));
#3142=EDGE_LOOP('',(#14101,#14102,#14103,#14104));
#3143=EDGE_LOOP('',(#14105,#14106,#14107,#14108,#14109));
#3144=EDGE_LOOP('',(#14110,#14111,#14112,#14113));
#3145=EDGE_LOOP('',(#14114,#14115,#14116,#14117,#14118));
#3146=EDGE_LOOP('',(#14119,#14120,#14121,#14122,#14123));
#3147=EDGE_LOOP('',(#14124,#14125,#14126,#14127,#14128));
#3148=EDGE_LOOP('',(#14129,#14130,#14131,#14132,#14133));
#3149=EDGE_LOOP('',(#14134,#14135,#14136,#14137,#14138));
#3150=EDGE_LOOP('',(#14139,#14140,#14141,#14142));
#3151=EDGE_LOOP('',(#14143,#14144,#14145,#14146));
#3152=EDGE_LOOP('',(#14147,#14148,#14149,#14150,#14151,#14152,#14153,#14154,
#14155,#14156,#14157,#14158));
#3153=EDGE_LOOP('',(#14159));
#3154=EDGE_LOOP('',(#14160,#14161,#14162,#14163));
#3155=EDGE_LOOP('',(#14164,#14165,#14166,#14167));
#3156=EDGE_LOOP('',(#14168,#14169,#14170,#14171));
#3157=EDGE_LOOP('',(#14172,#14173,#14174,#14175,#14176,#14177,#14178,#14179,
#14180,#14181,#14182,#14183,#14184,#14185,#14186,#14187,#14188,#14189,#14190,
#14191));
#3158=EDGE_LOOP('',(#14192,#14193,#14194,#14195));
#3159=EDGE_LOOP('',(#14196,#14197,#14198,#14199));
#3160=EDGE_LOOP('',(#14200,#14201,#14202,#14203));
#3161=EDGE_LOOP('',(#14204,#14205,#14206,#14207));
#3162=EDGE_LOOP('',(#14208,#14209,#14210,#14211));
#3163=EDGE_LOOP('',(#14212,#14213,#14214,#14215));
#3164=EDGE_LOOP('',(#14216,#14217,#14218,#14219,#14220,#14221,#14222,#14223,
#14224,#14225,#14226,#14227,#14228,#14229,#14230,#14231,#14232,#14233,#14234,
#14235,#14236,#14237));
#3165=EDGE_LOOP('',(#14238,#14239,#14240,#14241,#14242,#14243,#14244,#14245,
#14246,#14247,#14248,#14249,#14250,#14251,#14252,#14253,#14254,#14255,#14256,
#14257,#14258));
#3166=EDGE_LOOP('',(#14259,#14260,#14261,#14262));
#3167=EDGE_LOOP('',(#14263));
#3168=EDGE_LOOP('',(#14264));
#3169=EDGE_LOOP('',(#14265,#14266,#14267,#14268));
#3170=EDGE_LOOP('',(#14269,#14270,#14271));
#3171=EDGE_LOOP('',(#14272,#14273,#14274,#14275));
#3172=EDGE_LOOP('',(#14276,#14277,#14278,#14279));
#3173=EDGE_LOOP('',(#14280,#14281,#14282,#14283));
#3174=EDGE_LOOP('',(#14284,#14285,#14286,#14287,#14288));
#3175=EDGE_LOOP('',(#14289,#14290,#14291,#14292));
#3176=EDGE_LOOP('',(#14293,#14294,#14295,#14296));
#3177=EDGE_LOOP('',(#14297));
#3178=EDGE_LOOP('',(#14298));
#3179=EDGE_LOOP('',(#14299));
#3180=EDGE_LOOP('',(#14300));
#3181=EDGE_LOOP('',(#14301,#14302,#14303,#14304,#14305,#14306,#14307,#14308,
#14309,#14310,#14311,#14312,#14313));
#3182=EDGE_LOOP('',(#14314));
#3183=EDGE_LOOP('',(#14315,#14316));
#3184=EDGE_LOOP('',(#14317,#14318,#14319,#14320));
#3185=EDGE_LOOP('',(#14321,#14322));
#3186=EDGE_LOOP('',(#14323,#14324));
#3187=EDGE_LOOP('',(#14325,#14326));
#3188=EDGE_LOOP('',(#14327,#14328,#14329,#14330,#14331,#14332));
#3189=EDGE_LOOP('',(#14333,#14334,#14335,#14336,#14337,#14338));
#3190=EDGE_LOOP('',(#14339,#14340,#14341,#14342,#14343,#14344));
#3191=EDGE_LOOP('',(#14345,#14346,#14347,#14348,#14349,#14350));
#3192=EDGE_LOOP('',(#14351,#14352,#14353,#14354));
#3193=EDGE_LOOP('',(#14355,#14356,#14357,#14358));
#3194=EDGE_LOOP('',(#14359,#14360,#14361,#14362));
#3195=EDGE_LOOP('',(#14363,#14364,#14365,#14366));
#3196=EDGE_LOOP('',(#14367,#14368,#14369,#14370));
#3197=EDGE_LOOP('',(#14371,#14372,#14373,#14374));
#3198=EDGE_LOOP('',(#14375,#14376,#14377,#14378));
#3199=EDGE_LOOP('',(#14379,#14380,#14381,#14382));
#3200=EDGE_LOOP('',(#14383,#14384,#14385,#14386));
#3201=EDGE_LOOP('',(#14387,#14388,#14389,#14390));
#3202=EDGE_LOOP('',(#14391,#14392,#14393,#14394));
#3203=EDGE_LOOP('',(#14395,#14396,#14397,#14398));
#3204=EDGE_LOOP('',(#14399,#14400,#14401,#14402));
#3205=EDGE_LOOP('',(#14403,#14404,#14405,#14406));
#3206=EDGE_LOOP('',(#14407,#14408,#14409,#14410));
#3207=EDGE_LOOP('',(#14411,#14412,#14413,#14414));
#3208=EDGE_LOOP('',(#14415,#14416,#14417,#14418));
#3209=EDGE_LOOP('',(#14419,#14420,#14421,#14422));
#3210=EDGE_LOOP('',(#14423,#14424,#14425,#14426));
#3211=EDGE_LOOP('',(#14427,#14428,#14429,#14430));
#3212=EDGE_LOOP('',(#14431,#14432,#14433,#14434));
#3213=EDGE_LOOP('',(#14435,#14436,#14437,#14438));
#3214=EDGE_LOOP('',(#14439,#14440,#14441,#14442));
#3215=EDGE_LOOP('',(#14443,#14444,#14445,#14446));
#3216=EDGE_LOOP('',(#14447,#14448,#14449,#14450));
#3217=EDGE_LOOP('',(#14451,#14452,#14453,#14454));
#3218=EDGE_LOOP('',(#14455,#14456,#14457,#14458));
#3219=EDGE_LOOP('',(#14459,#14460,#14461,#14462));
#3220=EDGE_LOOP('',(#14463,#14464,#14465,#14466));
#3221=EDGE_LOOP('',(#14467,#14468,#14469,#14470));
#3222=EDGE_LOOP('',(#14471,#14472,#14473,#14474));
#3223=EDGE_LOOP('',(#14475,#14476,#14477,#14478));
#3224=EDGE_LOOP('',(#14479,#14480,#14481,#14482));
#3225=EDGE_LOOP('',(#14483,#14484,#14485,#14486));
#3226=EDGE_LOOP('',(#14487,#14488,#14489,#14490));
#3227=EDGE_LOOP('',(#14491,#14492,#14493,#14494));
#3228=EDGE_LOOP('',(#14495,#14496,#14497,#14498));
#3229=EDGE_LOOP('',(#14499,#14500,#14501,#14502));
#3230=EDGE_LOOP('',(#14503,#14504,#14505,#14506));
#3231=EDGE_LOOP('',(#14507,#14508,#14509,#14510));
#3232=EDGE_LOOP('',(#14511,#14512,#14513,#14514));
#3233=EDGE_LOOP('',(#14515,#14516,#14517,#14518));
#3234=EDGE_LOOP('',(#14519,#14520,#14521,#14522));
#3235=EDGE_LOOP('',(#14523,#14524,#14525,#14526));
#3236=EDGE_LOOP('',(#14527,#14528,#14529,#14530));
#3237=EDGE_LOOP('',(#14531,#14532,#14533,#14534));
#3238=EDGE_LOOP('',(#14535,#14536,#14537,#14538));
#3239=EDGE_LOOP('',(#14539,#14540,#14541,#14542));
#3240=EDGE_LOOP('',(#14543,#14544,#14545,#14546));
#3241=EDGE_LOOP('',(#14547,#14548,#14549,#14550));
#3242=EDGE_LOOP('',(#14551,#14552,#14553,#14554));
#3243=EDGE_LOOP('',(#14555,#14556,#14557,#14558));
#3244=EDGE_LOOP('',(#14559,#14560,#14561,#14562));
#3245=EDGE_LOOP('',(#14563,#14564,#14565,#14566));
#3246=EDGE_LOOP('',(#14567,#14568,#14569,#14570));
#3247=EDGE_LOOP('',(#14571,#14572,#14573,#14574));
#3248=EDGE_LOOP('',(#14575,#14576,#14577,#14578));
#3249=EDGE_LOOP('',(#14579,#14580,#14581,#14582));
#3250=EDGE_LOOP('',(#14583,#14584,#14585,#14586));
#3251=EDGE_LOOP('',(#14587,#14588,#14589,#14590));
#3252=EDGE_LOOP('',(#14591,#14592,#14593,#14594));
#3253=EDGE_LOOP('',(#14595,#14596,#14597,#14598));
#3254=EDGE_LOOP('',(#14599,#14600,#14601,#14602));
#3255=EDGE_LOOP('',(#14603,#14604,#14605,#14606));
#3256=EDGE_LOOP('',(#14607,#14608,#14609,#14610));
#3257=EDGE_LOOP('',(#14611,#14612,#14613,#14614));
#3258=EDGE_LOOP('',(#14615,#14616,#14617,#14618));
#3259=EDGE_LOOP('',(#14619,#14620,#14621,#14622));
#3260=EDGE_LOOP('',(#14623,#14624,#14625,#14626));
#3261=EDGE_LOOP('',(#14627,#14628,#14629,#14630));
#3262=EDGE_LOOP('',(#14631,#14632,#14633,#14634));
#3263=EDGE_LOOP('',(#14635,#14636,#14637,#14638));
#3264=EDGE_LOOP('',(#14639,#14640,#14641,#14642));
#3265=EDGE_LOOP('',(#14643,#14644,#14645,#14646));
#3266=EDGE_LOOP('',(#14647,#14648,#14649,#14650));
#3267=EDGE_LOOP('',(#14651,#14652,#14653,#14654));
#3268=EDGE_LOOP('',(#14655,#14656,#14657,#14658));
#3269=EDGE_LOOP('',(#14659,#14660,#14661,#14662));
#3270=EDGE_LOOP('',(#14663,#14664,#14665,#14666));
#3271=EDGE_LOOP('',(#14667,#14668,#14669,#14670));
#3272=EDGE_LOOP('',(#14671,#14672,#14673,#14674));
#3273=EDGE_LOOP('',(#14675,#14676,#14677,#14678));
#3274=EDGE_LOOP('',(#14679,#14680,#14681,#14682));
#3275=EDGE_LOOP('',(#14683,#14684,#14685,#14686));
#3276=EDGE_LOOP('',(#14687,#14688,#14689,#14690));
#3277=EDGE_LOOP('',(#14691,#14692,#14693,#14694));
#3278=EDGE_LOOP('',(#14695,#14696,#14697,#14698));
#3279=EDGE_LOOP('',(#14699,#14700,#14701,#14702));
#3280=EDGE_LOOP('',(#14703,#14704,#14705,#14706));
#3281=EDGE_LOOP('',(#14707,#14708,#14709,#14710));
#3282=EDGE_LOOP('',(#14711,#14712,#14713,#14714));
#3283=EDGE_LOOP('',(#14715,#14716,#14717,#14718,#14719,#14720,#14721,#14722,
#14723,#14724,#14725,#14726,#14727,#14728,#14729,#14730,#14731,#14732,#14733,
#14734,#14735,#14736,#14737,#14738,#14739,#14740,#14741,#14742,#14743,#14744,
#14745,#14746,#14747,#14748,#14749,#14750,#14751,#14752,#14753,#14754,#14755,
#14756,#14757,#14758,#14759,#14760,#14761,#14762,#14763,#14764,#14765,#14766,
#14767,#14768,#14769,#14770,#14771,#14772,#14773,#14774,#14775,#14776,#14777,
#14778,#14779,#14780,#14781,#14782,#14783,#14784,#14785,#14786,#14787,#14788,
#14789,#14790,#14791,#14792,#14793,#14794,#14795,#14796,#14797,#14798,#14799,
#14800,#14801,#14802,#14803,#14804));
#3284=EDGE_LOOP('',(#14805));
#3285=EDGE_LOOP('',(#14806));
#3286=EDGE_LOOP('',(#14807));
#3287=EDGE_LOOP('',(#14808));
#3288=EDGE_LOOP('',(#14809));
#3289=EDGE_LOOP('',(#14810,#14811,#14812,#14813,#14814,#14815,#14816,#14817,
#14818,#14819,#14820,#14821,#14822,#14823,#14824,#14825,#14826,#14827,#14828,
#14829,#14830,#14831,#14832,#14833,#14834,#14835,#14836,#14837,#14838,#14839,
#14840,#14841,#14842,#14843,#14844,#14845,#14846,#14847,#14848,#14849,#14850,
#14851,#14852,#14853,#14854,#14855,#14856,#14857,#14858,#14859,#14860,#14861,
#14862,#14863,#14864,#14865,#14866,#14867,#14868,#14869,#14870,#14871,#14872,
#14873,#14874,#14875,#14876,#14877,#14878,#14879,#14880,#14881,#14882,#14883,
#14884,#14885,#14886,#14887,#14888,#14889,#14890,#14891,#14892,#14893,#14894,
#14895,#14896,#14897,#14898,#14899));
#3290=EDGE_LOOP('',(#14900,#14901,#14902,#14903,#14904,#14905,#14906,#14907,
#14908,#14909,#14910));
#3291=EDGE_LOOP('',(#14911,#14912,#14913,#14914));
#3292=EDGE_LOOP('',(#14915));
#3293=EDGE_LOOP('',(#14916));
#3294=EDGE_LOOP('',(#14917));
#3295=EDGE_LOOP('',(#14918));
#3296=EDGE_LOOP('',(#14919,#14920,#14921,#14922,#14923));
#3297=EDGE_LOOP('',(#14924,#14925,#14926,#14927,#14928,#14929,#14930,#14931,
#14932,#14933,#14934,#14935,#14936,#14937,#14938,#14939,#14940,#14941,#14942,
#14943,#14944,#14945,#14946,#14947,#14948,#14949,#14950,#14951,#14952,#14953,
#14954,#14955,#14956,#14957,#14958,#14959,#14960,#14961,#14962,#14963,#14964,
#14965,#14966,#14967));
#3298=EDGE_LOOP('',(#14968,#14969,#14970,#14971));
#3299=EDGE_LOOP('',(#14972,#14973,#14974,#14975,#14976,#14977,#14978,#14979,
#14980,#14981,#14982,#14983,#14984,#14985,#14986,#14987,#14988,#14989,#14990,
#14991,#14992,#14993,#14994,#14995,#14996,#14997,#14998,#14999,#15000,#15001,
#15002,#15003,#15004,#15005,#15006,#15007,#15008,#15009,#15010,#15011,#15012,
#15013,#15014,#15015,#15016));
#3300=EDGE_LOOP('',(#15017,#15018,#15019,#15020));
#3301=EDGE_LOOP('',(#15021,#15022,#15023,#15024,#15025));
#3302=EDGE_LOOP('',(#15026,#15027,#15028));
#3303=EDGE_LOOP('',(#15029,#15030,#15031));
#3304=EDGE_LOOP('',(#15032,#15033,#15034,#15035,#15036,#15037));
#3305=EDGE_LOOP('',(#15038,#15039,#15040,#15041,#15042));
#3306=EDGE_LOOP('',(#15043,#15044,#15045,#15046,#15047));
#3307=EDGE_LOOP('',(#15048,#15049,#15050,#15051));
#3308=EDGE_LOOP('',(#15052,#15053,#15054,#15055));
#3309=EDGE_LOOP('',(#15056));
#3310=EDGE_LOOP('',(#15057));
#3311=EDGE_LOOP('',(#15058));
#3312=EDGE_LOOP('',(#15059));
#3313=EDGE_LOOP('',(#15060,#15061,#15062,#15063));
#4449=LINE('',#27558,#6159);
#4450=LINE('',#27560,#6160);
#4451=LINE('',#27584,#6161);
#4452=LINE('',#27660,#6162);
#4453=LINE('',#27736,#6163);
#4454=LINE('',#27814,#6164);
#4455=LINE('',#27890,#6165);
#4456=LINE('',#27966,#6166);
#4457=LINE('',#28042,#6167);
#4458=LINE('',#28118,#6168);
#4459=LINE('',#28196,#6169);
#4460=LINE('',#28272,#6170);
#4461=LINE('',#28348,#6171);
#4462=LINE('',#28426,#6172);
#4463=LINE('',#28502,#6173);
#4464=LINE('',#28578,#6174);
#4465=LINE('',#28654,#6175);
#4466=LINE('',#28732,#6176);
#4467=LINE('',#28808,#6177);
#4468=LINE('',#28884,#6178);
#4469=LINE('',#28957,#6179);
#4470=LINE('',#28962,#6180);
#4471=LINE('',#28973,#6181);
#4472=LINE('',#28983,#6182);
#4473=LINE('',#28994,#6183);
#4474=LINE('',#29024,#6184);
#4475=LINE('',#29054,#6185);
#4476=LINE('',#29084,#6186);
#4477=LINE('',#29114,#6187);
#4478=LINE('',#29144,#6188);
#4479=LINE('',#29174,#6189);
#4480=LINE('',#29204,#6190);
#4481=LINE('',#29234,#6191);
#4482=LINE('',#29264,#6192);
#4483=LINE('',#29294,#6193);
#4484=LINE('',#29324,#6194);
#4485=LINE('',#29354,#6195);
#4486=LINE('',#29384,#6196);
#4487=LINE('',#29414,#6197);
#4488=LINE('',#29444,#6198);
#4489=LINE('',#29474,#6199);
#4490=LINE('',#29504,#6200);
#4491=LINE('',#29534,#6201);
#4492=LINE('',#29544,#6202);
#4493=LINE('',#29555,#6203);
#4494=LINE('',#29622,#6204);
#4495=LINE('',#29698,#6205);
#4496=LINE('',#29774,#6206);
#4497=LINE('',#29786,#6207);
#4498=LINE('',#29799,#6208);
#4499=LINE('',#29837,#6209);
#4500=LINE('',#29875,#6210);
#4501=LINE('',#29913,#6211);
#4502=LINE('',#29951,#6212);
#4503=LINE('',#29989,#6213);
#4504=LINE('',#30027,#6214);
#4505=LINE('',#30065,#6215);
#4506=LINE('',#30112,#6216);
#4507=LINE('',#30190,#6217);
#4508=LINE('',#30266,#6218);
#4509=LINE('',#30295,#6219);
#4510=LINE('',#30400,#6220);
#4511=LINE('',#30402,#6221);
#4512=LINE('',#30403,#6222);
#4513=LINE('',#30410,#6223);
#4514=LINE('',#30411,#6224);
#4515=LINE('',#30418,#6225);
#4516=LINE('',#30419,#6226);
#4517=LINE('',#30426,#6227);
#4518=LINE('',#30427,#6228);
#4519=LINE('',#30431,#6229);
#4520=LINE('',#30433,#6230);
#4521=LINE('',#30435,#6231);
#4522=LINE('',#30444,#6232);
#4523=LINE('',#30445,#6233);
#4524=LINE('',#30446,#6234);
#4525=LINE('',#30452,#6235);
#4526=LINE('',#30459,#6236);
#4527=LINE('',#30460,#6237);
#4528=LINE('',#30464,#6238);
#4529=LINE('',#30466,#6239);
#4530=LINE('',#30468,#6240);
#4531=LINE('',#30477,#6241);
#4532=LINE('',#30478,#6242);
#4533=LINE('',#30479,#6243);
#4534=LINE('',#30485,#6244);
#4535=LINE('',#30492,#6245);
#4536=LINE('',#30493,#6246);
#4537=LINE('',#30497,#6247);
#4538=LINE('',#30499,#6248);
#4539=LINE('',#30501,#6249);
#4540=LINE('',#30512,#6250);
#4541=LINE('',#30513,#6251);
#4542=LINE('',#30514,#6252);
#4543=LINE('',#30524,#6253);
#4544=LINE('',#30531,#6254);
#4545=LINE('',#30532,#6255);
#4546=LINE('',#30541,#6256);
#4547=LINE('',#30572,#6257);
#4548=LINE('',#30581,#6258);
#4549=LINE('',#30851,#6259);
#4550=LINE('',#30862,#6260);
#4551=LINE('',#31182,#6261);
#4552=LINE('',#31193,#6262);
#4553=LINE('',#31195,#6263);
#4554=LINE('',#31203,#6264);
#4555=LINE('',#31206,#6265);
#4556=LINE('',#31224,#6266);
#4557=LINE('',#31230,#6267);
#4558=LINE('',#31248,#6268);
#4559=LINE('',#31271,#6269);
#4560=LINE('',#31277,#6270);
#4561=LINE('',#31284,#6271);
#4562=LINE('',#31291,#6272);
#4563=LINE('',#31296,#6273);
#4564=LINE('',#31301,#6274);
#4565=LINE('',#31303,#6275);
#4566=LINE('',#31305,#6276);
#4567=LINE('',#31306,#6277);
#4568=LINE('',#31309,#6278);
#4569=LINE('',#31311,#6279);
#4570=LINE('',#31312,#6280);
#4571=LINE('',#31315,#6281);
#4572=LINE('',#31317,#6282);
#4573=LINE('',#31318,#6283);
#4574=LINE('',#31321,#6284);
#4575=LINE('',#31323,#6285);
#4576=LINE('',#31324,#6286);
#4577=LINE('',#31327,#6287);
#4578=LINE('',#31329,#6288);
#4579=LINE('',#31330,#6289);
#4580=LINE('',#31333,#6290);
#4581=LINE('',#31335,#6291);
#4582=LINE('',#31336,#6292);
#4583=LINE('',#31339,#6293);
#4584=LINE('',#31341,#6294);
#4585=LINE('',#31342,#6295);
#4586=LINE('',#31345,#6296);
#4587=LINE('',#31347,#6297);
#4588=LINE('',#31348,#6298);
#4589=LINE('',#31351,#6299);
#4590=LINE('',#31353,#6300);
#4591=LINE('',#31354,#6301);
#4592=LINE('',#31357,#6302);
#4593=LINE('',#31359,#6303);
#4594=LINE('',#31360,#6304);
#4595=LINE('',#31363,#6305);
#4596=LINE('',#31365,#6306);
#4597=LINE('',#31366,#6307);
#4598=LINE('',#31369,#6308);
#4599=LINE('',#31371,#6309);
#4600=LINE('',#31372,#6310);
#4601=LINE('',#31375,#6311);
#4602=LINE('',#31377,#6312);
#4603=LINE('',#31378,#6313);
#4604=LINE('',#31381,#6314);
#4605=LINE('',#31383,#6315);
#4606=LINE('',#31384,#6316);
#4607=LINE('',#31387,#6317);
#4608=LINE('',#31389,#6318);
#4609=LINE('',#31390,#6319);
#4610=LINE('',#31393,#6320);
#4611=LINE('',#31395,#6321);
#4612=LINE('',#31396,#6322);
#4613=LINE('',#31399,#6323);
#4614=LINE('',#31401,#6324);
#4615=LINE('',#31402,#6325);
#4616=LINE('',#31405,#6326);
#4617=LINE('',#31407,#6327);
#4618=LINE('',#31408,#6328);
#4619=LINE('',#31411,#6329);
#4620=LINE('',#31413,#6330);
#4621=LINE('',#31414,#6331);
#4622=LINE('',#31417,#6332);
#4623=LINE('',#31419,#6333);
#4624=LINE('',#31420,#6334);
#4625=LINE('',#31423,#6335);
#4626=LINE('',#31425,#6336);
#4627=LINE('',#31426,#6337);
#4628=LINE('',#31429,#6338);
#4629=LINE('',#31431,#6339);
#4630=LINE('',#31432,#6340);
#4631=LINE('',#31435,#6341);
#4632=LINE('',#31437,#6342);
#4633=LINE('',#31438,#6343);
#4634=LINE('',#31441,#6344);
#4635=LINE('',#31443,#6345);
#4636=LINE('',#31444,#6346);
#4637=LINE('',#31447,#6347);
#4638=LINE('',#31449,#6348);
#4639=LINE('',#31450,#6349);
#4640=LINE('',#31453,#6350);
#4641=LINE('',#31455,#6351);
#4642=LINE('',#31456,#6352);
#4643=LINE('',#31459,#6353);
#4644=LINE('',#31461,#6354);
#4645=LINE('',#31462,#6355);
#4646=LINE('',#31465,#6356);
#4647=LINE('',#31467,#6357);
#4648=LINE('',#31468,#6358);
#4649=LINE('',#31471,#6359);
#4650=LINE('',#31473,#6360);
#4651=LINE('',#31474,#6361);
#4652=LINE('',#31477,#6362);
#4653=LINE('',#31479,#6363);
#4654=LINE('',#31480,#6364);
#4655=LINE('',#31483,#6365);
#4656=LINE('',#31485,#6366);
#4657=LINE('',#31486,#6367);
#4658=LINE('',#31489,#6368);
#4659=LINE('',#31491,#6369);
#4660=LINE('',#31492,#6370);
#4661=LINE('',#31495,#6371);
#4662=LINE('',#31497,#6372);
#4663=LINE('',#31498,#6373);
#4664=LINE('',#31501,#6374);
#4665=LINE('',#31503,#6375);
#4666=LINE('',#31504,#6376);
#4667=LINE('',#31507,#6377);
#4668=LINE('',#31509,#6378);
#4669=LINE('',#31510,#6379);
#4670=LINE('',#31513,#6380);
#4671=LINE('',#31515,#6381);
#4672=LINE('',#31516,#6382);
#4673=LINE('',#31519,#6383);
#4674=LINE('',#31521,#6384);
#4675=LINE('',#31522,#6385);
#4676=LINE('',#31525,#6386);
#4677=LINE('',#31527,#6387);
#4678=LINE('',#31528,#6388);
#4679=LINE('',#31531,#6389);
#4680=LINE('',#31533,#6390);
#4681=LINE('',#31534,#6391);
#4682=LINE('',#31537,#6392);
#4683=LINE('',#31539,#6393);
#4684=LINE('',#31540,#6394);
#4685=LINE('',#31543,#6395);
#4686=LINE('',#31545,#6396);
#4687=LINE('',#31546,#6397);
#4688=LINE('',#31549,#6398);
#4689=LINE('',#31551,#6399);
#4690=LINE('',#31552,#6400);
#4691=LINE('',#31555,#6401);
#4692=LINE('',#31557,#6402);
#4693=LINE('',#31558,#6403);
#4694=LINE('',#31561,#6404);
#4695=LINE('',#31563,#6405);
#4696=LINE('',#31564,#6406);
#4697=LINE('',#31567,#6407);
#4698=LINE('',#31569,#6408);
#4699=LINE('',#31570,#6409);
#4700=LINE('',#31573,#6410);
#4701=LINE('',#31575,#6411);
#4702=LINE('',#31576,#6412);
#4703=LINE('',#31579,#6413);
#4704=LINE('',#31581,#6414);
#4705=LINE('',#31582,#6415);
#4706=LINE('',#31585,#6416);
#4707=LINE('',#31587,#6417);
#4708=LINE('',#31588,#6418);
#4709=LINE('',#31591,#6419);
#4710=LINE('',#31593,#6420);
#4711=LINE('',#31594,#6421);
#4712=LINE('',#31597,#6422);
#4713=LINE('',#31599,#6423);
#4714=LINE('',#31600,#6424);
#4715=LINE('',#31603,#6425);
#4716=LINE('',#31605,#6426);
#4717=LINE('',#31606,#6427);
#4718=LINE('',#31609,#6428);
#4719=LINE('',#31611,#6429);
#4720=LINE('',#31612,#6430);
#4721=LINE('',#31615,#6431);
#4722=LINE('',#31617,#6432);
#4723=LINE('',#31618,#6433);
#4724=LINE('',#31621,#6434);
#4725=LINE('',#31623,#6435);
#4726=LINE('',#31624,#6436);
#4727=LINE('',#31627,#6437);
#4728=LINE('',#31629,#6438);
#4729=LINE('',#31630,#6439);
#4730=LINE('',#31633,#6440);
#4731=LINE('',#31635,#6441);
#4732=LINE('',#31636,#6442);
#4733=LINE('',#31639,#6443);
#4734=LINE('',#31641,#6444);
#4735=LINE('',#31642,#6445);
#4736=LINE('',#31645,#6446);
#4737=LINE('',#31647,#6447);
#4738=LINE('',#31648,#6448);
#4739=LINE('',#31651,#6449);
#4740=LINE('',#31653,#6450);
#4741=LINE('',#31654,#6451);
#4742=LINE('',#31657,#6452);
#4743=LINE('',#31659,#6453);
#4744=LINE('',#31660,#6454);
#4745=LINE('',#31663,#6455);
#4746=LINE('',#31665,#6456);
#4747=LINE('',#31666,#6457);
#4748=LINE('',#31669,#6458);
#4749=LINE('',#31671,#6459);
#4750=LINE('',#31672,#6460);
#4751=LINE('',#31675,#6461);
#4752=LINE('',#31677,#6462);
#4753=LINE('',#31678,#6463);
#4754=LINE('',#31681,#6464);
#4755=LINE('',#31683,#6465);
#4756=LINE('',#31684,#6466);
#4757=LINE('',#31687,#6467);
#4758=LINE('',#31689,#6468);
#4759=LINE('',#31690,#6469);
#4760=LINE('',#31693,#6470);
#4761=LINE('',#31695,#6471);
#4762=LINE('',#31696,#6472);
#4763=LINE('',#31699,#6473);
#4764=LINE('',#31701,#6474);
#4765=LINE('',#31702,#6475);
#4766=LINE('',#31705,#6476);
#4767=LINE('',#31707,#6477);
#4768=LINE('',#31708,#6478);
#4769=LINE('',#31711,#6479);
#4770=LINE('',#31713,#6480);
#4771=LINE('',#31714,#6481);
#4772=LINE('',#31717,#6482);
#4773=LINE('',#31719,#6483);
#4774=LINE('',#31720,#6484);
#4775=LINE('',#31723,#6485);
#4776=LINE('',#31725,#6486);
#4777=LINE('',#31726,#6487);
#4778=LINE('',#31729,#6488);
#4779=LINE('',#31731,#6489);
#4780=LINE('',#31732,#6490);
#4781=LINE('',#31735,#6491);
#4782=LINE('',#31737,#6492);
#4783=LINE('',#31738,#6493);
#4784=LINE('',#31741,#6494);
#4785=LINE('',#31743,#6495);
#4786=LINE('',#31744,#6496);
#4787=LINE('',#31747,#6497);
#4788=LINE('',#31749,#6498);
#4789=LINE('',#31750,#6499);
#4790=LINE('',#31753,#6500);
#4791=LINE('',#31755,#6501);
#4792=LINE('',#31756,#6502);
#4793=LINE('',#31759,#6503);
#4794=LINE('',#31761,#6504);
#4795=LINE('',#31762,#6505);
#4796=LINE('',#31765,#6506);
#4797=LINE('',#31767,#6507);
#4798=LINE('',#31768,#6508);
#4799=LINE('',#31771,#6509);
#4800=LINE('',#31773,#6510);
#4801=LINE('',#31774,#6511);
#4802=LINE('',#31777,#6512);
#4803=LINE('',#31779,#6513);
#4804=LINE('',#31780,#6514);
#4805=LINE('',#31783,#6515);
#4806=LINE('',#31785,#6516);
#4807=LINE('',#31786,#6517);
#4808=LINE('',#31789,#6518);
#4809=LINE('',#31791,#6519);
#4810=LINE('',#31792,#6520);
#4811=LINE('',#31795,#6521);
#4812=LINE('',#31797,#6522);
#4813=LINE('',#31798,#6523);
#4814=LINE('',#31801,#6524);
#4815=LINE('',#31803,#6525);
#4816=LINE('',#31804,#6526);
#4817=LINE('',#31807,#6527);
#4818=LINE('',#31809,#6528);
#4819=LINE('',#31810,#6529);
#4820=LINE('',#31813,#6530);
#4821=LINE('',#31815,#6531);
#4822=LINE('',#31816,#6532);
#4823=LINE('',#31819,#6533);
#4824=LINE('',#31821,#6534);
#4825=LINE('',#31822,#6535);
#4826=LINE('',#31825,#6536);
#4827=LINE('',#31827,#6537);
#4828=LINE('',#31828,#6538);
#4829=LINE('',#31831,#6539);
#4830=LINE('',#31833,#6540);
#4831=LINE('',#31834,#6541);
#4832=LINE('',#31836,#6542);
#4833=LINE('',#31837,#6543);
#4834=LINE('',#31852,#6544);
#4835=LINE('',#32335,#6545);
#4836=LINE('',#32383,#6546);
#4837=LINE('',#32894,#6547);
#4838=LINE('',#32895,#6548);
#4839=LINE('',#32943,#6549);
#4840=LINE('',#32950,#6550);
#4841=LINE('',#32954,#6551);
#4842=LINE('',#32958,#6552);
#4843=LINE('',#32964,#6553);
#4844=LINE('',#32967,#6554);
#6159=VECTOR('',#22049,1.60000000000001);
#6160=VECTOR('',#22050,1000.);
#6161=VECTOR('',#22055,1.60000000000001);
#6162=VECTOR('',#22058,1.60000000000001);
#6163=VECTOR('',#22061,1.60000000000001);
#6164=VECTOR('',#22064,1.60000000000001);
#6165=VECTOR('',#22067,1.60000000000001);
#6166=VECTOR('',#22070,1.60000000000001);
#6167=VECTOR('',#22073,1.60000000000001);
#6168=VECTOR('',#22076,1.60000000000001);
#6169=VECTOR('',#22079,1.60000000000001);
#6170=VECTOR('',#22082,1.60000000000001);
#6171=VECTOR('',#22085,1.60000000000001);
#6172=VECTOR('',#22088,1.60000000000001);
#6173=VECTOR('',#22091,1.60000000000001);
#6174=VECTOR('',#22094,1.60000000000001);
#6175=VECTOR('',#22097,1.60000000000001);
#6176=VECTOR('',#22100,1.60000000000001);
#6177=VECTOR('',#22103,1.60000000000001);
#6178=VECTOR('',#22106,1.60000000000001);
#6179=VECTOR('',#22111,1.59999999999791);
#6180=VECTOR('',#22116,1000.);
#6181=VECTOR('',#22119,1.22111388749974);
#6182=VECTOR('',#22120,1000.);
#6183=VECTOR('',#22123,1.22111388749974);
#6184=VECTOR('',#22126,1.22111388749974);
#6185=VECTOR('',#22129,1.22111388749974);
#6186=VECTOR('',#22132,1.22111388749974);
#6187=VECTOR('',#22135,1.22111388749974);
#6188=VECTOR('',#22138,1.22111388749974);
#6189=VECTOR('',#22141,1.22111388749974);
#6190=VECTOR('',#22144,1.22111388749974);
#6191=VECTOR('',#22147,1.22111388749974);
#6192=VECTOR('',#22150,1.22111388749974);
#6193=VECTOR('',#22153,1.22111388749974);
#6194=VECTOR('',#22156,1.22111388749974);
#6195=VECTOR('',#22159,1.22111388749974);
#6196=VECTOR('',#22162,1.22111388749974);
#6197=VECTOR('',#22165,1.22111388749974);
#6198=VECTOR('',#22168,1.22111388749974);
#6199=VECTOR('',#22171,1.22111388749974);
#6200=VECTOR('',#22174,1.22111388749974);
#6201=VECTOR('',#22177,1.22111388749974);
#6202=VECTOR('',#22178,1000.);
#6203=VECTOR('',#22181,8.49999999999999);
#6204=VECTOR('',#22186,8.49999999999999);
#6205=VECTOR('',#22189,8.49999999999999);
#6206=VECTOR('',#22192,7.68810118749996);
#6207=VECTOR('',#22193,1000.);
#6208=VECTOR('',#22196,7.68810118749996);
#6209=VECTOR('',#22199,7.68810118749996);
#6210=VECTOR('',#22202,7.68810118749996);
#6211=VECTOR('',#22205,7.68810118749996);
#6212=VECTOR('',#22208,7.68810118749996);
#6213=VECTOR('',#22211,7.68810118749996);
#6214=VECTOR('',#22214,7.68810118749996);
#6215=VECTOR('',#22217,8.10000000000001);
#6216=VECTOR('',#22222,8.10000000000001);
#6217=VECTOR('',#22225,8.10000000000001);
#6218=VECTOR('',#22228,8.10000000000001);
#6219=VECTOR('',#22229,1000.);
#6220=VECTOR('',#22236,1000.);
#6221=VECTOR('',#22237,1000.);
#6222=VECTOR('',#22238,1000.);
#6223=VECTOR('',#22241,1000.);
#6224=VECTOR('',#22242,1000.);
#6225=VECTOR('',#22245,1000.);
#6226=VECTOR('',#22246,1000.);
#6227=VECTOR('',#22249,1000.);
#6228=VECTOR('',#22250,1000.);
#6229=VECTOR('',#22253,1000.);
#6230=VECTOR('',#22254,1000.);
#6231=VECTOR('',#22255,1000.);
#6232=VECTOR('',#22260,1000.);
#6233=VECTOR('',#22261,1000.);
#6234=VECTOR('',#22262,1000.);
#6235=VECTOR('',#22265,1000.);
#6236=VECTOR('',#22268,1000.);
#6237=VECTOR('',#22269,1000.);
#6238=VECTOR('',#22272,1000.);
#6239=VECTOR('',#22273,1000.);
#6240=VECTOR('',#22274,1000.);
#6241=VECTOR('',#22279,1000.);
#6242=VECTOR('',#22280,1000.);
#6243=VECTOR('',#22281,1000.);
#6244=VECTOR('',#22284,1000.);
#6245=VECTOR('',#22287,1000.);
#6246=VECTOR('',#22288,1000.);
#6247=VECTOR('',#22291,1000.);
#6248=VECTOR('',#22292,1000.);
#6249=VECTOR('',#22293,1000.);
#6250=VECTOR('',#22300,1000.);
#6251=VECTOR('',#22301,1000.);
#6252=VECTOR('',#22302,1000.);
#6253=VECTOR('',#22305,1000.);
#6254=VECTOR('',#22308,1000.);
#6255=VECTOR('',#22309,1000.);
#6256=VECTOR('',#22324,12.);
#6257=VECTOR('',#22337,8.10000000000001);
#6258=VECTOR('',#22352,14.);
#6259=VECTOR('',#22373,1000.);
#6260=VECTOR('',#22374,1000.);
#6261=VECTOR('',#22375,1000.);
#6262=VECTOR('',#22376,1000.);
#6263=VECTOR('',#22379,1000.);
#6264=VECTOR('',#22388,6.00000000000001);
#6265=VECTOR('',#22393,1000.);
#6266=VECTOR('',#22418,4.75);
#6267=VECTOR('',#22425,7.00000000000001);
#6268=VECTOR('',#22446,10.);
#6269=VECTOR('',#22481,1.2500000000005);
#6270=VECTOR('',#22488,1.25000000000059);
#6271=VECTOR('',#22497,1.25000000000024);
#6272=VECTOR('',#22506,1.24999999999999);
#6273=VECTOR('',#22513,6.00000000000001);
#6274=VECTOR('',#22518,1000.);
#6275=VECTOR('',#22519,1000.);
#6276=VECTOR('',#22520,1000.);
#6277=VECTOR('',#22521,1000.);
#6278=VECTOR('',#22524,1000.);
#6279=VECTOR('',#22525,1000.);
#6280=VECTOR('',#22526,1000.);
#6281=VECTOR('',#22529,1000.);
#6282=VECTOR('',#22530,1000.);
#6283=VECTOR('',#22531,1000.);
#6284=VECTOR('',#22534,1000.);
#6285=VECTOR('',#22535,1000.);
#6286=VECTOR('',#22536,1000.);
#6287=VECTOR('',#22539,1000.);
#6288=VECTOR('',#22540,1000.);
#6289=VECTOR('',#22541,1000.);
#6290=VECTOR('',#22544,1000.);
#6291=VECTOR('',#22545,1000.);
#6292=VECTOR('',#22546,1000.);
#6293=VECTOR('',#22549,1000.);
#6294=VECTOR('',#22550,1000.);
#6295=VECTOR('',#22551,1000.);
#6296=VECTOR('',#22554,1000.);
#6297=VECTOR('',#22555,1000.);
#6298=VECTOR('',#22556,1000.);
#6299=VECTOR('',#22559,1000.);
#6300=VECTOR('',#22560,1000.);
#6301=VECTOR('',#22561,1000.);
#6302=VECTOR('',#22564,1000.);
#6303=VECTOR('',#22565,1000.);
#6304=VECTOR('',#22566,1000.);
#6305=VECTOR('',#22569,1000.);
#6306=VECTOR('',#22570,1000.);
#6307=VECTOR('',#22571,1000.);
#6308=VECTOR('',#22574,1000.);
#6309=VECTOR('',#22575,1000.);
#6310=VECTOR('',#22576,1000.);
#6311=VECTOR('',#22579,1000.);
#6312=VECTOR('',#22580,1000.);
#6313=VECTOR('',#22581,1000.);
#6314=VECTOR('',#22584,1000.);
#6315=VECTOR('',#22585,1000.);
#6316=VECTOR('',#22586,1000.);
#6317=VECTOR('',#22589,1000.);
#6318=VECTOR('',#22590,1000.);
#6319=VECTOR('',#22591,1000.);
#6320=VECTOR('',#22594,1000.);
#6321=VECTOR('',#22595,1000.);
#6322=VECTOR('',#22596,1000.);
#6323=VECTOR('',#22599,1000.);
#6324=VECTOR('',#22600,1000.);
#6325=VECTOR('',#22601,1000.);
#6326=VECTOR('',#22604,1000.);
#6327=VECTOR('',#22605,1000.);
#6328=VECTOR('',#22606,1000.);
#6329=VECTOR('',#22609,1000.);
#6330=VECTOR('',#22610,1000.);
#6331=VECTOR('',#22611,1000.);
#6332=VECTOR('',#22614,1000.);
#6333=VECTOR('',#22615,1000.);
#6334=VECTOR('',#22616,1000.);
#6335=VECTOR('',#22619,1000.);
#6336=VECTOR('',#22620,1000.);
#6337=VECTOR('',#22621,1000.);
#6338=VECTOR('',#22624,1000.);
#6339=VECTOR('',#22625,1000.);
#6340=VECTOR('',#22626,1000.);
#6341=VECTOR('',#22629,1000.);
#6342=VECTOR('',#22630,1000.);
#6343=VECTOR('',#22631,1000.);
#6344=VECTOR('',#22634,1000.);
#6345=VECTOR('',#22635,1000.);
#6346=VECTOR('',#22636,1000.);
#6347=VECTOR('',#22639,1000.);
#6348=VECTOR('',#22640,1000.);
#6349=VECTOR('',#22641,1000.);
#6350=VECTOR('',#22644,1000.);
#6351=VECTOR('',#22645,1000.);
#6352=VECTOR('',#22646,1000.);
#6353=VECTOR('',#22649,1000.);
#6354=VECTOR('',#22650,1000.);
#6355=VECTOR('',#22651,1000.);
#6356=VECTOR('',#22654,1000.);
#6357=VECTOR('',#22655,1000.);
#6358=VECTOR('',#22656,1000.);
#6359=VECTOR('',#22659,1000.);
#6360=VECTOR('',#22660,1000.);
#6361=VECTOR('',#22661,1000.);
#6362=VECTOR('',#22664,1000.);
#6363=VECTOR('',#22665,1000.);
#6364=VECTOR('',#22666,1000.);
#6365=VECTOR('',#22669,1000.);
#6366=VECTOR('',#22670,1000.);
#6367=VECTOR('',#22671,1000.);
#6368=VECTOR('',#22674,1000.);
#6369=VECTOR('',#22675,1000.);
#6370=VECTOR('',#22676,1000.);
#6371=VECTOR('',#22679,1000.);
#6372=VECTOR('',#22680,1000.);
#6373=VECTOR('',#22681,1000.);
#6374=VECTOR('',#22684,1000.);
#6375=VECTOR('',#22685,1000.);
#6376=VECTOR('',#22686,1000.);
#6377=VECTOR('',#22689,1000.);
#6378=VECTOR('',#22690,1000.);
#6379=VECTOR('',#22691,1000.);
#6380=VECTOR('',#22694,1000.);
#6381=VECTOR('',#22695,1000.);
#6382=VECTOR('',#22696,1000.);
#6383=VECTOR('',#22699,1000.);
#6384=VECTOR('',#22700,1000.);
#6385=VECTOR('',#22701,1000.);
#6386=VECTOR('',#22704,1000.);
#6387=VECTOR('',#22705,1000.);
#6388=VECTOR('',#22706,1000.);
#6389=VECTOR('',#22709,1000.);
#6390=VECTOR('',#22710,1000.);
#6391=VECTOR('',#22711,1000.);
#6392=VECTOR('',#22714,1000.);
#6393=VECTOR('',#22715,1000.);
#6394=VECTOR('',#22716,1000.);
#6395=VECTOR('',#22719,1000.);
#6396=VECTOR('',#22720,1000.);
#6397=VECTOR('',#22721,1000.);
#6398=VECTOR('',#22724,1000.);
#6399=VECTOR('',#22725,1000.);
#6400=VECTOR('',#22726,1000.);
#6401=VECTOR('',#22729,1000.);
#6402=VECTOR('',#22730,1000.);
#6403=VECTOR('',#22731,1000.);
#6404=VECTOR('',#22734,1000.);
#6405=VECTOR('',#22735,1000.);
#6406=VECTOR('',#22736,1000.);
#6407=VECTOR('',#22739,1000.);
#6408=VECTOR('',#22740,1000.);
#6409=VECTOR('',#22741,1000.);
#6410=VECTOR('',#22744,1000.);
#6411=VECTOR('',#22745,1000.);
#6412=VECTOR('',#22746,1000.);
#6413=VECTOR('',#22749,1000.);
#6414=VECTOR('',#22750,1000.);
#6415=VECTOR('',#22751,1000.);
#6416=VECTOR('',#22754,1000.);
#6417=VECTOR('',#22755,1000.);
#6418=VECTOR('',#22756,1000.);
#6419=VECTOR('',#22759,1000.);
#6420=VECTOR('',#22760,1000.);
#6421=VECTOR('',#22761,1000.);
#6422=VECTOR('',#22764,1000.);
#6423=VECTOR('',#22765,1000.);
#6424=VECTOR('',#22766,1000.);
#6425=VECTOR('',#22769,1000.);
#6426=VECTOR('',#22770,1000.);
#6427=VECTOR('',#22771,1000.);
#6428=VECTOR('',#22774,1000.);
#6429=VECTOR('',#22775,1000.);
#6430=VECTOR('',#22776,1000.);
#6431=VECTOR('',#22779,1000.);
#6432=VECTOR('',#22780,1000.);
#6433=VECTOR('',#22781,1000.);
#6434=VECTOR('',#22784,1000.);
#6435=VECTOR('',#22785,1000.);
#6436=VECTOR('',#22786,1000.);
#6437=VECTOR('',#22789,1000.);
#6438=VECTOR('',#22790,1000.);
#6439=VECTOR('',#22791,1000.);
#6440=VECTOR('',#22794,1000.);
#6441=VECTOR('',#22795,1000.);
#6442=VECTOR('',#22796,1000.);
#6443=VECTOR('',#22799,1000.);
#6444=VECTOR('',#22800,1000.);
#6445=VECTOR('',#22801,1000.);
#6446=VECTOR('',#22804,1000.);
#6447=VECTOR('',#22805,1000.);
#6448=VECTOR('',#22806,1000.);
#6449=VECTOR('',#22809,1000.);
#6450=VECTOR('',#22810,1000.);
#6451=VECTOR('',#22811,1000.);
#6452=VECTOR('',#22814,1000.);
#6453=VECTOR('',#22815,1000.);
#6454=VECTOR('',#22816,1000.);
#6455=VECTOR('',#22819,1000.);
#6456=VECTOR('',#22820,1000.);
#6457=VECTOR('',#22821,1000.);
#6458=VECTOR('',#22824,1000.);
#6459=VECTOR('',#22825,1000.);
#6460=VECTOR('',#22826,1000.);
#6461=VECTOR('',#22829,1000.);
#6462=VECTOR('',#22830,1000.);
#6463=VECTOR('',#22831,1000.);
#6464=VECTOR('',#22834,1000.);
#6465=VECTOR('',#22835,1000.);
#6466=VECTOR('',#22836,1000.);
#6467=VECTOR('',#22839,1000.);
#6468=VECTOR('',#22840,1000.);
#6469=VECTOR('',#22841,1000.);
#6470=VECTOR('',#22844,1000.);
#6471=VECTOR('',#22845,1000.);
#6472=VECTOR('',#22846,1000.);
#6473=VECTOR('',#22849,1000.);
#6474=VECTOR('',#22850,1000.);
#6475=VECTOR('',#22851,1000.);
#6476=VECTOR('',#22854,1000.);
#6477=VECTOR('',#22855,1000.);
#6478=VECTOR('',#22856,1000.);
#6479=VECTOR('',#22859,1000.);
#6480=VECTOR('',#22860,1000.);
#6481=VECTOR('',#22861,1000.);
#6482=VECTOR('',#22864,1000.);
#6483=VECTOR('',#22865,1000.);
#6484=VECTOR('',#22866,1000.);
#6485=VECTOR('',#22869,1000.);
#6486=VECTOR('',#22870,1000.);
#6487=VECTOR('',#22871,1000.);
#6488=VECTOR('',#22874,1000.);
#6489=VECTOR('',#22875,1000.);
#6490=VECTOR('',#22876,1000.);
#6491=VECTOR('',#22879,1000.);
#6492=VECTOR('',#22880,1000.);
#6493=VECTOR('',#22881,1000.);
#6494=VECTOR('',#22884,1000.);
#6495=VECTOR('',#22885,1000.);
#6496=VECTOR('',#22886,1000.);
#6497=VECTOR('',#22889,1000.);
#6498=VECTOR('',#22890,1000.);
#6499=VECTOR('',#22891,1000.);
#6500=VECTOR('',#22894,1000.);
#6501=VECTOR('',#22895,1000.);
#6502=VECTOR('',#22896,1000.);
#6503=VECTOR('',#22899,1000.);
#6504=VECTOR('',#22900,1000.);
#6505=VECTOR('',#22901,1000.);
#6506=VECTOR('',#22904,1000.);
#6507=VECTOR('',#22905,1000.);
#6508=VECTOR('',#22906,1000.);
#6509=VECTOR('',#22909,1000.);
#6510=VECTOR('',#22910,1000.);
#6511=VECTOR('',#22911,1000.);
#6512=VECTOR('',#22914,1000.);
#6513=VECTOR('',#22915,1000.);
#6514=VECTOR('',#22916,1000.);
#6515=VECTOR('',#22919,1000.);
#6516=VECTOR('',#22920,1000.);
#6517=VECTOR('',#22921,1000.);
#6518=VECTOR('',#22924,1000.);
#6519=VECTOR('',#22925,1000.);
#6520=VECTOR('',#22926,1000.);
#6521=VECTOR('',#22929,1000.);
#6522=VECTOR('',#22930,1000.);
#6523=VECTOR('',#22931,1000.);
#6524=VECTOR('',#22934,1000.);
#6525=VECTOR('',#22935,1000.);
#6526=VECTOR('',#22936,1000.);
#6527=VECTOR('',#22939,1000.);
#6528=VECTOR('',#22940,1000.);
#6529=VECTOR('',#22941,1000.);
#6530=VECTOR('',#22944,1000.);
#6531=VECTOR('',#22945,1000.);
#6532=VECTOR('',#22946,1000.);
#6533=VECTOR('',#22949,1000.);
#6534=VECTOR('',#22950,1000.);
#6535=VECTOR('',#22951,1000.);
#6536=VECTOR('',#22954,1000.);
#6537=VECTOR('',#22955,1000.);
#6538=VECTOR('',#22956,1000.);
#6539=VECTOR('',#22959,1000.);
#6540=VECTOR('',#22960,1000.);
#6541=VECTOR('',#22961,1000.);
#6542=VECTOR('',#22964,1000.);
#6543=VECTOR('',#22965,1000.);
#6544=VECTOR('',#22986,3.99999999999999);
#6545=VECTOR('',#22987,1000.);
#6546=VECTOR('',#22988,1000.);
#6547=VECTOR('',#22991,1000.);
#6548=VECTOR('',#22992,1000.);
#6549=VECTOR('',#22997,1000.);
#6550=VECTOR('',#23008,1.60000000000001);
#6551=VECTOR('',#23013,2.);
#6552=VECTOR('',#23018,3.99999999999999);
#6553=VECTOR('',#23025,3.6);
#6554=VECTOR('',#23030,3.99999999999999);
#7849=VERTEX_POINT('',#27556);
#7850=VERTEX_POINT('',#27557);
#7851=VERTEX_POINT('',#27559);
#7852=VERTEX_POINT('',#27561);
#7853=VERTEX_POINT('',#27582);
#7854=VERTEX_POINT('',#27583);
#7855=VERTEX_POINT('',#27658);
#7856=VERTEX_POINT('',#27659);
#7857=VERTEX_POINT('',#27734);
#7858=VERTEX_POINT('',#27735);
#7859=VERTEX_POINT('',#27812);
#7860=VERTEX_POINT('',#27813);
#7861=VERTEX_POINT('',#27888);
#7862=VERTEX_POINT('',#27889);
#7863=VERTEX_POINT('',#27964);
#7864=VERTEX_POINT('',#27965);
#7865=VERTEX_POINT('',#28040);
#7866=VERTEX_POINT('',#28041);
#7867=VERTEX_POINT('',#28116);
#7868=VERTEX_POINT('',#28117);
#7869=VERTEX_POINT('',#28194);
#7870=VERTEX_POINT('',#28195);
#7871=VERTEX_POINT('',#28270);
#7872=VERTEX_POINT('',#28271);
#7873=VERTEX_POINT('',#28346);
#7874=VERTEX_POINT('',#28347);
#7875=VERTEX_POINT('',#28424);
#7876=VERTEX_POINT('',#28425);
#7877=VERTEX_POINT('',#28500);
#7878=VERTEX_POINT('',#28501);
#7879=VERTEX_POINT('',#28576);
#7880=VERTEX_POINT('',#28577);
#7881=VERTEX_POINT('',#28652);
#7882=VERTEX_POINT('',#28653);
#7883=VERTEX_POINT('',#28730);
#7884=VERTEX_POINT('',#28731);
#7885=VERTEX_POINT('',#28806);
#7886=VERTEX_POINT('',#28807);
#7887=VERTEX_POINT('',#28882);
#7888=VERTEX_POINT('',#28883);
#7889=VERTEX_POINT('',#28885);
#7890=VERTEX_POINT('',#28918);
#7891=VERTEX_POINT('',#28955);
#7892=VERTEX_POINT('',#28956);
#7893=VERTEX_POINT('',#28959);
#7894=VERTEX_POINT('',#28961);
#7895=VERTEX_POINT('',#28971);
#7896=VERTEX_POINT('',#28972);
#7897=VERTEX_POINT('',#28974);
#7898=VERTEX_POINT('',#28982);
#7899=VERTEX_POINT('',#28992);
#7900=VERTEX_POINT('',#28993);
#7901=VERTEX_POINT('',#29022);
#7902=VERTEX_POINT('',#29023);
#7903=VERTEX_POINT('',#29052);
#7904=VERTEX_POINT('',#29053);
#7905=VERTEX_POINT('',#29082);
#7906=VERTEX_POINT('',#29083);
#7907=VERTEX_POINT('',#29112);
#7908=VERTEX_POINT('',#29113);
#7909=VERTEX_POINT('',#29142);
#7910=VERTEX_POINT('',#29143);
#7911=VERTEX_POINT('',#29172);
#7912=VERTEX_POINT('',#29173);
#7913=VERTEX_POINT('',#29202);
#7914=VERTEX_POINT('',#29203);
#7915=VERTEX_POINT('',#29232);
#7916=VERTEX_POINT('',#29233);
#7917=VERTEX_POINT('',#29262);
#7918=VERTEX_POINT('',#29263);
#7919=VERTEX_POINT('',#29292);
#7920=VERTEX_POINT('',#29293);
#7921=VERTEX_POINT('',#29322);
#7922=VERTEX_POINT('',#29323);
#7923=VERTEX_POINT('',#29352);
#7924=VERTEX_POINT('',#29353);
#7925=VERTEX_POINT('',#29382);
#7926=VERTEX_POINT('',#29383);
#7927=VERTEX_POINT('',#29412);
#7928=VERTEX_POINT('',#29413);
#7929=VERTEX_POINT('',#29442);
#7930=VERTEX_POINT('',#29443);
#7931=VERTEX_POINT('',#29472);
#7932=VERTEX_POINT('',#29473);
#7933=VERTEX_POINT('',#29502);
#7934=VERTEX_POINT('',#29503);
#7935=VERTEX_POINT('',#29532);
#7936=VERTEX_POINT('',#29533);
#7937=VERTEX_POINT('',#29535);
#7938=VERTEX_POINT('',#29543);
#7939=VERTEX_POINT('',#29553);
#7940=VERTEX_POINT('',#29554);
#7941=VERTEX_POINT('',#29556);
#7942=VERTEX_POINT('',#29589);
#7943=VERTEX_POINT('',#29620);
#7944=VERTEX_POINT('',#29621);
#7945=VERTEX_POINT('',#29696);
#7946=VERTEX_POINT('',#29697);
#7947=VERTEX_POINT('',#29772);
#7948=VERTEX_POINT('',#29773);
#7949=VERTEX_POINT('',#29775);
#7950=VERTEX_POINT('',#29785);
#7951=VERTEX_POINT('',#29797);
#7952=VERTEX_POINT('',#29798);
#7953=VERTEX_POINT('',#29835);
#7954=VERTEX_POINT('',#29836);
#7955=VERTEX_POINT('',#29873);
#7956=VERTEX_POINT('',#29874);
#7957=VERTEX_POINT('',#29911);
#7958=VERTEX_POINT('',#29912);
#7959=VERTEX_POINT('',#29949);
#7960=VERTEX_POINT('',#29950);
#7961=VERTEX_POINT('',#29987);
#7962=VERTEX_POINT('',#29988);
#7963=VERTEX_POINT('',#30025);
#7964=VERTEX_POINT('',#30026);
#7965=VERTEX_POINT('',#30063);
#7966=VERTEX_POINT('',#30064);
#7967=VERTEX_POINT('',#30066);
#7968=VERTEX_POINT('',#30077);
#7969=VERTEX_POINT('',#30110);
#7970=VERTEX_POINT('',#30111);
#7971=VERTEX_POINT('',#30188);
#7972=VERTEX_POINT('',#30189);
#7973=VERTEX_POINT('',#30264);
#7974=VERTEX_POINT('',#30265);
#7975=VERTEX_POINT('',#30267);
#7976=VERTEX_POINT('',#30294);
#7977=VERTEX_POINT('',#30396);
#7978=VERTEX_POINT('',#30397);
#7979=VERTEX_POINT('',#30399);
#7980=VERTEX_POINT('',#30401);
#7981=VERTEX_POINT('',#30405);
#7982=VERTEX_POINT('',#30406);
#7983=VERTEX_POINT('',#30413);
#7984=VERTEX_POINT('',#30417);
#7985=VERTEX_POINT('',#30421);
#7986=VERTEX_POINT('',#30425);
#7987=VERTEX_POINT('',#30429);
#7988=VERTEX_POINT('',#30430);
#7989=VERTEX_POINT('',#30432);
#7990=VERTEX_POINT('',#30434);
#7991=VERTEX_POINT('',#30438);
#7992=VERTEX_POINT('',#30439);
#7993=VERTEX_POINT('',#30443);
#7994=VERTEX_POINT('',#30448);
#7995=VERTEX_POINT('',#30454);
#7996=VERTEX_POINT('',#30458);
#7997=VERTEX_POINT('',#30462);
#7998=VERTEX_POINT('',#30463);
#7999=VERTEX_POINT('',#30465);
#8000=VERTEX_POINT('',#30467);
#8001=VERTEX_POINT('',#30471);
#8002=VERTEX_POINT('',#30472);
#8003=VERTEX_POINT('',#30476);
#8004=VERTEX_POINT('',#30481);
#8005=VERTEX_POINT('',#30487);
#8006=VERTEX_POINT('',#30491);
#8007=VERTEX_POINT('',#30495);
#8008=VERTEX_POINT('',#30496);
#8009=VERTEX_POINT('',#30498);
#8010=VERTEX_POINT('',#30500);
#8011=VERTEX_POINT('',#30502);
#8012=VERTEX_POINT('',#30506);
#8013=VERTEX_POINT('',#30507);
#8014=VERTEX_POINT('',#30511);
#8015=VERTEX_POINT('',#30516);
#8016=VERTEX_POINT('',#30517);
#8017=VERTEX_POINT('',#30526);
#8018=VERTEX_POINT('',#30530);
#8019=VERTEX_POINT('',#30539);
#8020=VERTEX_POINT('',#30569);
#8021=VERTEX_POINT('',#30571);
#8022=VERTEX_POINT('',#30575);
#8023=VERTEX_POINT('',#30850);
#8024=VERTEX_POINT('',#30861);
#8025=VERTEX_POINT('',#30863);
#8026=VERTEX_POINT('',#31161);
#8027=VERTEX_POINT('',#31183);
#8028=VERTEX_POINT('',#31197);
#8029=VERTEX_POINT('',#31200);
#8030=VERTEX_POINT('',#31202);
#8031=VERTEX_POINT('',#31213);
#8032=VERTEX_POINT('',#31215);
#8033=VERTEX_POINT('',#31217);
#8034=VERTEX_POINT('',#31221);
#8035=VERTEX_POINT('',#31223);
#8036=VERTEX_POINT('',#31227);
#8037=VERTEX_POINT('',#31229);
#8038=VERTEX_POINT('',#31234);
#8039=VERTEX_POINT('',#31237);
#8040=VERTEX_POINT('',#31238);
#8041=VERTEX_POINT('',#31240);
#8042=VERTEX_POINT('',#31242);
#8043=VERTEX_POINT('',#31244);
#8044=VERTEX_POINT('',#31246);
#8045=VERTEX_POINT('',#31249);
#8046=VERTEX_POINT('',#31251);
#8047=VERTEX_POINT('',#31253);
#8048=VERTEX_POINT('',#31259);
#8049=VERTEX_POINT('',#31269);
#8050=VERTEX_POINT('',#31274);
#8051=VERTEX_POINT('',#31276);
#8052=VERTEX_POINT('',#31281);
#8053=VERTEX_POINT('',#31283);
#8054=VERTEX_POINT('',#31288);
#8055=VERTEX_POINT('',#31290);
#8056=VERTEX_POINT('',#31295);
#8057=VERTEX_POINT('',#31299);
#8058=VERTEX_POINT('',#31300);
#8059=VERTEX_POINT('',#31302);
#8060=VERTEX_POINT('',#31304);
#8061=VERTEX_POINT('',#31308);
#8062=VERTEX_POINT('',#31310);
#8063=VERTEX_POINT('',#31314);
#8064=VERTEX_POINT('',#31316);
#8065=VERTEX_POINT('',#31320);
#8066=VERTEX_POINT('',#31322);
#8067=VERTEX_POINT('',#31326);
#8068=VERTEX_POINT('',#31328);
#8069=VERTEX_POINT('',#31332);
#8070=VERTEX_POINT('',#31334);
#8071=VERTEX_POINT('',#31338);
#8072=VERTEX_POINT('',#31340);
#8073=VERTEX_POINT('',#31344);
#8074=VERTEX_POINT('',#31346);
#8075=VERTEX_POINT('',#31350);
#8076=VERTEX_POINT('',#31352);
#8077=VERTEX_POINT('',#31356);
#8078=VERTEX_POINT('',#31358);
#8079=VERTEX_POINT('',#31362);
#8080=VERTEX_POINT('',#31364);
#8081=VERTEX_POINT('',#31368);
#8082=VERTEX_POINT('',#31370);
#8083=VERTEX_POINT('',#31374);
#8084=VERTEX_POINT('',#31376);
#8085=VERTEX_POINT('',#31380);
#8086=VERTEX_POINT('',#31382);
#8087=VERTEX_POINT('',#31386);
#8088=VERTEX_POINT('',#31388);
#8089=VERTEX_POINT('',#31392);
#8090=VERTEX_POINT('',#31394);
#8091=VERTEX_POINT('',#31398);
#8092=VERTEX_POINT('',#31400);
#8093=VERTEX_POINT('',#31404);
#8094=VERTEX_POINT('',#31406);
#8095=VERTEX_POINT('',#31410);
#8096=VERTEX_POINT('',#31412);
#8097=VERTEX_POINT('',#31416);
#8098=VERTEX_POINT('',#31418);
#8099=VERTEX_POINT('',#31422);
#8100=VERTEX_POINT('',#31424);
#8101=VERTEX_POINT('',#31428);
#8102=VERTEX_POINT('',#31430);
#8103=VERTEX_POINT('',#31434);
#8104=VERTEX_POINT('',#31436);
#8105=VERTEX_POINT('',#31440);
#8106=VERTEX_POINT('',#31442);
#8107=VERTEX_POINT('',#31446);
#8108=VERTEX_POINT('',#31448);
#8109=VERTEX_POINT('',#31452);
#8110=VERTEX_POINT('',#31454);
#8111=VERTEX_POINT('',#31458);
#8112=VERTEX_POINT('',#31460);
#8113=VERTEX_POINT('',#31464);
#8114=VERTEX_POINT('',#31466);
#8115=VERTEX_POINT('',#31470);
#8116=VERTEX_POINT('',#31472);
#8117=VERTEX_POINT('',#31476);
#8118=VERTEX_POINT('',#31478);
#8119=VERTEX_POINT('',#31482);
#8120=VERTEX_POINT('',#31484);
#8121=VERTEX_POINT('',#31488);
#8122=VERTEX_POINT('',#31490);
#8123=VERTEX_POINT('',#31494);
#8124=VERTEX_POINT('',#31496);
#8125=VERTEX_POINT('',#31500);
#8126=VERTEX_POINT('',#31502);
#8127=VERTEX_POINT('',#31506);
#8128=VERTEX_POINT('',#31508);
#8129=VERTEX_POINT('',#31512);
#8130=VERTEX_POINT('',#31514);
#8131=VERTEX_POINT('',#31518);
#8132=VERTEX_POINT('',#31520);
#8133=VERTEX_POINT('',#31524);
#8134=VERTEX_POINT('',#31526);
#8135=VERTEX_POINT('',#31530);
#8136=VERTEX_POINT('',#31532);
#8137=VERTEX_POINT('',#31536);
#8138=VERTEX_POINT('',#31538);
#8139=VERTEX_POINT('',#31542);
#8140=VERTEX_POINT('',#31544);
#8141=VERTEX_POINT('',#31548);
#8142=VERTEX_POINT('',#31550);
#8143=VERTEX_POINT('',#31554);
#8144=VERTEX_POINT('',#31556);
#8145=VERTEX_POINT('',#31560);
#8146=VERTEX_POINT('',#31562);
#8147=VERTEX_POINT('',#31566);
#8148=VERTEX_POINT('',#31568);
#8149=VERTEX_POINT('',#31572);
#8150=VERTEX_POINT('',#31574);
#8151=VERTEX_POINT('',#31578);
#8152=VERTEX_POINT('',#31580);
#8153=VERTEX_POINT('',#31584);
#8154=VERTEX_POINT('',#31586);
#8155=VERTEX_POINT('',#31590);
#8156=VERTEX_POINT('',#31592);
#8157=VERTEX_POINT('',#31596);
#8158=VERTEX_POINT('',#31598);
#8159=VERTEX_POINT('',#31602);
#8160=VERTEX_POINT('',#31604);
#8161=VERTEX_POINT('',#31608);
#8162=VERTEX_POINT('',#31610);
#8163=VERTEX_POINT('',#31614);
#8164=VERTEX_POINT('',#31616);
#8165=VERTEX_POINT('',#31620);
#8166=VERTEX_POINT('',#31622);
#8167=VERTEX_POINT('',#31626);
#8168=VERTEX_POINT('',#31628);
#8169=VERTEX_POINT('',#31632);
#8170=VERTEX_POINT('',#31634);
#8171=VERTEX_POINT('',#31638);
#8172=VERTEX_POINT('',#31640);
#8173=VERTEX_POINT('',#31644);
#8174=VERTEX_POINT('',#31646);
#8175=VERTEX_POINT('',#31650);
#8176=VERTEX_POINT('',#31652);
#8177=VERTEX_POINT('',#31656);
#8178=VERTEX_POINT('',#31658);
#8179=VERTEX_POINT('',#31662);
#8180=VERTEX_POINT('',#31664);
#8181=VERTEX_POINT('',#31668);
#8182=VERTEX_POINT('',#31670);
#8183=VERTEX_POINT('',#31674);
#8184=VERTEX_POINT('',#31676);
#8185=VERTEX_POINT('',#31680);
#8186=VERTEX_POINT('',#31682);
#8187=VERTEX_POINT('',#31686);
#8188=VERTEX_POINT('',#31688);
#8189=VERTEX_POINT('',#31692);
#8190=VERTEX_POINT('',#31694);
#8191=VERTEX_POINT('',#31698);
#8192=VERTEX_POINT('',#31700);
#8193=VERTEX_POINT('',#31704);
#8194=VERTEX_POINT('',#31706);
#8195=VERTEX_POINT('',#31710);
#8196=VERTEX_POINT('',#31712);
#8197=VERTEX_POINT('',#31716);
#8198=VERTEX_POINT('',#31718);
#8199=VERTEX_POINT('',#31722);
#8200=VERTEX_POINT('',#31724);
#8201=VERTEX_POINT('',#31728);
#8202=VERTEX_POINT('',#31730);
#8203=VERTEX_POINT('',#31734);
#8204=VERTEX_POINT('',#31736);
#8205=VERTEX_POINT('',#31740);
#8206=VERTEX_POINT('',#31742);
#8207=VERTEX_POINT('',#31746);
#8208=VERTEX_POINT('',#31748);
#8209=VERTEX_POINT('',#31752);
#8210=VERTEX_POINT('',#31754);
#8211=VERTEX_POINT('',#31758);
#8212=VERTEX_POINT('',#31760);
#8213=VERTEX_POINT('',#31764);
#8214=VERTEX_POINT('',#31766);
#8215=VERTEX_POINT('',#31770);
#8216=VERTEX_POINT('',#31772);
#8217=VERTEX_POINT('',#31776);
#8218=VERTEX_POINT('',#31778);
#8219=VERTEX_POINT('',#31782);
#8220=VERTEX_POINT('',#31784);
#8221=VERTEX_POINT('',#31788);
#8222=VERTEX_POINT('',#31790);
#8223=VERTEX_POINT('',#31794);
#8224=VERTEX_POINT('',#31796);
#8225=VERTEX_POINT('',#31800);
#8226=VERTEX_POINT('',#31802);
#8227=VERTEX_POINT('',#31806);
#8228=VERTEX_POINT('',#31808);
#8229=VERTEX_POINT('',#31812);
#8230=VERTEX_POINT('',#31814);
#8231=VERTEX_POINT('',#31818);
#8232=VERTEX_POINT('',#31820);
#8233=VERTEX_POINT('',#31824);
#8234=VERTEX_POINT('',#31826);
#8235=VERTEX_POINT('',#31830);
#8236=VERTEX_POINT('',#31832);
#8237=VERTEX_POINT('',#31842);
#8238=VERTEX_POINT('',#31845);
#8239=VERTEX_POINT('',#31848);
#8240=VERTEX_POINT('',#31849);
#8241=VERTEX_POINT('',#32893);
#8242=VERTEX_POINT('',#32949);
#8243=VERTEX_POINT('',#32953);
#8244=VERTEX_POINT('',#32957);
#8245=VERTEX_POINT('',#32961);
#8246=VERTEX_POINT('',#32963);
#9972=EDGE_CURVE('',#7849,#7850,#4449,.T.);
#9973=EDGE_CURVE('',#7851,#7850,#4450,.T.);
#9974=EDGE_CURVE('',#7851,#7852,#1361,.T.);
#9975=EDGE_CURVE('',#7852,#7849,#286,.F.);
#9976=EDGE_CURVE('',#7853,#7854,#4451,.T.);
#9977=EDGE_CURVE('',#7850,#7854,#287,.T.);
#9978=EDGE_CURVE('',#7849,#7853,#288,.F.);
#9979=EDGE_CURVE('',#7855,#7856,#4452,.T.);
#9980=EDGE_CURVE('',#7854,#7856,#289,.T.);
#9981=EDGE_CURVE('',#7853,#7855,#290,.F.);
#9982=EDGE_CURVE('',#7857,#7858,#4453,.T.);
#9983=EDGE_CURVE('',#7856,#7858,#291,.T.);
#9984=EDGE_CURVE('',#7855,#7857,#292,.F.);
#9985=EDGE_CURVE('',#7859,#7860,#4454,.T.);
#9986=EDGE_CURVE('',#7858,#7860,#293,.T.);
#9987=EDGE_CURVE('',#7857,#7859,#294,.F.);
#9988=EDGE_CURVE('',#7861,#7862,#4455,.T.);
#9989=EDGE_CURVE('',#7860,#7862,#295,.T.);
#9990=EDGE_CURVE('',#7859,#7861,#296,.F.);
#9991=EDGE_CURVE('',#7863,#7864,#4456,.T.);
#9992=EDGE_CURVE('',#7862,#7864,#297,.T.);
#9993=EDGE_CURVE('',#7861,#7863,#298,.F.);
#9994=EDGE_CURVE('',#7865,#7866,#4457,.T.);
#9995=EDGE_CURVE('',#7864,#7866,#299,.T.);
#9996=EDGE_CURVE('',#7863,#7865,#300,.F.);
#9997=EDGE_CURVE('',#7867,#7868,#4458,.T.);
#9998=EDGE_CURVE('',#7866,#7868,#301,.T.);
#9999=EDGE_CURVE('',#7865,#7867,#302,.F.);
#10000=EDGE_CURVE('',#7869,#7870,#4459,.T.);
#10001=EDGE_CURVE('',#7868,#7870,#303,.T.);
#10002=EDGE_CURVE('',#7867,#7869,#304,.F.);
#10003=EDGE_CURVE('',#7871,#7872,#4460,.T.);
#10004=EDGE_CURVE('',#7870,#7872,#305,.T.);
#10005=EDGE_CURVE('',#7869,#7871,#306,.F.);
#10006=EDGE_CURVE('',#7873,#7874,#4461,.T.);
#10007=EDGE_CURVE('',#7872,#7874,#307,.T.);
#10008=EDGE_CURVE('',#7871,#7873,#308,.F.);
#10009=EDGE_CURVE('',#7875,#7876,#4462,.T.);
#10010=EDGE_CURVE('',#7874,#7876,#309,.T.);
#10011=EDGE_CURVE('',#7873,#7875,#310,.F.);
#10012=EDGE_CURVE('',#7877,#7878,#4463,.T.);
#10013=EDGE_CURVE('',#7876,#7878,#311,.T.);
#10014=EDGE_CURVE('',#7875,#7877,#312,.F.);
#10015=EDGE_CURVE('',#7879,#7880,#4464,.T.);
#10016=EDGE_CURVE('',#7878,#7880,#313,.T.);
#10017=EDGE_CURVE('',#7877,#7879,#314,.F.);
#10018=EDGE_CURVE('',#7881,#7882,#4465,.T.);
#10019=EDGE_CURVE('',#7880,#7882,#315,.T.);
#10020=EDGE_CURVE('',#7879,#7881,#316,.F.);
#10021=EDGE_CURVE('',#7883,#7884,#4466,.T.);
#10022=EDGE_CURVE('',#7882,#7884,#317,.T.);
#10023=EDGE_CURVE('',#7881,#7883,#318,.F.);
#10024=EDGE_CURVE('',#7885,#7886,#4467,.T.);
#10025=EDGE_CURVE('',#7884,#7886,#319,.T.);
#10026=EDGE_CURVE('',#7883,#7885,#320,.F.);
#10027=EDGE_CURVE('',#7887,#7888,#4468,.T.);
#10028=EDGE_CURVE('',#7887,#7889,#321,.F.);
#10029=EDGE_CURVE('',#7889,#7890,#1362,.T.);
#10030=EDGE_CURVE('',#7888,#7890,#322,.T.);
#10031=EDGE_CURVE('',#7891,#7892,#4469,.T.);
#10032=EDGE_CURVE('',#7891,#7889,#1363,.T.);
#10033=EDGE_CURVE('',#7889,#7893,#429,.T.);
#10034=EDGE_CURVE('',#7894,#7893,#4470,.T.);
#10035=EDGE_CURVE('',#7892,#7894,#59,.T.);
#10036=EDGE_CURVE('',#7895,#7896,#4471,.T.);
#10037=EDGE_CURVE('',#7896,#7897,#60,.T.);
#10038=EDGE_CURVE('',#7898,#7897,#4472,.T.);
#10039=EDGE_CURVE('',#7895,#7898,#61,.T.);
#10040=EDGE_CURVE('',#7899,#7900,#4473,.T.);
#10041=EDGE_CURVE('',#7900,#7896,#62,.T.);
#10042=EDGE_CURVE('',#7899,#7895,#63,.T.);
#10043=EDGE_CURVE('',#7901,#7902,#4474,.T.);
#10044=EDGE_CURVE('',#7902,#7900,#64,.T.);
#10045=EDGE_CURVE('',#7901,#7899,#65,.T.);
#10046=EDGE_CURVE('',#7903,#7904,#4475,.T.);
#10047=EDGE_CURVE('',#7904,#7902,#66,.T.);
#10048=EDGE_CURVE('',#7903,#7901,#67,.T.);
#10049=EDGE_CURVE('',#7905,#7906,#4476,.T.);
#10050=EDGE_CURVE('',#7906,#7904,#68,.T.);
#10051=EDGE_CURVE('',#7905,#7903,#69,.T.);
#10052=EDGE_CURVE('',#7907,#7908,#4477,.T.);
#10053=EDGE_CURVE('',#7908,#7906,#70,.T.);
#10054=EDGE_CURVE('',#7907,#7905,#71,.T.);
#10055=EDGE_CURVE('',#7909,#7910,#4478,.T.);
#10056=EDGE_CURVE('',#7910,#7908,#72,.T.);
#10057=EDGE_CURVE('',#7909,#7907,#73,.T.);
#10058=EDGE_CURVE('',#7911,#7912,#4479,.T.);
#10059=EDGE_CURVE('',#7912,#7910,#74,.T.);
#10060=EDGE_CURVE('',#7911,#7909,#75,.T.);
#10061=EDGE_CURVE('',#7913,#7914,#4480,.T.);
#10062=EDGE_CURVE('',#7914,#7912,#76,.T.);
#10063=EDGE_CURVE('',#7913,#7911,#77,.T.);
#10064=EDGE_CURVE('',#7915,#7916,#4481,.T.);
#10065=EDGE_CURVE('',#7916,#7914,#78,.T.);
#10066=EDGE_CURVE('',#7915,#7913,#79,.T.);
#10067=EDGE_CURVE('',#7917,#7918,#4482,.T.);
#10068=EDGE_CURVE('',#7918,#7916,#80,.T.);
#10069=EDGE_CURVE('',#7917,#7915,#81,.T.);
#10070=EDGE_CURVE('',#7919,#7920,#4483,.T.);
#10071=EDGE_CURVE('',#7920,#7918,#82,.T.);
#10072=EDGE_CURVE('',#7919,#7917,#83,.T.);
#10073=EDGE_CURVE('',#7921,#7922,#4484,.T.);
#10074=EDGE_CURVE('',#7922,#7920,#84,.T.);
#10075=EDGE_CURVE('',#7921,#7919,#85,.T.);
#10076=EDGE_CURVE('',#7923,#7924,#4485,.T.);
#10077=EDGE_CURVE('',#7924,#7922,#86,.T.);
#10078=EDGE_CURVE('',#7923,#7921,#87,.T.);
#10079=EDGE_CURVE('',#7925,#7926,#4486,.T.);
#10080=EDGE_CURVE('',#7926,#7924,#88,.T.);
#10081=EDGE_CURVE('',#7925,#7923,#89,.T.);
#10082=EDGE_CURVE('',#7927,#7928,#4487,.T.);
#10083=EDGE_CURVE('',#7928,#7926,#90,.T.);
#10084=EDGE_CURVE('',#7927,#7925,#91,.T.);
#10085=EDGE_CURVE('',#7929,#7930,#4488,.T.);
#10086=EDGE_CURVE('',#7930,#7928,#92,.T.);
#10087=EDGE_CURVE('',#7929,#7927,#93,.T.);
#10088=EDGE_CURVE('',#7931,#7932,#4489,.T.);
#10089=EDGE_CURVE('',#7932,#7930,#94,.T.);
#10090=EDGE_CURVE('',#7931,#7929,#95,.T.);
#10091=EDGE_CURVE('',#7933,#7934,#4490,.T.);
#10092=EDGE_CURVE('',#7934,#7932,#96,.T.);
#10093=EDGE_CURVE('',#7933,#7931,#97,.T.);
#10094=EDGE_CURVE('',#7935,#7936,#4491,.T.);
#10095=EDGE_CURVE('',#7937,#7935,#98,.T.);
#10096=EDGE_CURVE('',#7938,#7937,#4492,.T.);
#10097=EDGE_CURVE('',#7938,#7936,#99,.T.);
#10098=EDGE_CURVE('',#7939,#7940,#4493,.T.);
#10099=EDGE_CURVE('',#7941,#7939,#323,.T.);
#10100=EDGE_CURVE('',#7941,#7942,#1364,.T.);
#10101=EDGE_CURVE('',#7942,#7940,#324,.F.);
#10102=EDGE_CURVE('',#7943,#7944,#4494,.T.);
#10103=EDGE_CURVE('',#7939,#7943,#325,.T.);
#10104=EDGE_CURVE('',#7940,#7944,#326,.F.);
#10105=EDGE_CURVE('',#7945,#7946,#4495,.T.);
#10106=EDGE_CURVE('',#7943,#7945,#327,.T.);
#10107=EDGE_CURVE('',#7944,#7946,#328,.F.);
#10108=EDGE_CURVE('',#7947,#7948,#4496,.T.);
#10109=EDGE_CURVE('',#7947,#7949,#100,.T.);
#10110=EDGE_CURVE('',#7949,#7950,#4497,.T.);
#10111=EDGE_CURVE('',#7948,#7950,#101,.T.);
#10112=EDGE_CURVE('',#7951,#7952,#4498,.T.);
#10113=EDGE_CURVE('',#7951,#7947,#102,.T.);
#10114=EDGE_CURVE('',#7952,#7948,#103,.T.);
#10115=EDGE_CURVE('',#7953,#7954,#4499,.T.);
#10116=EDGE_CURVE('',#7953,#7951,#104,.T.);
#10117=EDGE_CURVE('',#7954,#7952,#105,.T.);
#10118=EDGE_CURVE('',#7955,#7956,#4500,.T.);
#10119=EDGE_CURVE('',#7955,#7953,#106,.T.);
#10120=EDGE_CURVE('',#7956,#7954,#107,.T.);
#10121=EDGE_CURVE('',#7957,#7958,#4501,.T.);
#10122=EDGE_CURVE('',#7957,#7955,#108,.T.);
#10123=EDGE_CURVE('',#7958,#7956,#109,.T.);
#10124=EDGE_CURVE('',#7959,#7960,#4502,.T.);
#10125=EDGE_CURVE('',#7959,#7957,#110,.T.);
#10126=EDGE_CURVE('',#7960,#7958,#111,.T.);
#10127=EDGE_CURVE('',#7961,#7962,#4503,.T.);
#10128=EDGE_CURVE('',#7961,#7959,#112,.T.);
#10129=EDGE_CURVE('',#7962,#7960,#113,.T.);
#10130=EDGE_CURVE('',#7963,#7964,#4504,.T.);
#10131=EDGE_CURVE('',#7963,#7961,#114,.T.);
#10132=EDGE_CURVE('',#7964,#7962,#115,.T.);
#10133=EDGE_CURVE('',#7965,#7966,#4505,.T.);
#10134=EDGE_CURVE('',#7966,#7967,#329,.T.);
#10135=EDGE_CURVE('',#7967,#7968,#1365,.T.);
#10136=EDGE_CURVE('',#7968,#7965,#330,.T.);
#10137=EDGE_CURVE('',#7969,#7970,#4506,.T.);
#10138=EDGE_CURVE('',#7970,#7966,#331,.T.);
#10139=EDGE_CURVE('',#7965,#7969,#332,.T.);
#10140=EDGE_CURVE('',#7971,#7972,#4507,.T.);
#10141=EDGE_CURVE('',#7972,#7970,#333,.T.);
#10142=EDGE_CURVE('',#7969,#7971,#334,.T.);
#10143=EDGE_CURVE('',#7973,#7974,#4508,.T.);
#10144=EDGE_CURVE('',#7973,#7975,#335,.T.);
#10145=EDGE_CURVE('',#7976,#7975,#4509,.T.);
#10146=EDGE_CURVE('',#7976,#7974,#336,.T.);
#10147=EDGE_CURVE('',#7974,#7972,#337,.T.);
#10148=EDGE_CURVE('',#7971,#7973,#338,.T.);
#10149=EDGE_CURVE('',#7977,#7978,#1366,.T.);
#10150=EDGE_CURVE('',#7979,#7978,#4510,.T.);
#10151=EDGE_CURVE('',#7980,#7979,#4511,.T.);
#10152=EDGE_CURVE('',#7977,#7980,#4512,.T.);
#10153=EDGE_CURVE('',#7981,#7982,#116,.T.);
#10154=EDGE_CURVE('',#7982,#7980,#4513,.T.);
#10155=EDGE_CURVE('',#7981,#7979,#4514,.T.);
#10156=EDGE_CURVE('',#7983,#7981,#117,.T.);
#10157=EDGE_CURVE('',#7978,#7984,#4515,.T.);
#10158=EDGE_CURVE('',#7984,#7983,#4516,.T.);
#10159=EDGE_CURVE('',#7982,#7985,#118,.T.);
#10160=EDGE_CURVE('',#7985,#7986,#4517,.T.);
#10161=EDGE_CURVE('',#7986,#7977,#4518,.T.);
#10162=EDGE_CURVE('',#7987,#7988,#4519,.T.);
#10163=EDGE_CURVE('',#7989,#7987,#4520,.T.);
#10164=EDGE_CURVE('',#7990,#7989,#4521,.T.);
#10165=EDGE_CURVE('',#7988,#7990,#1367,.T.);
#10166=EDGE_CURVE('',#7991,#7992,#119,.T.);
#10167=EDGE_CURVE('',#7992,#7993,#4522,.T.);
#10168=EDGE_CURVE('',#7993,#7990,#4523,.T.);
#10169=EDGE_CURVE('',#7991,#7989,#4524,.T.);
#10170=EDGE_CURVE('',#7994,#7991,#120,.T.);
#10171=EDGE_CURVE('',#7994,#7987,#4525,.T.);
#10172=EDGE_CURVE('',#7995,#7994,#121,.T.);
#10173=EDGE_CURVE('',#7988,#7996,#4526,.T.);
#10174=EDGE_CURVE('',#7996,#7995,#4527,.T.);
#10175=EDGE_CURVE('',#7997,#7998,#4528,.T.);
#10176=EDGE_CURVE('',#7999,#7997,#4529,.T.);
#10177=EDGE_CURVE('',#8000,#7999,#4530,.T.);
#10178=EDGE_CURVE('',#7998,#8000,#1368,.T.);
#10179=EDGE_CURVE('',#8001,#8002,#122,.T.);
#10180=EDGE_CURVE('',#8002,#8003,#4531,.T.);
#10181=EDGE_CURVE('',#8003,#8000,#4532,.T.);
#10182=EDGE_CURVE('',#8001,#7999,#4533,.T.);
#10183=EDGE_CURVE('',#8004,#8001,#123,.T.);
#10184=EDGE_CURVE('',#8004,#7997,#4534,.T.);
#10185=EDGE_CURVE('',#8005,#8004,#124,.T.);
#10186=EDGE_CURVE('',#7998,#8006,#4535,.T.);
#10187=EDGE_CURVE('',#8006,#8005,#4536,.T.);
#10188=EDGE_CURVE('',#8007,#8008,#4537,.T.);
#10189=EDGE_CURVE('',#8009,#8007,#4538,.T.);
#10190=EDGE_CURVE('',#8010,#8009,#4539,.T.);
#10191=EDGE_CURVE('',#8011,#8010,#1369,.T.);
#10192=EDGE_CURVE('',#8008,#8011,#1370,.T.);
#10193=EDGE_CURVE('',#8012,#8013,#125,.T.);
#10194=EDGE_CURVE('',#8013,#8014,#4540,.T.);
#10195=EDGE_CURVE('',#8014,#8010,#4541,.T.);
#10196=EDGE_CURVE('',#8012,#8009,#4542,.T.);
#10197=EDGE_CURVE('',#8015,#8016,#126,.T.);
#10198=EDGE_CURVE('',#8016,#8012,#127,.T.);
#10199=EDGE_CURVE('',#8015,#8007,#4543,.T.);
#10200=EDGE_CURVE('',#8017,#8015,#128,.T.);
#10201=EDGE_CURVE('',#8008,#8018,#4544,.T.);
#10202=EDGE_CURVE('',#8018,#8017,#4545,.T.);
#10203=EDGE_CURVE('',#7993,#7984,#1371,.T.);
#10204=EDGE_CURVE('',#7992,#7983,#1372,.T.);
#10205=EDGE_CURVE('',#7990,#7978,#1373,.T.);
#10206=EDGE_CURVE('',#8019,#8019,#1374,.T.);
#10207=EDGE_CURVE('',#8019,#8011,#4546,.T.);
#10208=EDGE_CURVE('',#8010,#7998,#1375,.T.);
#10209=EDGE_CURVE('',#8000,#7988,#1376,.T.);
#10210=EDGE_CURVE('',#7977,#8008,#1377,.T.);
#10211=EDGE_CURVE('',#7942,#7967,#339,.T.);
#10212=EDGE_CURVE('',#7968,#7941,#340,.T.);
#10213=EDGE_CURVE('',#8020,#8020,#1378,.T.);
#10214=EDGE_CURVE('',#8020,#8021,#4547,.T.);
#10215=EDGE_CURVE('',#8021,#8021,#1379,.T.);
#10216=EDGE_CURVE('',#8022,#8022,#1380,.T.);
#10217=EDGE_CURVE('',#8022,#8020,#1381,.T.);
#10218=EDGE_CURVE('',#8002,#7995,#1382,.T.);
#10219=EDGE_CURVE('',#8013,#8005,#1383,.T.);
#10220=EDGE_CURVE('',#8016,#8022,#4548,.T.);
#10221=EDGE_CURVE('',#7985,#8017,#1384,.T.);
#10222=EDGE_CURVE('',#8014,#8006,#1385,.T.);
#10223=EDGE_CURVE('',#8003,#7996,#1386,.T.);
#10224=EDGE_CURVE('',#7986,#8018,#1387,.T.);
#10225=EDGE_CURVE('',#7976,#8023,#4549,.T.);
#10226=EDGE_CURVE('',#8023,#7964,#129,.T.);
#10227=EDGE_CURVE('',#7950,#8024,#4550,.T.);
#10228=EDGE_CURVE('',#8025,#8024,#130,.T.);
#10229=EDGE_CURVE('',#7946,#8025,#341,.F.);
#10230=EDGE_CURVE('',#7945,#8026,#342,.T.);
#10231=EDGE_CURVE('',#8026,#7949,#4551,.T.);
#10232=EDGE_CURVE('',#8027,#7963,#131,.T.);
#10233=EDGE_CURVE('',#8027,#7975,#4552,.T.);
#10234=EDGE_CURVE('',#8023,#8027,#4553,.T.);
#10235=EDGE_CURVE('',#8028,#8028,#1388,.T.);
#10236=EDGE_CURVE('',#8029,#8029,#1389,.T.);
#10237=EDGE_CURVE('',#8029,#8030,#4554,.T.);
#10238=EDGE_CURVE('',#8030,#8030,#1390,.T.);
#10239=EDGE_CURVE('',#8024,#8026,#4555,.T.);
#10240=EDGE_CURVE('',#8026,#8025,#1391,.T.);
#10241=EDGE_CURVE('',#8030,#8028,#1392,.T.);
#10242=EDGE_CURVE('',#8031,#8031,#1393,.T.);
#10243=EDGE_CURVE('',#8031,#8032,#1394,.T.);
#10244=EDGE_CURVE('',#8033,#8032,#1395,.T.);
#10245=EDGE_CURVE('',#8032,#8033,#1396,.T.);
#10246=EDGE_CURVE('',#8034,#8034,#1397,.T.);
#10247=EDGE_CURVE('',#8034,#8035,#4556,.T.);
#10248=EDGE_CURVE('',#8035,#8035,#1398,.T.);
#10249=EDGE_CURVE('',#8036,#8036,#1399,.T.);
#10250=EDGE_CURVE('',#8036,#8037,#4557,.T.);
#10251=EDGE_CURVE('',#8037,#8037,#1400,.T.);
#10252=EDGE_CURVE('',#8038,#8038,#1401,.T.);
#10253=EDGE_CURVE('',#8039,#8040,#1402,.T.);
#10254=EDGE_CURVE('',#8040,#8041,#1403,.T.);
#10255=EDGE_CURVE('',#8041,#8042,#1404,.T.);
#10256=EDGE_CURVE('',#8042,#8043,#1405,.T.);
#10257=EDGE_CURVE('',#8043,#8044,#1406,.T.);
#10258=EDGE_CURVE('',#8044,#8033,#4558,.T.);
#10259=EDGE_CURVE('',#8044,#8045,#1407,.T.);
#10260=EDGE_CURVE('',#8045,#8046,#1408,.T.);
#10261=EDGE_CURVE('',#8046,#8047,#1409,.T.);
#10262=EDGE_CURVE('',#8047,#8039,#1410,.T.);
#10263=EDGE_CURVE('',#8025,#8026,#1411,.T.);
#10264=EDGE_CURVE('',#8043,#8048,#1412,.T.);
#10265=EDGE_CURVE('',#8048,#8045,#1413,.T.);
#10266=EDGE_CURVE('',#8041,#8042,#1414,.T.);
#10267=EDGE_CURVE('',#8039,#8040,#1415,.T.);
#10268=EDGE_CURVE('',#8046,#8047,#1416,.T.);
#10269=EDGE_CURVE('',#8049,#8049,#1417,.T.);
#10270=EDGE_CURVE('',#8049,#8048,#4559,.T.);
#10271=EDGE_CURVE('',#8045,#8043,#1418,.T.);
#10272=EDGE_CURVE('',#8050,#8050,#1419,.T.);
#10273=EDGE_CURVE('',#8050,#8051,#4560,.T.);
#10274=EDGE_CURVE('',#8042,#8051,#1420,.T.);
#10275=EDGE_CURVE('',#8051,#8041,#1421,.T.);
#10276=EDGE_CURVE('',#8052,#8052,#1422,.T.);
#10277=EDGE_CURVE('',#8052,#8053,#4561,.T.);
#10278=EDGE_CURVE('',#8040,#8053,#1423,.T.);
#10279=EDGE_CURVE('',#8053,#8039,#1424,.T.);
#10280=EDGE_CURVE('',#8054,#8054,#1425,.T.);
#10281=EDGE_CURVE('',#8054,#8055,#4562,.T.);
#10282=EDGE_CURVE('',#8047,#8055,#1426,.T.);
#10283=EDGE_CURVE('',#8055,#8046,#1427,.T.);
#10284=EDGE_CURVE('',#8038,#8056,#4563,.T.);
#10285=EDGE_CURVE('',#8056,#8056,#1428,.T.);
#10286=EDGE_CURVE('',#8057,#8058,#4564,.T.);
#10287=EDGE_CURVE('',#8059,#8058,#4565,.T.);
#10288=EDGE_CURVE('',#8060,#8059,#4566,.T.);
#10289=EDGE_CURVE('',#8060,#8057,#4567,.T.);
#10290=EDGE_CURVE('',#8061,#8057,#4568,.T.);
#10291=EDGE_CURVE('',#8062,#8060,#4569,.T.);
#10292=EDGE_CURVE('',#8062,#8061,#4570,.T.);
#10293=EDGE_CURVE('',#8063,#8061,#4571,.T.);
#10294=EDGE_CURVE('',#8064,#8062,#4572,.T.);
#10295=EDGE_CURVE('',#8064,#8063,#4573,.T.);
#10296=EDGE_CURVE('',#8065,#8063,#4574,.T.);
#10297=EDGE_CURVE('',#8066,#8064,#4575,.T.);
#10298=EDGE_CURVE('',#8066,#8065,#4576,.T.);
#10299=EDGE_CURVE('',#8067,#8065,#4577,.T.);
#10300=EDGE_CURVE('',#8068,#8066,#4578,.T.);
#10301=EDGE_CURVE('',#8068,#8067,#4579,.T.);
#10302=EDGE_CURVE('',#8069,#8067,#4580,.T.);
#10303=EDGE_CURVE('',#8070,#8068,#4581,.T.);
#10304=EDGE_CURVE('',#8070,#8069,#4582,.T.);
#10305=EDGE_CURVE('',#8071,#8069,#4583,.T.);
#10306=EDGE_CURVE('',#8072,#8070,#4584,.T.);
#10307=EDGE_CURVE('',#8072,#8071,#4585,.T.);
#10308=EDGE_CURVE('',#8073,#8071,#4586,.T.);
#10309=EDGE_CURVE('',#8074,#8072,#4587,.T.);
#10310=EDGE_CURVE('',#8074,#8073,#4588,.T.);
#10311=EDGE_CURVE('',#8075,#8073,#4589,.T.);
#10312=EDGE_CURVE('',#8076,#8074,#4590,.T.);
#10313=EDGE_CURVE('',#8076,#8075,#4591,.T.);
#10314=EDGE_CURVE('',#8077,#8075,#4592,.T.);
#10315=EDGE_CURVE('',#8078,#8076,#4593,.T.);
#10316=EDGE_CURVE('',#8078,#8077,#4594,.T.);
#10317=EDGE_CURVE('',#8079,#8077,#4595,.T.);
#10318=EDGE_CURVE('',#8080,#8078,#4596,.T.);
#10319=EDGE_CURVE('',#8080,#8079,#4597,.T.);
#10320=EDGE_CURVE('',#8081,#8079,#4598,.T.);
#10321=EDGE_CURVE('',#8082,#8080,#4599,.T.);
#10322=EDGE_CURVE('',#8082,#8081,#4600,.T.);
#10323=EDGE_CURVE('',#8083,#8081,#4601,.T.);
#10324=EDGE_CURVE('',#8084,#8082,#4602,.T.);
#10325=EDGE_CURVE('',#8084,#8083,#4603,.T.);
#10326=EDGE_CURVE('',#8085,#8083,#4604,.T.);
#10327=EDGE_CURVE('',#8086,#8084,#4605,.T.);
#10328=EDGE_CURVE('',#8086,#8085,#4606,.T.);
#10329=EDGE_CURVE('',#8087,#8085,#4607,.T.);
#10330=EDGE_CURVE('',#8088,#8086,#4608,.T.);
#10331=EDGE_CURVE('',#8088,#8087,#4609,.T.);
#10332=EDGE_CURVE('',#8089,#8087,#4610,.T.);
#10333=EDGE_CURVE('',#8090,#8088,#4611,.T.);
#10334=EDGE_CURVE('',#8090,#8089,#4612,.T.);
#10335=EDGE_CURVE('',#8091,#8089,#4613,.T.);
#10336=EDGE_CURVE('',#8092,#8090,#4614,.T.);
#10337=EDGE_CURVE('',#8092,#8091,#4615,.T.);
#10338=EDGE_CURVE('',#8093,#8091,#4616,.T.);
#10339=EDGE_CURVE('',#8094,#8092,#4617,.T.);
#10340=EDGE_CURVE('',#8094,#8093,#4618,.T.);
#10341=EDGE_CURVE('',#8095,#8093,#4619,.T.);
#10342=EDGE_CURVE('',#8096,#8094,#4620,.T.);
#10343=EDGE_CURVE('',#8096,#8095,#4621,.T.);
#10344=EDGE_CURVE('',#8097,#8095,#4622,.T.);
#10345=EDGE_CURVE('',#8098,#8096,#4623,.T.);
#10346=EDGE_CURVE('',#8098,#8097,#4624,.T.);
#10347=EDGE_CURVE('',#8099,#8097,#4625,.T.);
#10348=EDGE_CURVE('',#8100,#8098,#4626,.T.);
#10349=EDGE_CURVE('',#8100,#8099,#4627,.T.);
#10350=EDGE_CURVE('',#8101,#8099,#4628,.T.);
#10351=EDGE_CURVE('',#8102,#8100,#4629,.T.);
#10352=EDGE_CURVE('',#8102,#8101,#4630,.T.);
#10353=EDGE_CURVE('',#8103,#8101,#4631,.T.);
#10354=EDGE_CURVE('',#8104,#8102,#4632,.T.);
#10355=EDGE_CURVE('',#8104,#8103,#4633,.T.);
#10356=EDGE_CURVE('',#8105,#8103,#4634,.T.);
#10357=EDGE_CURVE('',#8106,#8104,#4635,.T.);
#10358=EDGE_CURVE('',#8106,#8105,#4636,.T.);
#10359=EDGE_CURVE('',#8107,#8105,#4637,.T.);
#10360=EDGE_CURVE('',#8108,#8106,#4638,.T.);
#10361=EDGE_CURVE('',#8108,#8107,#4639,.T.);
#10362=EDGE_CURVE('',#8109,#8107,#4640,.T.);
#10363=EDGE_CURVE('',#8110,#8108,#4641,.T.);
#10364=EDGE_CURVE('',#8110,#8109,#4642,.T.);
#10365=EDGE_CURVE('',#8111,#8109,#4643,.T.);
#10366=EDGE_CURVE('',#8112,#8110,#4644,.T.);
#10367=EDGE_CURVE('',#8112,#8111,#4645,.T.);
#10368=EDGE_CURVE('',#8113,#8111,#4646,.T.);
#10369=EDGE_CURVE('',#8114,#8112,#4647,.T.);
#10370=EDGE_CURVE('',#8114,#8113,#4648,.T.);
#10371=EDGE_CURVE('',#8115,#8113,#4649,.T.);
#10372=EDGE_CURVE('',#8116,#8114,#4650,.T.);
#10373=EDGE_CURVE('',#8116,#8115,#4651,.T.);
#10374=EDGE_CURVE('',#8117,#8115,#4652,.T.);
#10375=EDGE_CURVE('',#8118,#8116,#4653,.T.);
#10376=EDGE_CURVE('',#8118,#8117,#4654,.T.);
#10377=EDGE_CURVE('',#8119,#8117,#4655,.T.);
#10378=EDGE_CURVE('',#8120,#8118,#4656,.T.);
#10379=EDGE_CURVE('',#8120,#8119,#4657,.T.);
#10380=EDGE_CURVE('',#8121,#8119,#4658,.T.);
#10381=EDGE_CURVE('',#8122,#8120,#4659,.T.);
#10382=EDGE_CURVE('',#8122,#8121,#4660,.T.);
#10383=EDGE_CURVE('',#8123,#8121,#4661,.T.);
#10384=EDGE_CURVE('',#8124,#8122,#4662,.T.);
#10385=EDGE_CURVE('',#8124,#8123,#4663,.T.);
#10386=EDGE_CURVE('',#8125,#8123,#4664,.T.);
#10387=EDGE_CURVE('',#8126,#8124,#4665,.T.);
#10388=EDGE_CURVE('',#8126,#8125,#4666,.T.);
#10389=EDGE_CURVE('',#8127,#8125,#4667,.T.);
#10390=EDGE_CURVE('',#8128,#8126,#4668,.T.);
#10391=EDGE_CURVE('',#8128,#8127,#4669,.T.);
#10392=EDGE_CURVE('',#8129,#8127,#4670,.T.);
#10393=EDGE_CURVE('',#8130,#8128,#4671,.T.);
#10394=EDGE_CURVE('',#8130,#8129,#4672,.T.);
#10395=EDGE_CURVE('',#8131,#8129,#4673,.T.);
#10396=EDGE_CURVE('',#8132,#8130,#4674,.T.);
#10397=EDGE_CURVE('',#8132,#8131,#4675,.T.);
#10398=EDGE_CURVE('',#8133,#8131,#4676,.T.);
#10399=EDGE_CURVE('',#8134,#8132,#4677,.T.);
#10400=EDGE_CURVE('',#8134,#8133,#4678,.T.);
#10401=EDGE_CURVE('',#8135,#8133,#4679,.T.);
#10402=EDGE_CURVE('',#8136,#8134,#4680,.T.);
#10403=EDGE_CURVE('',#8136,#8135,#4681,.T.);
#10404=EDGE_CURVE('',#8137,#8135,#4682,.T.);
#10405=EDGE_CURVE('',#8138,#8136,#4683,.T.);
#10406=EDGE_CURVE('',#8138,#8137,#4684,.T.);
#10407=EDGE_CURVE('',#8139,#8137,#4685,.T.);
#10408=EDGE_CURVE('',#8140,#8138,#4686,.T.);
#10409=EDGE_CURVE('',#8140,#8139,#4687,.T.);
#10410=EDGE_CURVE('',#8141,#8139,#4688,.T.);
#10411=EDGE_CURVE('',#8142,#8140,#4689,.T.);
#10412=EDGE_CURVE('',#8142,#8141,#4690,.T.);
#10413=EDGE_CURVE('',#8143,#8141,#4691,.T.);
#10414=EDGE_CURVE('',#8144,#8142,#4692,.T.);
#10415=EDGE_CURVE('',#8144,#8143,#4693,.T.);
#10416=EDGE_CURVE('',#8145,#8143,#4694,.T.);
#10417=EDGE_CURVE('',#8146,#8144,#4695,.T.);
#10418=EDGE_CURVE('',#8146,#8145,#4696,.T.);
#10419=EDGE_CURVE('',#8147,#8145,#4697,.T.);
#10420=EDGE_CURVE('',#8148,#8146,#4698,.T.);
#10421=EDGE_CURVE('',#8148,#8147,#4699,.T.);
#10422=EDGE_CURVE('',#8149,#8147,#4700,.T.);
#10423=EDGE_CURVE('',#8150,#8148,#4701,.T.);
#10424=EDGE_CURVE('',#8150,#8149,#4702,.T.);
#10425=EDGE_CURVE('',#8151,#8149,#4703,.T.);
#10426=EDGE_CURVE('',#8152,#8150,#4704,.T.);
#10427=EDGE_CURVE('',#8152,#8151,#4705,.T.);
#10428=EDGE_CURVE('',#8153,#8151,#4706,.T.);
#10429=EDGE_CURVE('',#8154,#8152,#4707,.T.);
#10430=EDGE_CURVE('',#8154,#8153,#4708,.T.);
#10431=EDGE_CURVE('',#8155,#8153,#4709,.T.);
#10432=EDGE_CURVE('',#8156,#8154,#4710,.T.);
#10433=EDGE_CURVE('',#8156,#8155,#4711,.T.);
#10434=EDGE_CURVE('',#8157,#8155,#4712,.T.);
#10435=EDGE_CURVE('',#8158,#8156,#4713,.T.);
#10436=EDGE_CURVE('',#8158,#8157,#4714,.T.);
#10437=EDGE_CURVE('',#8159,#8157,#4715,.T.);
#10438=EDGE_CURVE('',#8160,#8158,#4716,.T.);
#10439=EDGE_CURVE('',#8160,#8159,#4717,.T.);
#10440=EDGE_CURVE('',#8161,#8159,#4718,.T.);
#10441=EDGE_CURVE('',#8162,#8160,#4719,.T.);
#10442=EDGE_CURVE('',#8162,#8161,#4720,.T.);
#10443=EDGE_CURVE('',#8163,#8161,#4721,.T.);
#10444=EDGE_CURVE('',#8164,#8162,#4722,.T.);
#10445=EDGE_CURVE('',#8164,#8163,#4723,.T.);
#10446=EDGE_CURVE('',#8165,#8163,#4724,.T.);
#10447=EDGE_CURVE('',#8166,#8164,#4725,.T.);
#10448=EDGE_CURVE('',#8166,#8165,#4726,.T.);
#10449=EDGE_CURVE('',#8167,#8165,#4727,.T.);
#10450=EDGE_CURVE('',#8168,#8166,#4728,.T.);
#10451=EDGE_CURVE('',#8168,#8167,#4729,.T.);
#10452=EDGE_CURVE('',#8169,#8167,#4730,.T.);
#10453=EDGE_CURVE('',#8170,#8168,#4731,.T.);
#10454=EDGE_CURVE('',#8170,#8169,#4732,.T.);
#10455=EDGE_CURVE('',#8171,#8169,#4733,.T.);
#10456=EDGE_CURVE('',#8172,#8170,#4734,.T.);
#10457=EDGE_CURVE('',#8172,#8171,#4735,.T.);
#10458=EDGE_CURVE('',#8173,#8171,#4736,.T.);
#10459=EDGE_CURVE('',#8174,#8172,#4737,.T.);
#10460=EDGE_CURVE('',#8174,#8173,#4738,.T.);
#10461=EDGE_CURVE('',#8175,#8173,#4739,.T.);
#10462=EDGE_CURVE('',#8176,#8174,#4740,.T.);
#10463=EDGE_CURVE('',#8176,#8175,#4741,.T.);
#10464=EDGE_CURVE('',#8177,#8175,#4742,.T.);
#10465=EDGE_CURVE('',#8178,#8176,#4743,.T.);
#10466=EDGE_CURVE('',#8178,#8177,#4744,.T.);
#10467=EDGE_CURVE('',#8179,#8177,#4745,.T.);
#10468=EDGE_CURVE('',#8180,#8178,#4746,.T.);
#10469=EDGE_CURVE('',#8180,#8179,#4747,.T.);
#10470=EDGE_CURVE('',#8181,#8179,#4748,.T.);
#10471=EDGE_CURVE('',#8182,#8180,#4749,.T.);
#10472=EDGE_CURVE('',#8182,#8181,#4750,.T.);
#10473=EDGE_CURVE('',#8183,#8181,#4751,.T.);
#10474=EDGE_CURVE('',#8184,#8182,#4752,.T.);
#10475=EDGE_CURVE('',#8184,#8183,#4753,.T.);
#10476=EDGE_CURVE('',#8185,#8183,#4754,.T.);
#10477=EDGE_CURVE('',#8186,#8184,#4755,.T.);
#10478=EDGE_CURVE('',#8186,#8185,#4756,.T.);
#10479=EDGE_CURVE('',#8187,#8185,#4757,.T.);
#10480=EDGE_CURVE('',#8188,#8186,#4758,.T.);
#10481=EDGE_CURVE('',#8188,#8187,#4759,.T.);
#10482=EDGE_CURVE('',#8189,#8187,#4760,.T.);
#10483=EDGE_CURVE('',#8190,#8188,#4761,.T.);
#10484=EDGE_CURVE('',#8190,#8189,#4762,.T.);
#10485=EDGE_CURVE('',#8191,#8189,#4763,.T.);
#10486=EDGE_CURVE('',#8192,#8190,#4764,.T.);
#10487=EDGE_CURVE('',#8192,#8191,#4765,.T.);
#10488=EDGE_CURVE('',#8193,#8191,#4766,.T.);
#10489=EDGE_CURVE('',#8194,#8192,#4767,.T.);
#10490=EDGE_CURVE('',#8194,#8193,#4768,.T.);
#10491=EDGE_CURVE('',#8195,#8193,#4769,.T.);
#10492=EDGE_CURVE('',#8196,#8194,#4770,.T.);
#10493=EDGE_CURVE('',#8196,#8195,#4771,.T.);
#10494=EDGE_CURVE('',#8197,#8195,#4772,.T.);
#10495=EDGE_CURVE('',#8198,#8196,#4773,.T.);
#10496=EDGE_CURVE('',#8198,#8197,#4774,.T.);
#10497=EDGE_CURVE('',#8199,#8197,#4775,.T.);
#10498=EDGE_CURVE('',#8200,#8198,#4776,.T.);
#10499=EDGE_CURVE('',#8200,#8199,#4777,.T.);
#10500=EDGE_CURVE('',#8201,#8199,#4778,.T.);
#10501=EDGE_CURVE('',#8202,#8200,#4779,.T.);
#10502=EDGE_CURVE('',#8202,#8201,#4780,.T.);
#10503=EDGE_CURVE('',#8203,#8201,#4781,.T.);
#10504=EDGE_CURVE('',#8204,#8202,#4782,.T.);
#10505=EDGE_CURVE('',#8204,#8203,#4783,.T.);
#10506=EDGE_CURVE('',#8205,#8203,#4784,.T.);
#10507=EDGE_CURVE('',#8206,#8204,#4785,.T.);
#10508=EDGE_CURVE('',#8206,#8205,#4786,.T.);
#10509=EDGE_CURVE('',#8207,#8205,#4787,.T.);
#10510=EDGE_CURVE('',#8208,#8206,#4788,.T.);
#10511=EDGE_CURVE('',#8208,#8207,#4789,.T.);
#10512=EDGE_CURVE('',#8209,#8207,#4790,.T.);
#10513=EDGE_CURVE('',#8210,#8208,#4791,.T.);
#10514=EDGE_CURVE('',#8210,#8209,#4792,.T.);
#10515=EDGE_CURVE('',#8211,#8209,#4793,.T.);
#10516=EDGE_CURVE('',#8212,#8210,#4794,.T.);
#10517=EDGE_CURVE('',#8212,#8211,#4795,.T.);
#10518=EDGE_CURVE('',#8213,#8211,#4796,.T.);
#10519=EDGE_CURVE('',#8214,#8212,#4797,.T.);
#10520=EDGE_CURVE('',#8214,#8213,#4798,.T.);
#10521=EDGE_CURVE('',#8215,#8213,#4799,.T.);
#10522=EDGE_CURVE('',#8216,#8214,#4800,.T.);
#10523=EDGE_CURVE('',#8216,#8215,#4801,.T.);
#10524=EDGE_CURVE('',#8217,#8215,#4802,.T.);
#10525=EDGE_CURVE('',#8218,#8216,#4803,.T.);
#10526=EDGE_CURVE('',#8218,#8217,#4804,.T.);
#10527=EDGE_CURVE('',#8219,#8217,#4805,.T.);
#10528=EDGE_CURVE('',#8220,#8218,#4806,.T.);
#10529=EDGE_CURVE('',#8220,#8219,#4807,.T.);
#10530=EDGE_CURVE('',#8221,#8219,#4808,.T.);
#10531=EDGE_CURVE('',#8222,#8220,#4809,.T.);
#10532=EDGE_CURVE('',#8222,#8221,#4810,.T.);
#10533=EDGE_CURVE('',#8223,#8221,#4811,.T.);
#10534=EDGE_CURVE('',#8224,#8222,#4812,.T.);
#10535=EDGE_CURVE('',#8224,#8223,#4813,.T.);
#10536=EDGE_CURVE('',#8225,#8223,#4814,.T.);
#10537=EDGE_CURVE('',#8226,#8224,#4815,.T.);
#10538=EDGE_CURVE('',#8226,#8225,#4816,.T.);
#10539=EDGE_CURVE('',#8227,#8225,#4817,.T.);
#10540=EDGE_CURVE('',#8228,#8226,#4818,.T.);
#10541=EDGE_CURVE('',#8228,#8227,#4819,.T.);
#10542=EDGE_CURVE('',#8229,#8227,#4820,.T.);
#10543=EDGE_CURVE('',#8230,#8228,#4821,.T.);
#10544=EDGE_CURVE('',#8230,#8229,#4822,.T.);
#10545=EDGE_CURVE('',#8231,#8229,#4823,.T.);
#10546=EDGE_CURVE('',#8232,#8230,#4824,.T.);
#10547=EDGE_CURVE('',#8232,#8231,#4825,.T.);
#10548=EDGE_CURVE('',#8233,#8231,#4826,.T.);
#10549=EDGE_CURVE('',#8234,#8232,#4827,.T.);
#10550=EDGE_CURVE('',#8234,#8233,#4828,.T.);
#10551=EDGE_CURVE('',#8235,#8233,#4829,.T.);
#10552=EDGE_CURVE('',#8236,#8234,#4830,.T.);
#10553=EDGE_CURVE('',#8236,#8235,#4831,.T.);
#10554=EDGE_CURVE('',#8058,#8235,#4832,.T.);
#10555=EDGE_CURVE('',#8059,#8236,#4833,.T.);
#10556=EDGE_CURVE('',#8237,#8237,#1429,.T.);
#10557=EDGE_CURVE('',#8238,#8238,#1430,.T.);
#10558=EDGE_CURVE('',#8239,#8240,#1431,.T.);
#10559=EDGE_CURVE('',#8240,#8239,#1432,.T.);
#10560=EDGE_CURVE('',#8239,#8237,#4834,.T.);
#10561=EDGE_CURVE('',#7850,#7938,#4835,.T.);
#10562=EDGE_CURVE('',#7886,#7888,#343,.T.);
#10563=EDGE_CURVE('',#7890,#7892,#132,.T.);
#10564=EDGE_CURVE('',#7897,#7894,#4836,.T.);
#10565=EDGE_CURVE('',#7936,#7934,#133,.T.);
#10566=EDGE_CURVE('',#7935,#7933,#134,.T.);
#10567=EDGE_CURVE('',#7937,#8241,#4837,.T.);
#10568=EDGE_CURVE('',#7893,#7898,#4838,.T.);
#10569=EDGE_CURVE('',#7885,#7887,#344,.F.);
#10570=EDGE_CURVE('',#8241,#7852,#135,.T.);
#10571=EDGE_CURVE('',#8241,#7851,#4839,.T.);
#10572=EDGE_CURVE('',#7890,#7891,#1433,.T.);
#10573=EDGE_CURVE('',#7852,#7851,#1434,.T.);
#10574=EDGE_CURVE('',#7891,#8242,#4840,.T.);
#10575=EDGE_CURVE('',#8242,#8242,#1435,.T.);
#10576=EDGE_CURVE('',#7851,#8243,#4841,.T.);
#10577=EDGE_CURVE('',#8243,#8243,#1436,.T.);
#10578=EDGE_CURVE('',#8240,#8244,#4842,.T.);
#10579=EDGE_CURVE('',#8244,#8244,#1437,.T.);
#10580=EDGE_CURVE('',#8245,#8245,#1438,.T.);
#10581=EDGE_CURVE('',#8245,#8246,#4843,.T.);
#10582=EDGE_CURVE('',#8246,#8246,#1439,.T.);
#10583=EDGE_CURVE('',#8238,#8245,#4844,.T.);
#13840=ORIENTED_EDGE('',*,*,#9972,.T.);
#13841=ORIENTED_EDGE('',*,*,#9973,.F.);
#13842=ORIENTED_EDGE('',*,*,#9974,.T.);
#13843=ORIENTED_EDGE('',*,*,#9975,.T.);
#13844=ORIENTED_EDGE('',*,*,#9976,.T.);
#13845=ORIENTED_EDGE('',*,*,#9977,.F.);
#13846=ORIENTED_EDGE('',*,*,#9972,.F.);
#13847=ORIENTED_EDGE('',*,*,#9978,.T.);
#13848=ORIENTED_EDGE('',*,*,#9979,.T.);
#13849=ORIENTED_EDGE('',*,*,#9980,.F.);
#13850=ORIENTED_EDGE('',*,*,#9976,.F.);
#13851=ORIENTED_EDGE('',*,*,#9981,.T.);
#13852=ORIENTED_EDGE('',*,*,#9982,.T.);
#13853=ORIENTED_EDGE('',*,*,#9983,.F.);
#13854=ORIENTED_EDGE('',*,*,#9979,.F.);
#13855=ORIENTED_EDGE('',*,*,#9984,.T.);
#13856=ORIENTED_EDGE('',*,*,#9985,.T.);
#13857=ORIENTED_EDGE('',*,*,#9986,.F.);
#13858=ORIENTED_EDGE('',*,*,#9982,.F.);
#13859=ORIENTED_EDGE('',*,*,#9987,.T.);
#13860=ORIENTED_EDGE('',*,*,#9988,.T.);
#13861=ORIENTED_EDGE('',*,*,#9989,.F.);
#13862=ORIENTED_EDGE('',*,*,#9985,.F.);
#13863=ORIENTED_EDGE('',*,*,#9990,.T.);
#13864=ORIENTED_EDGE('',*,*,#9991,.T.);
#13865=ORIENTED_EDGE('',*,*,#9992,.F.);
#13866=ORIENTED_EDGE('',*,*,#9988,.F.);
#13867=ORIENTED_EDGE('',*,*,#9993,.T.);
#13868=ORIENTED_EDGE('',*,*,#9994,.T.);
#13869=ORIENTED_EDGE('',*,*,#9995,.F.);
#13870=ORIENTED_EDGE('',*,*,#9991,.F.);
#13871=ORIENTED_EDGE('',*,*,#9996,.T.);
#13872=ORIENTED_EDGE('',*,*,#9997,.T.);
#13873=ORIENTED_EDGE('',*,*,#9998,.F.);
#13874=ORIENTED_EDGE('',*,*,#9994,.F.);
#13875=ORIENTED_EDGE('',*,*,#9999,.T.);
#13876=ORIENTED_EDGE('',*,*,#10000,.T.);
#13877=ORIENTED_EDGE('',*,*,#10001,.F.);
#13878=ORIENTED_EDGE('',*,*,#9997,.F.);
#13879=ORIENTED_EDGE('',*,*,#10002,.T.);
#13880=ORIENTED_EDGE('',*,*,#10003,.T.);
#13881=ORIENTED_EDGE('',*,*,#10004,.F.);
#13882=ORIENTED_EDGE('',*,*,#10000,.F.);
#13883=ORIENTED_EDGE('',*,*,#10005,.T.);
#13884=ORIENTED_EDGE('',*,*,#10006,.T.);
#13885=ORIENTED_EDGE('',*,*,#10007,.F.);
#13886=ORIENTED_EDGE('',*,*,#10003,.F.);
#13887=ORIENTED_EDGE('',*,*,#10008,.T.);
#13888=ORIENTED_EDGE('',*,*,#10009,.T.);
#13889=ORIENTED_EDGE('',*,*,#10010,.F.);
#13890=ORIENTED_EDGE('',*,*,#10006,.F.);
#13891=ORIENTED_EDGE('',*,*,#10011,.T.);
#13892=ORIENTED_EDGE('',*,*,#10012,.T.);
#13893=ORIENTED_EDGE('',*,*,#10013,.F.);
#13894=ORIENTED_EDGE('',*,*,#10009,.F.);
#13895=ORIENTED_EDGE('',*,*,#10014,.T.);
#13896=ORIENTED_EDGE('',*,*,#10015,.T.);
#13897=ORIENTED_EDGE('',*,*,#10016,.F.);
#13898=ORIENTED_EDGE('',*,*,#10012,.F.);
#13899=ORIENTED_EDGE('',*,*,#10017,.T.);
#13900=ORIENTED_EDGE('',*,*,#10018,.T.);
#13901=ORIENTED_EDGE('',*,*,#10019,.F.);
#13902=ORIENTED_EDGE('',*,*,#10015,.F.);
#13903=ORIENTED_EDGE('',*,*,#10020,.T.);
#13904=ORIENTED_EDGE('',*,*,#10021,.T.);
#13905=ORIENTED_EDGE('',*,*,#10022,.F.);
#13906=ORIENTED_EDGE('',*,*,#10018,.F.);
#13907=ORIENTED_EDGE('',*,*,#10023,.T.);
#13908=ORIENTED_EDGE('',*,*,#10024,.T.);
#13909=ORIENTED_EDGE('',*,*,#10025,.F.);
#13910=ORIENTED_EDGE('',*,*,#10021,.F.);
#13911=ORIENTED_EDGE('',*,*,#10026,.T.);
#13912=ORIENTED_EDGE('',*,*,#10027,.F.);
#13913=ORIENTED_EDGE('',*,*,#10028,.T.);
#13914=ORIENTED_EDGE('',*,*,#10029,.T.);
#13915=ORIENTED_EDGE('',*,*,#10030,.F.);
#13916=ORIENTED_EDGE('',*,*,#10031,.F.);
#13917=ORIENTED_EDGE('',*,*,#10032,.T.);
#13918=ORIENTED_EDGE('',*,*,#10033,.T.);
#13919=ORIENTED_EDGE('',*,*,#10034,.F.);
#13920=ORIENTED_EDGE('',*,*,#10035,.F.);
#13921=ORIENTED_EDGE('',*,*,#10036,.T.);
#13922=ORIENTED_EDGE('',*,*,#10037,.T.);
#13923=ORIENTED_EDGE('',*,*,#10038,.F.);
#13924=ORIENTED_EDGE('',*,*,#10039,.F.);
#13925=ORIENTED_EDGE('',*,*,#10040,.T.);
#13926=ORIENTED_EDGE('',*,*,#10041,.T.);
#13927=ORIENTED_EDGE('',*,*,#10036,.F.);
#13928=ORIENTED_EDGE('',*,*,#10042,.F.);
#13929=ORIENTED_EDGE('',*,*,#10043,.T.);
#13930=ORIENTED_EDGE('',*,*,#10044,.T.);
#13931=ORIENTED_EDGE('',*,*,#10040,.F.);
#13932=ORIENTED_EDGE('',*,*,#10045,.F.);
#13933=ORIENTED_EDGE('',*,*,#10046,.T.);
#13934=ORIENTED_EDGE('',*,*,#10047,.T.);
#13935=ORIENTED_EDGE('',*,*,#10043,.F.);
#13936=ORIENTED_EDGE('',*,*,#10048,.F.);
#13937=ORIENTED_EDGE('',*,*,#10049,.T.);
#13938=ORIENTED_EDGE('',*,*,#10050,.T.);
#13939=ORIENTED_EDGE('',*,*,#10046,.F.);
#13940=ORIENTED_EDGE('',*,*,#10051,.F.);
#13941=ORIENTED_EDGE('',*,*,#10052,.T.);
#13942=ORIENTED_EDGE('',*,*,#10053,.T.);
#13943=ORIENTED_EDGE('',*,*,#10049,.F.);
#13944=ORIENTED_EDGE('',*,*,#10054,.F.);
#13945=ORIENTED_EDGE('',*,*,#10055,.T.);
#13946=ORIENTED_EDGE('',*,*,#10056,.T.);
#13947=ORIENTED_EDGE('',*,*,#10052,.F.);
#13948=ORIENTED_EDGE('',*,*,#10057,.F.);
#13949=ORIENTED_EDGE('',*,*,#10058,.T.);
#13950=ORIENTED_EDGE('',*,*,#10059,.T.);
#13951=ORIENTED_EDGE('',*,*,#10055,.F.);
#13952=ORIENTED_EDGE('',*,*,#10060,.F.);
#13953=ORIENTED_EDGE('',*,*,#10061,.T.);
#13954=ORIENTED_EDGE('',*,*,#10062,.T.);
#13955=ORIENTED_EDGE('',*,*,#10058,.F.);
#13956=ORIENTED_EDGE('',*,*,#10063,.F.);
#13957=ORIENTED_EDGE('',*,*,#10064,.T.);
#13958=ORIENTED_EDGE('',*,*,#10065,.T.);
#13959=ORIENTED_EDGE('',*,*,#10061,.F.);
#13960=ORIENTED_EDGE('',*,*,#10066,.F.);
#13961=ORIENTED_EDGE('',*,*,#10067,.T.);
#13962=ORIENTED_EDGE('',*,*,#10068,.T.);
#13963=ORIENTED_EDGE('',*,*,#10064,.F.);
#13964=ORIENTED_EDGE('',*,*,#10069,.F.);
#13965=ORIENTED_EDGE('',*,*,#10070,.T.);
#13966=ORIENTED_EDGE('',*,*,#10071,.T.);
#13967=ORIENTED_EDGE('',*,*,#10067,.F.);
#13968=ORIENTED_EDGE('',*,*,#10072,.F.);
#13969=ORIENTED_EDGE('',*,*,#10073,.T.);
#13970=ORIENTED_EDGE('',*,*,#10074,.T.);
#13971=ORIENTED_EDGE('',*,*,#10070,.F.);
#13972=ORIENTED_EDGE('',*,*,#10075,.F.);
#13973=ORIENTED_EDGE('',*,*,#10076,.T.);
#13974=ORIENTED_EDGE('',*,*,#10077,.T.);
#13975=ORIENTED_EDGE('',*,*,#10073,.F.);
#13976=ORIENTED_EDGE('',*,*,#10078,.F.);
#13977=ORIENTED_EDGE('',*,*,#10079,.T.);
#13978=ORIENTED_EDGE('',*,*,#10080,.T.);
#13979=ORIENTED_EDGE('',*,*,#10076,.F.);
#13980=ORIENTED_EDGE('',*,*,#10081,.F.);
#13981=ORIENTED_EDGE('',*,*,#10082,.T.);
#13982=ORIENTED_EDGE('',*,*,#10083,.T.);
#13983=ORIENTED_EDGE('',*,*,#10079,.F.);
#13984=ORIENTED_EDGE('',*,*,#10084,.F.);
#13985=ORIENTED_EDGE('',*,*,#10085,.T.);
#13986=ORIENTED_EDGE('',*,*,#10086,.T.);
#13987=ORIENTED_EDGE('',*,*,#10082,.F.);
#13988=ORIENTED_EDGE('',*,*,#10087,.F.);
#13989=ORIENTED_EDGE('',*,*,#10088,.T.);
#13990=ORIENTED_EDGE('',*,*,#10089,.T.);
#13991=ORIENTED_EDGE('',*,*,#10085,.F.);
#13992=ORIENTED_EDGE('',*,*,#10090,.F.);
#13993=ORIENTED_EDGE('',*,*,#10091,.T.);
#13994=ORIENTED_EDGE('',*,*,#10092,.T.);
#13995=ORIENTED_EDGE('',*,*,#10088,.F.);
#13996=ORIENTED_EDGE('',*,*,#10093,.F.);
#13997=ORIENTED_EDGE('',*,*,#10094,.F.);
#13998=ORIENTED_EDGE('',*,*,#10095,.F.);
#13999=ORIENTED_EDGE('',*,*,#10096,.F.);
#14000=ORIENTED_EDGE('',*,*,#10097,.T.);
#14001=ORIENTED_EDGE('',*,*,#10098,.F.);
#14002=ORIENTED_EDGE('',*,*,#10099,.F.);
#14003=ORIENTED_EDGE('',*,*,#10100,.T.);
#14004=ORIENTED_EDGE('',*,*,#10101,.T.);
#14005=ORIENTED_EDGE('',*,*,#10102,.F.);
#14006=ORIENTED_EDGE('',*,*,#10103,.F.);
#14007=ORIENTED_EDGE('',*,*,#10098,.T.);
#14008=ORIENTED_EDGE('',*,*,#10104,.T.);
#14009=ORIENTED_EDGE('',*,*,#10105,.F.);
#14010=ORIENTED_EDGE('',*,*,#10106,.F.);
#14011=ORIENTED_EDGE('',*,*,#10102,.T.);
#14012=ORIENTED_EDGE('',*,*,#10107,.T.);
#14013=ORIENTED_EDGE('',*,*,#10108,.F.);
#14014=ORIENTED_EDGE('',*,*,#10109,.T.);
#14015=ORIENTED_EDGE('',*,*,#10110,.T.);
#14016=ORIENTED_EDGE('',*,*,#10111,.F.);
#14017=ORIENTED_EDGE('',*,*,#10112,.F.);
#14018=ORIENTED_EDGE('',*,*,#10113,.T.);
#14019=ORIENTED_EDGE('',*,*,#10108,.T.);
#14020=ORIENTED_EDGE('',*,*,#10114,.F.);
#14021=ORIENTED_EDGE('',*,*,#10115,.F.);
#14022=ORIENTED_EDGE('',*,*,#10116,.T.);
#14023=ORIENTED_EDGE('',*,*,#10112,.T.);
#14024=ORIENTED_EDGE('',*,*,#10117,.F.);
#14025=ORIENTED_EDGE('',*,*,#10118,.F.);
#14026=ORIENTED_EDGE('',*,*,#10119,.T.);
#14027=ORIENTED_EDGE('',*,*,#10115,.T.);
#14028=ORIENTED_EDGE('',*,*,#10120,.F.);
#14029=ORIENTED_EDGE('',*,*,#10121,.F.);
#14030=ORIENTED_EDGE('',*,*,#10122,.T.);
#14031=ORIENTED_EDGE('',*,*,#10118,.T.);
#14032=ORIENTED_EDGE('',*,*,#10123,.F.);
#14033=ORIENTED_EDGE('',*,*,#10124,.F.);
#14034=ORIENTED_EDGE('',*,*,#10125,.T.);
#14035=ORIENTED_EDGE('',*,*,#10121,.T.);
#14036=ORIENTED_EDGE('',*,*,#10126,.F.);
#14037=ORIENTED_EDGE('',*,*,#10127,.F.);
#14038=ORIENTED_EDGE('',*,*,#10128,.T.);
#14039=ORIENTED_EDGE('',*,*,#10124,.T.);
#14040=ORIENTED_EDGE('',*,*,#10129,.F.);
#14041=ORIENTED_EDGE('',*,*,#10130,.F.);
#14042=ORIENTED_EDGE('',*,*,#10131,.T.);
#14043=ORIENTED_EDGE('',*,*,#10127,.T.);
#14044=ORIENTED_EDGE('',*,*,#10132,.F.);
#14045=ORIENTED_EDGE('',*,*,#10133,.T.);
#14046=ORIENTED_EDGE('',*,*,#10134,.T.);
#14047=ORIENTED_EDGE('',*,*,#10135,.T.);
#14048=ORIENTED_EDGE('',*,*,#10136,.T.);
#14049=ORIENTED_EDGE('',*,*,#10137,.T.);
#14050=ORIENTED_EDGE('',*,*,#10138,.T.);
#14051=ORIENTED_EDGE('',*,*,#10133,.F.);
#14052=ORIENTED_EDGE('',*,*,#10139,.T.);
#14053=ORIENTED_EDGE('',*,*,#10140,.T.);
#14054=ORIENTED_EDGE('',*,*,#10141,.T.);
#14055=ORIENTED_EDGE('',*,*,#10137,.F.);
#14056=ORIENTED_EDGE('',*,*,#10142,.T.);
#14057=ORIENTED_EDGE('',*,*,#10143,.F.);
#14058=ORIENTED_EDGE('',*,*,#10144,.T.);
#14059=ORIENTED_EDGE('',*,*,#10145,.F.);
#14060=ORIENTED_EDGE('',*,*,#10146,.T.);
#14061=ORIENTED_EDGE('',*,*,#10143,.T.);
#14062=ORIENTED_EDGE('',*,*,#10147,.T.);
#14063=ORIENTED_EDGE('',*,*,#10140,.F.);
#14064=ORIENTED_EDGE('',*,*,#10148,.T.);
#14065=ORIENTED_EDGE('',*,*,#10149,.T.);
#14066=ORIENTED_EDGE('',*,*,#10150,.F.);
#14067=ORIENTED_EDGE('',*,*,#10151,.F.);
#14068=ORIENTED_EDGE('',*,*,#10152,.F.);
#14069=ORIENTED_EDGE('',*,*,#10153,.T.);
#14070=ORIENTED_EDGE('',*,*,#10154,.T.);
#14071=ORIENTED_EDGE('',*,*,#10151,.T.);
#14072=ORIENTED_EDGE('',*,*,#10155,.F.);
#14073=ORIENTED_EDGE('',*,*,#10156,.T.);
#14074=ORIENTED_EDGE('',*,*,#10155,.T.);
#14075=ORIENTED_EDGE('',*,*,#10150,.T.);
#14076=ORIENTED_EDGE('',*,*,#10157,.T.);
#14077=ORIENTED_EDGE('',*,*,#10158,.T.);
#14078=ORIENTED_EDGE('',*,*,#10159,.T.);
#14079=ORIENTED_EDGE('',*,*,#10160,.T.);
#14080=ORIENTED_EDGE('',*,*,#10161,.T.);
#14081=ORIENTED_EDGE('',*,*,#10152,.T.);
#14082=ORIENTED_EDGE('',*,*,#10154,.F.);
#14083=ORIENTED_EDGE('',*,*,#10162,.F.);
#14084=ORIENTED_EDGE('',*,*,#10163,.F.);
#14085=ORIENTED_EDGE('',*,*,#10164,.F.);
#14086=ORIENTED_EDGE('',*,*,#10165,.F.);
#14087=ORIENTED_EDGE('',*,*,#10166,.T.);
#14088=ORIENTED_EDGE('',*,*,#10167,.T.);
#14089=ORIENTED_EDGE('',*,*,#10168,.T.);
#14090=ORIENTED_EDGE('',*,*,#10164,.T.);
#14091=ORIENTED_EDGE('',*,*,#10169,.F.);
#14092=ORIENTED_EDGE('',*,*,#10170,.T.);
#14093=ORIENTED_EDGE('',*,*,#10169,.T.);
#14094=ORIENTED_EDGE('',*,*,#10163,.T.);
#14095=ORIENTED_EDGE('',*,*,#10171,.F.);
#14096=ORIENTED_EDGE('',*,*,#10172,.T.);
#14097=ORIENTED_EDGE('',*,*,#10171,.T.);
#14098=ORIENTED_EDGE('',*,*,#10162,.T.);
#14099=ORIENTED_EDGE('',*,*,#10173,.T.);
#14100=ORIENTED_EDGE('',*,*,#10174,.T.);
#14101=ORIENTED_EDGE('',*,*,#10175,.F.);
#14102=ORIENTED_EDGE('',*,*,#10176,.F.);
#14103=ORIENTED_EDGE('',*,*,#10177,.F.);
#14104=ORIENTED_EDGE('',*,*,#10178,.F.);
#14105=ORIENTED_EDGE('',*,*,#10179,.T.);
#14106=ORIENTED_EDGE('',*,*,#10180,.T.);
#14107=ORIENTED_EDGE('',*,*,#10181,.T.);
#14108=ORIENTED_EDGE('',*,*,#10177,.T.);
#14109=ORIENTED_EDGE('',*,*,#10182,.F.);
#14110=ORIENTED_EDGE('',*,*,#10183,.T.);
#14111=ORIENTED_EDGE('',*,*,#10182,.T.);
#14112=ORIENTED_EDGE('',*,*,#10176,.T.);
#14113=ORIENTED_EDGE('',*,*,#10184,.F.);
#14114=ORIENTED_EDGE('',*,*,#10185,.T.);
#14115=ORIENTED_EDGE('',*,*,#10184,.T.);
#14116=ORIENTED_EDGE('',*,*,#10175,.T.);
#14117=ORIENTED_EDGE('',*,*,#10186,.T.);
#14118=ORIENTED_EDGE('',*,*,#10187,.T.);
#14119=ORIENTED_EDGE('',*,*,#10188,.F.);
#14120=ORIENTED_EDGE('',*,*,#10189,.F.);
#14121=ORIENTED_EDGE('',*,*,#10190,.F.);
#14122=ORIENTED_EDGE('',*,*,#10191,.F.);
#14123=ORIENTED_EDGE('',*,*,#10192,.F.);
#14124=ORIENTED_EDGE('',*,*,#10193,.T.);
#14125=ORIENTED_EDGE('',*,*,#10194,.T.);
#14126=ORIENTED_EDGE('',*,*,#10195,.T.);
#14127=ORIENTED_EDGE('',*,*,#10190,.T.);
#14128=ORIENTED_EDGE('',*,*,#10196,.F.);
#14129=ORIENTED_EDGE('',*,*,#10197,.T.);
#14130=ORIENTED_EDGE('',*,*,#10198,.T.);
#14131=ORIENTED_EDGE('',*,*,#10196,.T.);
#14132=ORIENTED_EDGE('',*,*,#10189,.T.);
#14133=ORIENTED_EDGE('',*,*,#10199,.F.);
#14134=ORIENTED_EDGE('',*,*,#10200,.T.);
#14135=ORIENTED_EDGE('',*,*,#10199,.T.);
#14136=ORIENTED_EDGE('',*,*,#10188,.T.);
#14137=ORIENTED_EDGE('',*,*,#10201,.T.);
#14138=ORIENTED_EDGE('',*,*,#10202,.T.);
#14139=ORIENTED_EDGE('',*,*,#10158,.F.);
#14140=ORIENTED_EDGE('',*,*,#10203,.F.);
#14141=ORIENTED_EDGE('',*,*,#10167,.F.);
#14142=ORIENTED_EDGE('',*,*,#10204,.T.);
#14143=ORIENTED_EDGE('',*,*,#10157,.F.);
#14144=ORIENTED_EDGE('',*,*,#10205,.F.);
#14145=ORIENTED_EDGE('',*,*,#10168,.F.);
#14146=ORIENTED_EDGE('',*,*,#10203,.T.);
#14147=ORIENTED_EDGE('',*,*,#10206,.F.);
#14148=ORIENTED_EDGE('',*,*,#10207,.T.);
#14149=ORIENTED_EDGE('',*,*,#10191,.T.);
#14150=ORIENTED_EDGE('',*,*,#10208,.T.);
#14151=ORIENTED_EDGE('',*,*,#10178,.T.);
#14152=ORIENTED_EDGE('',*,*,#10209,.T.);
#14153=ORIENTED_EDGE('',*,*,#10165,.T.);
#14154=ORIENTED_EDGE('',*,*,#10205,.T.);
#14155=ORIENTED_EDGE('',*,*,#10149,.F.);
#14156=ORIENTED_EDGE('',*,*,#10210,.T.);
#14157=ORIENTED_EDGE('',*,*,#10192,.T.);
#14158=ORIENTED_EDGE('',*,*,#10207,.F.);
#14159=ORIENTED_EDGE('',*,*,#10206,.T.);
#14160=ORIENTED_EDGE('',*,*,#10211,.F.);
#14161=ORIENTED_EDGE('',*,*,#10100,.F.);
#14162=ORIENTED_EDGE('',*,*,#10212,.F.);
#14163=ORIENTED_EDGE('',*,*,#10135,.F.);
#14164=ORIENTED_EDGE('',*,*,#10213,.F.);
#14165=ORIENTED_EDGE('',*,*,#10214,.T.);
#14166=ORIENTED_EDGE('',*,*,#10215,.T.);
#14167=ORIENTED_EDGE('',*,*,#10214,.F.);
#14168=ORIENTED_EDGE('',*,*,#10216,.F.);
#14169=ORIENTED_EDGE('',*,*,#10217,.T.);
#14170=ORIENTED_EDGE('',*,*,#10213,.T.);
#14171=ORIENTED_EDGE('',*,*,#10217,.F.);
#14172=ORIENTED_EDGE('',*,*,#10170,.F.);
#14173=ORIENTED_EDGE('',*,*,#10172,.F.);
#14174=ORIENTED_EDGE('',*,*,#10218,.F.);
#14175=ORIENTED_EDGE('',*,*,#10179,.F.);
#14176=ORIENTED_EDGE('',*,*,#10183,.F.);
#14177=ORIENTED_EDGE('',*,*,#10185,.F.);
#14178=ORIENTED_EDGE('',*,*,#10219,.F.);
#14179=ORIENTED_EDGE('',*,*,#10193,.F.);
#14180=ORIENTED_EDGE('',*,*,#10198,.F.);
#14181=ORIENTED_EDGE('',*,*,#10220,.T.);
#14182=ORIENTED_EDGE('',*,*,#10216,.T.);
#14183=ORIENTED_EDGE('',*,*,#10220,.F.);
#14184=ORIENTED_EDGE('',*,*,#10197,.F.);
#14185=ORIENTED_EDGE('',*,*,#10200,.F.);
#14186=ORIENTED_EDGE('',*,*,#10221,.F.);
#14187=ORIENTED_EDGE('',*,*,#10159,.F.);
#14188=ORIENTED_EDGE('',*,*,#10153,.F.);
#14189=ORIENTED_EDGE('',*,*,#10156,.F.);
#14190=ORIENTED_EDGE('',*,*,#10204,.F.);
#14191=ORIENTED_EDGE('',*,*,#10166,.F.);
#14192=ORIENTED_EDGE('',*,*,#10187,.F.);
#14193=ORIENTED_EDGE('',*,*,#10222,.F.);
#14194=ORIENTED_EDGE('',*,*,#10194,.F.);
#14195=ORIENTED_EDGE('',*,*,#10219,.T.);
#14196=ORIENTED_EDGE('',*,*,#10174,.F.);
#14197=ORIENTED_EDGE('',*,*,#10223,.F.);
#14198=ORIENTED_EDGE('',*,*,#10180,.F.);
#14199=ORIENTED_EDGE('',*,*,#10218,.T.);
#14200=ORIENTED_EDGE('',*,*,#10160,.F.);
#14201=ORIENTED_EDGE('',*,*,#10221,.T.);
#14202=ORIENTED_EDGE('',*,*,#10202,.F.);
#14203=ORIENTED_EDGE('',*,*,#10224,.F.);
#14204=ORIENTED_EDGE('',*,*,#10186,.F.);
#14205=ORIENTED_EDGE('',*,*,#10208,.F.);
#14206=ORIENTED_EDGE('',*,*,#10195,.F.);
#14207=ORIENTED_EDGE('',*,*,#10222,.T.);
#14208=ORIENTED_EDGE('',*,*,#10173,.F.);
#14209=ORIENTED_EDGE('',*,*,#10209,.F.);
#14210=ORIENTED_EDGE('',*,*,#10181,.F.);
#14211=ORIENTED_EDGE('',*,*,#10223,.T.);
#14212=ORIENTED_EDGE('',*,*,#10161,.F.);
#14213=ORIENTED_EDGE('',*,*,#10224,.T.);
#14214=ORIENTED_EDGE('',*,*,#10201,.F.);
#14215=ORIENTED_EDGE('',*,*,#10210,.F.);
#14216=ORIENTED_EDGE('',*,*,#10146,.F.);
#14217=ORIENTED_EDGE('',*,*,#10225,.T.);
#14218=ORIENTED_EDGE('',*,*,#10226,.T.);
#14219=ORIENTED_EDGE('',*,*,#10132,.T.);
#14220=ORIENTED_EDGE('',*,*,#10129,.T.);
#14221=ORIENTED_EDGE('',*,*,#10126,.T.);
#14222=ORIENTED_EDGE('',*,*,#10123,.T.);
#14223=ORIENTED_EDGE('',*,*,#10120,.T.);
#14224=ORIENTED_EDGE('',*,*,#10117,.T.);
#14225=ORIENTED_EDGE('',*,*,#10114,.T.);
#14226=ORIENTED_EDGE('',*,*,#10111,.T.);
#14227=ORIENTED_EDGE('',*,*,#10227,.T.);
#14228=ORIENTED_EDGE('',*,*,#10228,.F.);
#14229=ORIENTED_EDGE('',*,*,#10229,.F.);
#14230=ORIENTED_EDGE('',*,*,#10107,.F.);
#14231=ORIENTED_EDGE('',*,*,#10104,.F.);
#14232=ORIENTED_EDGE('',*,*,#10101,.F.);
#14233=ORIENTED_EDGE('',*,*,#10211,.T.);
#14234=ORIENTED_EDGE('',*,*,#10134,.F.);
#14235=ORIENTED_EDGE('',*,*,#10138,.F.);
#14236=ORIENTED_EDGE('',*,*,#10141,.F.);
#14237=ORIENTED_EDGE('',*,*,#10147,.F.);
#14238=ORIENTED_EDGE('',*,*,#10136,.F.);
#14239=ORIENTED_EDGE('',*,*,#10212,.T.);
#14240=ORIENTED_EDGE('',*,*,#10099,.T.);
#14241=ORIENTED_EDGE('',*,*,#10103,.T.);
#14242=ORIENTED_EDGE('',*,*,#10106,.T.);
#14243=ORIENTED_EDGE('',*,*,#10230,.T.);
#14244=ORIENTED_EDGE('',*,*,#10231,.T.);
#14245=ORIENTED_EDGE('',*,*,#10109,.F.);
#14246=ORIENTED_EDGE('',*,*,#10113,.F.);
#14247=ORIENTED_EDGE('',*,*,#10116,.F.);
#14248=ORIENTED_EDGE('',*,*,#10119,.F.);
#14249=ORIENTED_EDGE('',*,*,#10122,.F.);
#14250=ORIENTED_EDGE('',*,*,#10125,.F.);
#14251=ORIENTED_EDGE('',*,*,#10128,.F.);
#14252=ORIENTED_EDGE('',*,*,#10131,.F.);
#14253=ORIENTED_EDGE('',*,*,#10232,.F.);
#14254=ORIENTED_EDGE('',*,*,#10233,.T.);
#14255=ORIENTED_EDGE('',*,*,#10144,.F.);
#14256=ORIENTED_EDGE('',*,*,#10148,.F.);
#14257=ORIENTED_EDGE('',*,*,#10142,.F.);
#14258=ORIENTED_EDGE('',*,*,#10139,.F.);
#14259=ORIENTED_EDGE('',*,*,#10225,.F.);
#14260=ORIENTED_EDGE('',*,*,#10145,.T.);
#14261=ORIENTED_EDGE('',*,*,#10233,.F.);
#14262=ORIENTED_EDGE('',*,*,#10234,.F.);
#14263=ORIENTED_EDGE('',*,*,#10215,.F.);
#14264=ORIENTED_EDGE('',*,*,#10235,.T.);
#14265=ORIENTED_EDGE('',*,*,#10236,.F.);
#14266=ORIENTED_EDGE('',*,*,#10237,.T.);
#14267=ORIENTED_EDGE('',*,*,#10238,.T.);
#14268=ORIENTED_EDGE('',*,*,#10237,.F.);
#14269=ORIENTED_EDGE('',*,*,#10228,.T.);
#14270=ORIENTED_EDGE('',*,*,#10239,.T.);
#14271=ORIENTED_EDGE('',*,*,#10240,.T.);
#14272=ORIENTED_EDGE('',*,*,#10130,.T.);
#14273=ORIENTED_EDGE('',*,*,#10226,.F.);
#14274=ORIENTED_EDGE('',*,*,#10234,.T.);
#14275=ORIENTED_EDGE('',*,*,#10232,.T.);
#14276=ORIENTED_EDGE('',*,*,#10231,.F.);
#14277=ORIENTED_EDGE('',*,*,#10239,.F.);
#14278=ORIENTED_EDGE('',*,*,#10227,.F.);
#14279=ORIENTED_EDGE('',*,*,#10110,.F.);
#14280=ORIENTED_EDGE('',*,*,#10238,.F.);
#14281=ORIENTED_EDGE('',*,*,#10241,.T.);
#14282=ORIENTED_EDGE('',*,*,#10235,.F.);
#14283=ORIENTED_EDGE('',*,*,#10241,.F.);
#14284=ORIENTED_EDGE('',*,*,#10242,.F.);
#14285=ORIENTED_EDGE('',*,*,#10243,.T.);
#14286=ORIENTED_EDGE('',*,*,#10244,.F.);
#14287=ORIENTED_EDGE('',*,*,#10245,.F.);
#14288=ORIENTED_EDGE('',*,*,#10243,.F.);
#14289=ORIENTED_EDGE('',*,*,#10246,.T.);
#14290=ORIENTED_EDGE('',*,*,#10247,.T.);
#14291=ORIENTED_EDGE('',*,*,#10248,.F.);
#14292=ORIENTED_EDGE('',*,*,#10247,.F.);
#14293=ORIENTED_EDGE('',*,*,#10249,.T.);
#14294=ORIENTED_EDGE('',*,*,#10250,.T.);
#14295=ORIENTED_EDGE('',*,*,#10251,.F.);
#14296=ORIENTED_EDGE('',*,*,#10250,.F.);
#14297=ORIENTED_EDGE('',*,*,#10251,.T.);
#14298=ORIENTED_EDGE('',*,*,#10246,.F.);
#14299=ORIENTED_EDGE('',*,*,#10252,.F.);
#14300=ORIENTED_EDGE('',*,*,#10248,.T.);
#14301=ORIENTED_EDGE('',*,*,#10253,.T.);
#14302=ORIENTED_EDGE('',*,*,#10254,.T.);
#14303=ORIENTED_EDGE('',*,*,#10255,.T.);
#14304=ORIENTED_EDGE('',*,*,#10256,.T.);
#14305=ORIENTED_EDGE('',*,*,#10257,.T.);
#14306=ORIENTED_EDGE('',*,*,#10258,.T.);
#14307=ORIENTED_EDGE('',*,*,#10244,.T.);
#14308=ORIENTED_EDGE('',*,*,#10245,.T.);
#14309=ORIENTED_EDGE('',*,*,#10258,.F.);
#14310=ORIENTED_EDGE('',*,*,#10259,.T.);
#14311=ORIENTED_EDGE('',*,*,#10260,.T.);
#14312=ORIENTED_EDGE('',*,*,#10261,.T.);
#14313=ORIENTED_EDGE('',*,*,#10262,.T.);
#14314=ORIENTED_EDGE('',*,*,#10242,.T.);
#14315=ORIENTED_EDGE('',*,*,#10263,.F.);
#14316=ORIENTED_EDGE('',*,*,#10240,.F.);
#14317=ORIENTED_EDGE('',*,*,#10264,.T.);
#14318=ORIENTED_EDGE('',*,*,#10265,.T.);
#14319=ORIENTED_EDGE('',*,*,#10259,.F.);
#14320=ORIENTED_EDGE('',*,*,#10257,.F.);
#14321=ORIENTED_EDGE('',*,*,#10266,.T.);
#14322=ORIENTED_EDGE('',*,*,#10255,.F.);
#14323=ORIENTED_EDGE('',*,*,#10267,.T.);
#14324=ORIENTED_EDGE('',*,*,#10253,.F.);
#14325=ORIENTED_EDGE('',*,*,#10268,.T.);
#14326=ORIENTED_EDGE('',*,*,#10261,.F.);
#14327=ORIENTED_EDGE('',*,*,#10269,.T.);
#14328=ORIENTED_EDGE('',*,*,#10270,.T.);
#14329=ORIENTED_EDGE('',*,*,#10264,.F.);
#14330=ORIENTED_EDGE('',*,*,#10271,.F.);
#14331=ORIENTED_EDGE('',*,*,#10265,.F.);
#14332=ORIENTED_EDGE('',*,*,#10270,.F.);
#14333=ORIENTED_EDGE('',*,*,#10272,.T.);
#14334=ORIENTED_EDGE('',*,*,#10273,.T.);
#14335=ORIENTED_EDGE('',*,*,#10274,.F.);
#14336=ORIENTED_EDGE('',*,*,#10266,.F.);
#14337=ORIENTED_EDGE('',*,*,#10275,.F.);
#14338=ORIENTED_EDGE('',*,*,#10273,.F.);
#14339=ORIENTED_EDGE('',*,*,#10276,.T.);
#14340=ORIENTED_EDGE('',*,*,#10277,.T.);
#14341=ORIENTED_EDGE('',*,*,#10278,.F.);
#14342=ORIENTED_EDGE('',*,*,#10267,.F.);
#14343=ORIENTED_EDGE('',*,*,#10279,.F.);
#14344=ORIENTED_EDGE('',*,*,#10277,.F.);
#14345=ORIENTED_EDGE('',*,*,#10280,.T.);
#14346=ORIENTED_EDGE('',*,*,#10281,.T.);
#14347=ORIENTED_EDGE('',*,*,#10282,.F.);
#14348=ORIENTED_EDGE('',*,*,#10268,.F.);
#14349=ORIENTED_EDGE('',*,*,#10283,.F.);
#14350=ORIENTED_EDGE('',*,*,#10281,.F.);
#14351=ORIENTED_EDGE('',*,*,#10252,.T.);
#14352=ORIENTED_EDGE('',*,*,#10284,.T.);
#14353=ORIENTED_EDGE('',*,*,#10285,.T.);
#14354=ORIENTED_EDGE('',*,*,#10284,.F.);
#14355=ORIENTED_EDGE('',*,*,#10286,.T.);
#14356=ORIENTED_EDGE('',*,*,#10287,.F.);
#14357=ORIENTED_EDGE('',*,*,#10288,.F.);
#14358=ORIENTED_EDGE('',*,*,#10289,.T.);
#14359=ORIENTED_EDGE('',*,*,#10290,.T.);
#14360=ORIENTED_EDGE('',*,*,#10289,.F.);
#14361=ORIENTED_EDGE('',*,*,#10291,.F.);
#14362=ORIENTED_EDGE('',*,*,#10292,.T.);
#14363=ORIENTED_EDGE('',*,*,#10293,.T.);
#14364=ORIENTED_EDGE('',*,*,#10292,.F.);
#14365=ORIENTED_EDGE('',*,*,#10294,.F.);
#14366=ORIENTED_EDGE('',*,*,#10295,.T.);
#14367=ORIENTED_EDGE('',*,*,#10296,.T.);
#14368=ORIENTED_EDGE('',*,*,#10295,.F.);
#14369=ORIENTED_EDGE('',*,*,#10297,.F.);
#14370=ORIENTED_EDGE('',*,*,#10298,.T.);
#14371=ORIENTED_EDGE('',*,*,#10299,.T.);
#14372=ORIENTED_EDGE('',*,*,#10298,.F.);
#14373=ORIENTED_EDGE('',*,*,#10300,.F.);
#14374=ORIENTED_EDGE('',*,*,#10301,.T.);
#14375=ORIENTED_EDGE('',*,*,#10302,.T.);
#14376=ORIENTED_EDGE('',*,*,#10301,.F.);
#14377=ORIENTED_EDGE('',*,*,#10303,.F.);
#14378=ORIENTED_EDGE('',*,*,#10304,.T.);
#14379=ORIENTED_EDGE('',*,*,#10305,.T.);
#14380=ORIENTED_EDGE('',*,*,#10304,.F.);
#14381=ORIENTED_EDGE('',*,*,#10306,.F.);
#14382=ORIENTED_EDGE('',*,*,#10307,.T.);
#14383=ORIENTED_EDGE('',*,*,#10308,.T.);
#14384=ORIENTED_EDGE('',*,*,#10307,.F.);
#14385=ORIENTED_EDGE('',*,*,#10309,.F.);
#14386=ORIENTED_EDGE('',*,*,#10310,.T.);
#14387=ORIENTED_EDGE('',*,*,#10311,.T.);
#14388=ORIENTED_EDGE('',*,*,#10310,.F.);
#14389=ORIENTED_EDGE('',*,*,#10312,.F.);
#14390=ORIENTED_EDGE('',*,*,#10313,.T.);
#14391=ORIENTED_EDGE('',*,*,#10314,.T.);
#14392=ORIENTED_EDGE('',*,*,#10313,.F.);
#14393=ORIENTED_EDGE('',*,*,#10315,.F.);
#14394=ORIENTED_EDGE('',*,*,#10316,.T.);
#14395=ORIENTED_EDGE('',*,*,#10317,.T.);
#14396=ORIENTED_EDGE('',*,*,#10316,.F.);
#14397=ORIENTED_EDGE('',*,*,#10318,.F.);
#14398=ORIENTED_EDGE('',*,*,#10319,.T.);
#14399=ORIENTED_EDGE('',*,*,#10320,.T.);
#14400=ORIENTED_EDGE('',*,*,#10319,.F.);
#14401=ORIENTED_EDGE('',*,*,#10321,.F.);
#14402=ORIENTED_EDGE('',*,*,#10322,.T.);
#14403=ORIENTED_EDGE('',*,*,#10323,.T.);
#14404=ORIENTED_EDGE('',*,*,#10322,.F.);
#14405=ORIENTED_EDGE('',*,*,#10324,.F.);
#14406=ORIENTED_EDGE('',*,*,#10325,.T.);
#14407=ORIENTED_EDGE('',*,*,#10326,.T.);
#14408=ORIENTED_EDGE('',*,*,#10325,.F.);
#14409=ORIENTED_EDGE('',*,*,#10327,.F.);
#14410=ORIENTED_EDGE('',*,*,#10328,.T.);
#14411=ORIENTED_EDGE('',*,*,#10329,.T.);
#14412=ORIENTED_EDGE('',*,*,#10328,.F.);
#14413=ORIENTED_EDGE('',*,*,#10330,.F.);
#14414=ORIENTED_EDGE('',*,*,#10331,.T.);
#14415=ORIENTED_EDGE('',*,*,#10332,.T.);
#14416=ORIENTED_EDGE('',*,*,#10331,.F.);
#14417=ORIENTED_EDGE('',*,*,#10333,.F.);
#14418=ORIENTED_EDGE('',*,*,#10334,.T.);
#14419=ORIENTED_EDGE('',*,*,#10335,.T.);
#14420=ORIENTED_EDGE('',*,*,#10334,.F.);
#14421=ORIENTED_EDGE('',*,*,#10336,.F.);
#14422=ORIENTED_EDGE('',*,*,#10337,.T.);
#14423=ORIENTED_EDGE('',*,*,#10338,.T.);
#14424=ORIENTED_EDGE('',*,*,#10337,.F.);
#14425=ORIENTED_EDGE('',*,*,#10339,.F.);
#14426=ORIENTED_EDGE('',*,*,#10340,.T.);
#14427=ORIENTED_EDGE('',*,*,#10341,.T.);
#14428=ORIENTED_EDGE('',*,*,#10340,.F.);
#14429=ORIENTED_EDGE('',*,*,#10342,.F.);
#14430=ORIENTED_EDGE('',*,*,#10343,.T.);
#14431=ORIENTED_EDGE('',*,*,#10344,.T.);
#14432=ORIENTED_EDGE('',*,*,#10343,.F.);
#14433=ORIENTED_EDGE('',*,*,#10345,.F.);
#14434=ORIENTED_EDGE('',*,*,#10346,.T.);
#14435=ORIENTED_EDGE('',*,*,#10347,.T.);
#14436=ORIENTED_EDGE('',*,*,#10346,.F.);
#14437=ORIENTED_EDGE('',*,*,#10348,.F.);
#14438=ORIENTED_EDGE('',*,*,#10349,.T.);
#14439=ORIENTED_EDGE('',*,*,#10350,.T.);
#14440=ORIENTED_EDGE('',*,*,#10349,.F.);
#14441=ORIENTED_EDGE('',*,*,#10351,.F.);
#14442=ORIENTED_EDGE('',*,*,#10352,.T.);
#14443=ORIENTED_EDGE('',*,*,#10353,.T.);
#14444=ORIENTED_EDGE('',*,*,#10352,.F.);
#14445=ORIENTED_EDGE('',*,*,#10354,.F.);
#14446=ORIENTED_EDGE('',*,*,#10355,.T.);
#14447=ORIENTED_EDGE('',*,*,#10356,.T.);
#14448=ORIENTED_EDGE('',*,*,#10355,.F.);
#14449=ORIENTED_EDGE('',*,*,#10357,.F.);
#14450=ORIENTED_EDGE('',*,*,#10358,.T.);
#14451=ORIENTED_EDGE('',*,*,#10359,.T.);
#14452=ORIENTED_EDGE('',*,*,#10358,.F.);
#14453=ORIENTED_EDGE('',*,*,#10360,.F.);
#14454=ORIENTED_EDGE('',*,*,#10361,.T.);
#14455=ORIENTED_EDGE('',*,*,#10362,.T.);
#14456=ORIENTED_EDGE('',*,*,#10361,.F.);
#14457=ORIENTED_EDGE('',*,*,#10363,.F.);
#14458=ORIENTED_EDGE('',*,*,#10364,.T.);
#14459=ORIENTED_EDGE('',*,*,#10365,.T.);
#14460=ORIENTED_EDGE('',*,*,#10364,.F.);
#14461=ORIENTED_EDGE('',*,*,#10366,.F.);
#14462=ORIENTED_EDGE('',*,*,#10367,.T.);
#14463=ORIENTED_EDGE('',*,*,#10368,.T.);
#14464=ORIENTED_EDGE('',*,*,#10367,.F.);
#14465=ORIENTED_EDGE('',*,*,#10369,.F.);
#14466=ORIENTED_EDGE('',*,*,#10370,.T.);
#14467=ORIENTED_EDGE('',*,*,#10371,.T.);
#14468=ORIENTED_EDGE('',*,*,#10370,.F.);
#14469=ORIENTED_EDGE('',*,*,#10372,.F.);
#14470=ORIENTED_EDGE('',*,*,#10373,.T.);
#14471=ORIENTED_EDGE('',*,*,#10374,.T.);
#14472=ORIENTED_EDGE('',*,*,#10373,.F.);
#14473=ORIENTED_EDGE('',*,*,#10375,.F.);
#14474=ORIENTED_EDGE('',*,*,#10376,.T.);
#14475=ORIENTED_EDGE('',*,*,#10377,.T.);
#14476=ORIENTED_EDGE('',*,*,#10376,.F.);
#14477=ORIENTED_EDGE('',*,*,#10378,.F.);
#14478=ORIENTED_EDGE('',*,*,#10379,.T.);
#14479=ORIENTED_EDGE('',*,*,#10380,.T.);
#14480=ORIENTED_EDGE('',*,*,#10379,.F.);
#14481=ORIENTED_EDGE('',*,*,#10381,.F.);
#14482=ORIENTED_EDGE('',*,*,#10382,.T.);
#14483=ORIENTED_EDGE('',*,*,#10383,.T.);
#14484=ORIENTED_EDGE('',*,*,#10382,.F.);
#14485=ORIENTED_EDGE('',*,*,#10384,.F.);
#14486=ORIENTED_EDGE('',*,*,#10385,.T.);
#14487=ORIENTED_EDGE('',*,*,#10386,.T.);
#14488=ORIENTED_EDGE('',*,*,#10385,.F.);
#14489=ORIENTED_EDGE('',*,*,#10387,.F.);
#14490=ORIENTED_EDGE('',*,*,#10388,.T.);
#14491=ORIENTED_EDGE('',*,*,#10389,.T.);
#14492=ORIENTED_EDGE('',*,*,#10388,.F.);
#14493=ORIENTED_EDGE('',*,*,#10390,.F.);
#14494=ORIENTED_EDGE('',*,*,#10391,.T.);
#14495=ORIENTED_EDGE('',*,*,#10392,.T.);
#14496=ORIENTED_EDGE('',*,*,#10391,.F.);
#14497=ORIENTED_EDGE('',*,*,#10393,.F.);
#14498=ORIENTED_EDGE('',*,*,#10394,.T.);
#14499=ORIENTED_EDGE('',*,*,#10395,.T.);
#14500=ORIENTED_EDGE('',*,*,#10394,.F.);
#14501=ORIENTED_EDGE('',*,*,#10396,.F.);
#14502=ORIENTED_EDGE('',*,*,#10397,.T.);
#14503=ORIENTED_EDGE('',*,*,#10398,.T.);
#14504=ORIENTED_EDGE('',*,*,#10397,.F.);
#14505=ORIENTED_EDGE('',*,*,#10399,.F.);
#14506=ORIENTED_EDGE('',*,*,#10400,.T.);
#14507=ORIENTED_EDGE('',*,*,#10401,.T.);
#14508=ORIENTED_EDGE('',*,*,#10400,.F.);
#14509=ORIENTED_EDGE('',*,*,#10402,.F.);
#14510=ORIENTED_EDGE('',*,*,#10403,.T.);
#14511=ORIENTED_EDGE('',*,*,#10404,.T.);
#14512=ORIENTED_EDGE('',*,*,#10403,.F.);
#14513=ORIENTED_EDGE('',*,*,#10405,.F.);
#14514=ORIENTED_EDGE('',*,*,#10406,.T.);
#14515=ORIENTED_EDGE('',*,*,#10407,.T.);
#14516=ORIENTED_EDGE('',*,*,#10406,.F.);
#14517=ORIENTED_EDGE('',*,*,#10408,.F.);
#14518=ORIENTED_EDGE('',*,*,#10409,.T.);
#14519=ORIENTED_EDGE('',*,*,#10410,.T.);
#14520=ORIENTED_EDGE('',*,*,#10409,.F.);
#14521=ORIENTED_EDGE('',*,*,#10411,.F.);
#14522=ORIENTED_EDGE('',*,*,#10412,.T.);
#14523=ORIENTED_EDGE('',*,*,#10413,.T.);
#14524=ORIENTED_EDGE('',*,*,#10412,.F.);
#14525=ORIENTED_EDGE('',*,*,#10414,.F.);
#14526=ORIENTED_EDGE('',*,*,#10415,.T.);
#14527=ORIENTED_EDGE('',*,*,#10416,.T.);
#14528=ORIENTED_EDGE('',*,*,#10415,.F.);
#14529=ORIENTED_EDGE('',*,*,#10417,.F.);
#14530=ORIENTED_EDGE('',*,*,#10418,.T.);
#14531=ORIENTED_EDGE('',*,*,#10419,.T.);
#14532=ORIENTED_EDGE('',*,*,#10418,.F.);
#14533=ORIENTED_EDGE('',*,*,#10420,.F.);
#14534=ORIENTED_EDGE('',*,*,#10421,.T.);
#14535=ORIENTED_EDGE('',*,*,#10422,.T.);
#14536=ORIENTED_EDGE('',*,*,#10421,.F.);
#14537=ORIENTED_EDGE('',*,*,#10423,.F.);
#14538=ORIENTED_EDGE('',*,*,#10424,.T.);
#14539=ORIENTED_EDGE('',*,*,#10425,.T.);
#14540=ORIENTED_EDGE('',*,*,#10424,.F.);
#14541=ORIENTED_EDGE('',*,*,#10426,.F.);
#14542=ORIENTED_EDGE('',*,*,#10427,.T.);
#14543=ORIENTED_EDGE('',*,*,#10428,.T.);
#14544=ORIENTED_EDGE('',*,*,#10427,.F.);
#14545=ORIENTED_EDGE('',*,*,#10429,.F.);
#14546=ORIENTED_EDGE('',*,*,#10430,.T.);
#14547=ORIENTED_EDGE('',*,*,#10431,.T.);
#14548=ORIENTED_EDGE('',*,*,#10430,.F.);
#14549=ORIENTED_EDGE('',*,*,#10432,.F.);
#14550=ORIENTED_EDGE('',*,*,#10433,.T.);
#14551=ORIENTED_EDGE('',*,*,#10434,.T.);
#14552=ORIENTED_EDGE('',*,*,#10433,.F.);
#14553=ORIENTED_EDGE('',*,*,#10435,.F.);
#14554=ORIENTED_EDGE('',*,*,#10436,.T.);
#14555=ORIENTED_EDGE('',*,*,#10437,.T.);
#14556=ORIENTED_EDGE('',*,*,#10436,.F.);
#14557=ORIENTED_EDGE('',*,*,#10438,.F.);
#14558=ORIENTED_EDGE('',*,*,#10439,.T.);
#14559=ORIENTED_EDGE('',*,*,#10440,.T.);
#14560=ORIENTED_EDGE('',*,*,#10439,.F.);
#14561=ORIENTED_EDGE('',*,*,#10441,.F.);
#14562=ORIENTED_EDGE('',*,*,#10442,.T.);
#14563=ORIENTED_EDGE('',*,*,#10443,.T.);
#14564=ORIENTED_EDGE('',*,*,#10442,.F.);
#14565=ORIENTED_EDGE('',*,*,#10444,.F.);
#14566=ORIENTED_EDGE('',*,*,#10445,.T.);
#14567=ORIENTED_EDGE('',*,*,#10446,.T.);
#14568=ORIENTED_EDGE('',*,*,#10445,.F.);
#14569=ORIENTED_EDGE('',*,*,#10447,.F.);
#14570=ORIENTED_EDGE('',*,*,#10448,.T.);
#14571=ORIENTED_EDGE('',*,*,#10449,.T.);
#14572=ORIENTED_EDGE('',*,*,#10448,.F.);
#14573=ORIENTED_EDGE('',*,*,#10450,.F.);
#14574=ORIENTED_EDGE('',*,*,#10451,.T.);
#14575=ORIENTED_EDGE('',*,*,#10452,.T.);
#14576=ORIENTED_EDGE('',*,*,#10451,.F.);
#14577=ORIENTED_EDGE('',*,*,#10453,.F.);
#14578=ORIENTED_EDGE('',*,*,#10454,.T.);
#14579=ORIENTED_EDGE('',*,*,#10455,.T.);
#14580=ORIENTED_EDGE('',*,*,#10454,.F.);
#14581=ORIENTED_EDGE('',*,*,#10456,.F.);
#14582=ORIENTED_EDGE('',*,*,#10457,.T.);
#14583=ORIENTED_EDGE('',*,*,#10458,.T.);
#14584=ORIENTED_EDGE('',*,*,#10457,.F.);
#14585=ORIENTED_EDGE('',*,*,#10459,.F.);
#14586=ORIENTED_EDGE('',*,*,#10460,.T.);
#14587=ORIENTED_EDGE('',*,*,#10461,.T.);
#14588=ORIENTED_EDGE('',*,*,#10460,.F.);
#14589=ORIENTED_EDGE('',*,*,#10462,.F.);
#14590=ORIENTED_EDGE('',*,*,#10463,.T.);
#14591=ORIENTED_EDGE('',*,*,#10464,.T.);
#14592=ORIENTED_EDGE('',*,*,#10463,.F.);
#14593=ORIENTED_EDGE('',*,*,#10465,.F.);
#14594=ORIENTED_EDGE('',*,*,#10466,.T.);
#14595=ORIENTED_EDGE('',*,*,#10467,.T.);
#14596=ORIENTED_EDGE('',*,*,#10466,.F.);
#14597=ORIENTED_EDGE('',*,*,#10468,.F.);
#14598=ORIENTED_EDGE('',*,*,#10469,.T.);
#14599=ORIENTED_EDGE('',*,*,#10470,.T.);
#14600=ORIENTED_EDGE('',*,*,#10469,.F.);
#14601=ORIENTED_EDGE('',*,*,#10471,.F.);
#14602=ORIENTED_EDGE('',*,*,#10472,.T.);
#14603=ORIENTED_EDGE('',*,*,#10473,.T.);
#14604=ORIENTED_EDGE('',*,*,#10472,.F.);
#14605=ORIENTED_EDGE('',*,*,#10474,.F.);
#14606=ORIENTED_EDGE('',*,*,#10475,.T.);
#14607=ORIENTED_EDGE('',*,*,#10476,.T.);
#14608=ORIENTED_EDGE('',*,*,#10475,.F.);
#14609=ORIENTED_EDGE('',*,*,#10477,.F.);
#14610=ORIENTED_EDGE('',*,*,#10478,.T.);
#14611=ORIENTED_EDGE('',*,*,#10479,.T.);
#14612=ORIENTED_EDGE('',*,*,#10478,.F.);
#14613=ORIENTED_EDGE('',*,*,#10480,.F.);
#14614=ORIENTED_EDGE('',*,*,#10481,.T.);
#14615=ORIENTED_EDGE('',*,*,#10482,.T.);
#14616=ORIENTED_EDGE('',*,*,#10481,.F.);
#14617=ORIENTED_EDGE('',*,*,#10483,.F.);
#14618=ORIENTED_EDGE('',*,*,#10484,.T.);
#14619=ORIENTED_EDGE('',*,*,#10485,.T.);
#14620=ORIENTED_EDGE('',*,*,#10484,.F.);
#14621=ORIENTED_EDGE('',*,*,#10486,.F.);
#14622=ORIENTED_EDGE('',*,*,#10487,.T.);
#14623=ORIENTED_EDGE('',*,*,#10488,.T.);
#14624=ORIENTED_EDGE('',*,*,#10487,.F.);
#14625=ORIENTED_EDGE('',*,*,#10489,.F.);
#14626=ORIENTED_EDGE('',*,*,#10490,.T.);
#14627=ORIENTED_EDGE('',*,*,#10491,.T.);
#14628=ORIENTED_EDGE('',*,*,#10490,.F.);
#14629=ORIENTED_EDGE('',*,*,#10492,.F.);
#14630=ORIENTED_EDGE('',*,*,#10493,.T.);
#14631=ORIENTED_EDGE('',*,*,#10494,.T.);
#14632=ORIENTED_EDGE('',*,*,#10493,.F.);
#14633=ORIENTED_EDGE('',*,*,#10495,.F.);
#14634=ORIENTED_EDGE('',*,*,#10496,.T.);
#14635=ORIENTED_EDGE('',*,*,#10497,.T.);
#14636=ORIENTED_EDGE('',*,*,#10496,.F.);
#14637=ORIENTED_EDGE('',*,*,#10498,.F.);
#14638=ORIENTED_EDGE('',*,*,#10499,.T.);
#14639=ORIENTED_EDGE('',*,*,#10500,.T.);
#14640=ORIENTED_EDGE('',*,*,#10499,.F.);
#14641=ORIENTED_EDGE('',*,*,#10501,.F.);
#14642=ORIENTED_EDGE('',*,*,#10502,.T.);
#14643=ORIENTED_EDGE('',*,*,#10503,.T.);
#14644=ORIENTED_EDGE('',*,*,#10502,.F.);
#14645=ORIENTED_EDGE('',*,*,#10504,.F.);
#14646=ORIENTED_EDGE('',*,*,#10505,.T.);
#14647=ORIENTED_EDGE('',*,*,#10506,.T.);
#14648=ORIENTED_EDGE('',*,*,#10505,.F.);
#14649=ORIENTED_EDGE('',*,*,#10507,.F.);
#14650=ORIENTED_EDGE('',*,*,#10508,.T.);
#14651=ORIENTED_EDGE('',*,*,#10509,.T.);
#14652=ORIENTED_EDGE('',*,*,#10508,.F.);
#14653=ORIENTED_EDGE('',*,*,#10510,.F.);
#14654=ORIENTED_EDGE('',*,*,#10511,.T.);
#14655=ORIENTED_EDGE('',*,*,#10512,.T.);
#14656=ORIENTED_EDGE('',*,*,#10511,.F.);
#14657=ORIENTED_EDGE('',*,*,#10513,.F.);
#14658=ORIENTED_EDGE('',*,*,#10514,.T.);
#14659=ORIENTED_EDGE('',*,*,#10515,.T.);
#14660=ORIENTED_EDGE('',*,*,#10514,.F.);
#14661=ORIENTED_EDGE('',*,*,#10516,.F.);
#14662=ORIENTED_EDGE('',*,*,#10517,.T.);
#14663=ORIENTED_EDGE('',*,*,#10518,.T.);
#14664=ORIENTED_EDGE('',*,*,#10517,.F.);
#14665=ORIENTED_EDGE('',*,*,#10519,.F.);
#14666=ORIENTED_EDGE('',*,*,#10520,.T.);
#14667=ORIENTED_EDGE('',*,*,#10521,.T.);
#14668=ORIENTED_EDGE('',*,*,#10520,.F.);
#14669=ORIENTED_EDGE('',*,*,#10522,.F.);
#14670=ORIENTED_EDGE('',*,*,#10523,.T.);
#14671=ORIENTED_EDGE('',*,*,#10524,.T.);
#14672=ORIENTED_EDGE('',*,*,#10523,.F.);
#14673=ORIENTED_EDGE('',*,*,#10525,.F.);
#14674=ORIENTED_EDGE('',*,*,#10526,.T.);
#14675=ORIENTED_EDGE('',*,*,#10527,.T.);
#14676=ORIENTED_EDGE('',*,*,#10526,.F.);
#14677=ORIENTED_EDGE('',*,*,#10528,.F.);
#14678=ORIENTED_EDGE('',*,*,#10529,.T.);
#14679=ORIENTED_EDGE('',*,*,#10530,.T.);
#14680=ORIENTED_EDGE('',*,*,#10529,.F.);
#14681=ORIENTED_EDGE('',*,*,#10531,.F.);
#14682=ORIENTED_EDGE('',*,*,#10532,.T.);
#14683=ORIENTED_EDGE('',*,*,#10533,.T.);
#14684=ORIENTED_EDGE('',*,*,#10532,.F.);
#14685=ORIENTED_EDGE('',*,*,#10534,.F.);
#14686=ORIENTED_EDGE('',*,*,#10535,.T.);
#14687=ORIENTED_EDGE('',*,*,#10536,.T.);
#14688=ORIENTED_EDGE('',*,*,#10535,.F.);
#14689=ORIENTED_EDGE('',*,*,#10537,.F.);
#14690=ORIENTED_EDGE('',*,*,#10538,.T.);
#14691=ORIENTED_EDGE('',*,*,#10539,.T.);
#14692=ORIENTED_EDGE('',*,*,#10538,.F.);
#14693=ORIENTED_EDGE('',*,*,#10540,.F.);
#14694=ORIENTED_EDGE('',*,*,#10541,.T.);
#14695=ORIENTED_EDGE('',*,*,#10542,.T.);
#14696=ORIENTED_EDGE('',*,*,#10541,.F.);
#14697=ORIENTED_EDGE('',*,*,#10543,.F.);
#14698=ORIENTED_EDGE('',*,*,#10544,.T.);
#14699=ORIENTED_EDGE('',*,*,#10545,.T.);
#14700=ORIENTED_EDGE('',*,*,#10544,.F.);
#14701=ORIENTED_EDGE('',*,*,#10546,.F.);
#14702=ORIENTED_EDGE('',*,*,#10547,.T.);
#14703=ORIENTED_EDGE('',*,*,#10548,.T.);
#14704=ORIENTED_EDGE('',*,*,#10547,.F.);
#14705=ORIENTED_EDGE('',*,*,#10549,.F.);
#14706=ORIENTED_EDGE('',*,*,#10550,.T.);
#14707=ORIENTED_EDGE('',*,*,#10551,.T.);
#14708=ORIENTED_EDGE('',*,*,#10550,.F.);
#14709=ORIENTED_EDGE('',*,*,#10552,.F.);
#14710=ORIENTED_EDGE('',*,*,#10553,.T.);
#14711=ORIENTED_EDGE('',*,*,#10554,.T.);
#14712=ORIENTED_EDGE('',*,*,#10553,.F.);
#14713=ORIENTED_EDGE('',*,*,#10555,.F.);
#14714=ORIENTED_EDGE('',*,*,#10287,.T.);
#14715=ORIENTED_EDGE('',*,*,#10555,.T.);
#14716=ORIENTED_EDGE('',*,*,#10552,.T.);
#14717=ORIENTED_EDGE('',*,*,#10549,.T.);
#14718=ORIENTED_EDGE('',*,*,#10546,.T.);
#14719=ORIENTED_EDGE('',*,*,#10543,.T.);
#14720=ORIENTED_EDGE('',*,*,#10540,.T.);
#14721=ORIENTED_EDGE('',*,*,#10537,.T.);
#14722=ORIENTED_EDGE('',*,*,#10534,.T.);
#14723=ORIENTED_EDGE('',*,*,#10531,.T.);
#14724=ORIENTED_EDGE('',*,*,#10528,.T.);
#14725=ORIENTED_EDGE('',*,*,#10525,.T.);
#14726=ORIENTED_EDGE('',*,*,#10522,.T.);
#14727=ORIENTED_EDGE('',*,*,#10519,.T.);
#14728=ORIENTED_EDGE('',*,*,#10516,.T.);
#14729=ORIENTED_EDGE('',*,*,#10513,.T.);
#14730=ORIENTED_EDGE('',*,*,#10510,.T.);
#14731=ORIENTED_EDGE('',*,*,#10507,.T.);
#14732=ORIENTED_EDGE('',*,*,#10504,.T.);
#14733=ORIENTED_EDGE('',*,*,#10501,.T.);
#14734=ORIENTED_EDGE('',*,*,#10498,.T.);
#14735=ORIENTED_EDGE('',*,*,#10495,.T.);
#14736=ORIENTED_EDGE('',*,*,#10492,.T.);
#14737=ORIENTED_EDGE('',*,*,#10489,.T.);
#14738=ORIENTED_EDGE('',*,*,#10486,.T.);
#14739=ORIENTED_EDGE('',*,*,#10483,.T.);
#14740=ORIENTED_EDGE('',*,*,#10480,.T.);
#14741=ORIENTED_EDGE('',*,*,#10477,.T.);
#14742=ORIENTED_EDGE('',*,*,#10474,.T.);
#14743=ORIENTED_EDGE('',*,*,#10471,.T.);
#14744=ORIENTED_EDGE('',*,*,#10468,.T.);
#14745=ORIENTED_EDGE('',*,*,#10465,.T.);
#14746=ORIENTED_EDGE('',*,*,#10462,.T.);
#14747=ORIENTED_EDGE('',*,*,#10459,.T.);
#14748=ORIENTED_EDGE('',*,*,#10456,.T.);
#14749=ORIENTED_EDGE('',*,*,#10453,.T.);
#14750=ORIENTED_EDGE('',*,*,#10450,.T.);
#14751=ORIENTED_EDGE('',*,*,#10447,.T.);
#14752=ORIENTED_EDGE('',*,*,#10444,.T.);
#14753=ORIENTED_EDGE('',*,*,#10441,.T.);
#14754=ORIENTED_EDGE('',*,*,#10438,.T.);
#14755=ORIENTED_EDGE('',*,*,#10435,.T.);
#14756=ORIENTED_EDGE('',*,*,#10432,.T.);
#14757=ORIENTED_EDGE('',*,*,#10429,.T.);
#14758=ORIENTED_EDGE('',*,*,#10426,.T.);
#14759=ORIENTED_EDGE('',*,*,#10423,.T.);
#14760=ORIENTED_EDGE('',*,*,#10420,.T.);
#14761=ORIENTED_EDGE('',*,*,#10417,.T.);
#14762=ORIENTED_EDGE('',*,*,#10414,.T.);
#14763=ORIENTED_EDGE('',*,*,#10411,.T.);
#14764=ORIENTED_EDGE('',*,*,#10408,.T.);
#14765=ORIENTED_EDGE('',*,*,#10405,.T.);
#14766=ORIENTED_EDGE('',*,*,#10402,.T.);
#14767=ORIENTED_EDGE('',*,*,#10399,.T.);
#14768=ORIENTED_EDGE('',*,*,#10396,.T.);
#14769=ORIENTED_EDGE('',*,*,#10393,.T.);
#14770=ORIENTED_EDGE('',*,*,#10390,.T.);
#14771=ORIENTED_EDGE('',*,*,#10387,.T.);
#14772=ORIENTED_EDGE('',*,*,#10384,.T.);
#14773=ORIENTED_EDGE('',*,*,#10381,.T.);
#14774=ORIENTED_EDGE('',*,*,#10378,.T.);
#14775=ORIENTED_EDGE('',*,*,#10375,.T.);
#14776=ORIENTED_EDGE('',*,*,#10372,.T.);
#14777=ORIENTED_EDGE('',*,*,#10369,.T.);
#14778=ORIENTED_EDGE('',*,*,#10366,.T.);
#14779=ORIENTED_EDGE('',*,*,#10363,.T.);
#14780=ORIENTED_EDGE('',*,*,#10360,.T.);
#14781=ORIENTED_EDGE('',*,*,#10357,.T.);
#14782=ORIENTED_EDGE('',*,*,#10354,.T.);
#14783=ORIENTED_EDGE('',*,*,#10351,.T.);
#14784=ORIENTED_EDGE('',*,*,#10348,.T.);
#14785=ORIENTED_EDGE('',*,*,#10345,.T.);
#14786=ORIENTED_EDGE('',*,*,#10342,.T.);
#14787=ORIENTED_EDGE('',*,*,#10339,.T.);
#14788=ORIENTED_EDGE('',*,*,#10336,.T.);
#14789=ORIENTED_EDGE('',*,*,#10333,.T.);
#14790=ORIENTED_EDGE('',*,*,#10330,.T.);
#14791=ORIENTED_EDGE('',*,*,#10327,.T.);
#14792=ORIENTED_EDGE('',*,*,#10324,.T.);
#14793=ORIENTED_EDGE('',*,*,#10321,.T.);
#14794=ORIENTED_EDGE('',*,*,#10318,.T.);
#14795=ORIENTED_EDGE('',*,*,#10315,.T.);
#14796=ORIENTED_EDGE('',*,*,#10312,.T.);
#14797=ORIENTED_EDGE('',*,*,#10309,.T.);
#14798=ORIENTED_EDGE('',*,*,#10306,.T.);
#14799=ORIENTED_EDGE('',*,*,#10303,.T.);
#14800=ORIENTED_EDGE('',*,*,#10300,.T.);
#14801=ORIENTED_EDGE('',*,*,#10297,.T.);
#14802=ORIENTED_EDGE('',*,*,#10294,.T.);
#14803=ORIENTED_EDGE('',*,*,#10291,.T.);
#14804=ORIENTED_EDGE('',*,*,#10288,.T.);
#14805=ORIENTED_EDGE('',*,*,#10269,.F.);
#14806=ORIENTED_EDGE('',*,*,#10276,.F.);
#14807=ORIENTED_EDGE('',*,*,#10280,.F.);
#14808=ORIENTED_EDGE('',*,*,#10272,.F.);
#14809=ORIENTED_EDGE('',*,*,#10249,.F.);
#14810=ORIENTED_EDGE('',*,*,#10554,.F.);
#14811=ORIENTED_EDGE('',*,*,#10286,.F.);
#14812=ORIENTED_EDGE('',*,*,#10290,.F.);
#14813=ORIENTED_EDGE('',*,*,#10293,.F.);
#14814=ORIENTED_EDGE('',*,*,#10296,.F.);
#14815=ORIENTED_EDGE('',*,*,#10299,.F.);
#14816=ORIENTED_EDGE('',*,*,#10302,.F.);
#14817=ORIENTED_EDGE('',*,*,#10305,.F.);
#14818=ORIENTED_EDGE('',*,*,#10308,.F.);
#14819=ORIENTED_EDGE('',*,*,#10311,.F.);
#14820=ORIENTED_EDGE('',*,*,#10314,.F.);
#14821=ORIENTED_EDGE('',*,*,#10317,.F.);
#14822=ORIENTED_EDGE('',*,*,#10320,.F.);
#14823=ORIENTED_EDGE('',*,*,#10323,.F.);
#14824=ORIENTED_EDGE('',*,*,#10326,.F.);
#14825=ORIENTED_EDGE('',*,*,#10329,.F.);
#14826=ORIENTED_EDGE('',*,*,#10332,.F.);
#14827=ORIENTED_EDGE('',*,*,#10335,.F.);
#14828=ORIENTED_EDGE('',*,*,#10338,.F.);
#14829=ORIENTED_EDGE('',*,*,#10341,.F.);
#14830=ORIENTED_EDGE('',*,*,#10344,.F.);
#14831=ORIENTED_EDGE('',*,*,#10347,.F.);
#14832=ORIENTED_EDGE('',*,*,#10350,.F.);
#14833=ORIENTED_EDGE('',*,*,#10353,.F.);
#14834=ORIENTED_EDGE('',*,*,#10356,.F.);
#14835=ORIENTED_EDGE('',*,*,#10359,.F.);
#14836=ORIENTED_EDGE('',*,*,#10362,.F.);
#14837=ORIENTED_EDGE('',*,*,#10365,.F.);
#14838=ORIENTED_EDGE('',*,*,#10368,.F.);
#14839=ORIENTED_EDGE('',*,*,#10371,.F.);
#14840=ORIENTED_EDGE('',*,*,#10374,.F.);
#14841=ORIENTED_EDGE('',*,*,#10377,.F.);
#14842=ORIENTED_EDGE('',*,*,#10380,.F.);
#14843=ORIENTED_EDGE('',*,*,#10383,.F.);
#14844=ORIENTED_EDGE('',*,*,#10386,.F.);
#14845=ORIENTED_EDGE('',*,*,#10389,.F.);
#14846=ORIENTED_EDGE('',*,*,#10392,.F.);
#14847=ORIENTED_EDGE('',*,*,#10395,.F.);
#14848=ORIENTED_EDGE('',*,*,#10398,.F.);
#14849=ORIENTED_EDGE('',*,*,#10401,.F.);
#14850=ORIENTED_EDGE('',*,*,#10404,.F.);
#14851=ORIENTED_EDGE('',*,*,#10407,.F.);
#14852=ORIENTED_EDGE('',*,*,#10410,.F.);
#14853=ORIENTED_EDGE('',*,*,#10413,.F.);
#14854=ORIENTED_EDGE('',*,*,#10416,.F.);
#14855=ORIENTED_EDGE('',*,*,#10419,.F.);
#14856=ORIENTED_EDGE('',*,*,#10422,.F.);
#14857=ORIENTED_EDGE('',*,*,#10425,.F.);
#14858=ORIENTED_EDGE('',*,*,#10428,.F.);
#14859=ORIENTED_EDGE('',*,*,#10431,.F.);
#14860=ORIENTED_EDGE('',*,*,#10434,.F.);
#14861=ORIENTED_EDGE('',*,*,#10437,.F.);
#14862=ORIENTED_EDGE('',*,*,#10440,.F.);
#14863=ORIENTED_EDGE('',*,*,#10443,.F.);
#14864=ORIENTED_EDGE('',*,*,#10446,.F.);
#14865=ORIENTED_EDGE('',*,*,#10449,.F.);
#14866=ORIENTED_EDGE('',*,*,#10452,.F.);
#14867=ORIENTED_EDGE('',*,*,#10455,.F.);
#14868=ORIENTED_EDGE('',*,*,#10458,.F.);
#14869=ORIENTED_EDGE('',*,*,#10461,.F.);
#14870=ORIENTED_EDGE('',*,*,#10464,.F.);
#14871=ORIENTED_EDGE('',*,*,#10467,.F.);
#14872=ORIENTED_EDGE('',*,*,#10470,.F.);
#14873=ORIENTED_EDGE('',*,*,#10473,.F.);
#14874=ORIENTED_EDGE('',*,*,#10476,.F.);
#14875=ORIENTED_EDGE('',*,*,#10479,.F.);
#14876=ORIENTED_EDGE('',*,*,#10482,.F.);
#14877=ORIENTED_EDGE('',*,*,#10485,.F.);
#14878=ORIENTED_EDGE('',*,*,#10488,.F.);
#14879=ORIENTED_EDGE('',*,*,#10491,.F.);
#14880=ORIENTED_EDGE('',*,*,#10494,.F.);
#14881=ORIENTED_EDGE('',*,*,#10497,.F.);
#14882=ORIENTED_EDGE('',*,*,#10500,.F.);
#14883=ORIENTED_EDGE('',*,*,#10503,.F.);
#14884=ORIENTED_EDGE('',*,*,#10506,.F.);
#14885=ORIENTED_EDGE('',*,*,#10509,.F.);
#14886=ORIENTED_EDGE('',*,*,#10512,.F.);
#14887=ORIENTED_EDGE('',*,*,#10515,.F.);
#14888=ORIENTED_EDGE('',*,*,#10518,.F.);
#14889=ORIENTED_EDGE('',*,*,#10521,.F.);
#14890=ORIENTED_EDGE('',*,*,#10524,.F.);
#14891=ORIENTED_EDGE('',*,*,#10527,.F.);
#14892=ORIENTED_EDGE('',*,*,#10530,.F.);
#14893=ORIENTED_EDGE('',*,*,#10533,.F.);
#14894=ORIENTED_EDGE('',*,*,#10536,.F.);
#14895=ORIENTED_EDGE('',*,*,#10539,.F.);
#14896=ORIENTED_EDGE('',*,*,#10542,.F.);
#14897=ORIENTED_EDGE('',*,*,#10545,.F.);
#14898=ORIENTED_EDGE('',*,*,#10548,.F.);
#14899=ORIENTED_EDGE('',*,*,#10551,.F.);
#14900=ORIENTED_EDGE('',*,*,#10254,.F.);
#14901=ORIENTED_EDGE('',*,*,#10278,.T.);
#14902=ORIENTED_EDGE('',*,*,#10279,.T.);
#14903=ORIENTED_EDGE('',*,*,#10262,.F.);
#14904=ORIENTED_EDGE('',*,*,#10282,.T.);
#14905=ORIENTED_EDGE('',*,*,#10283,.T.);
#14906=ORIENTED_EDGE('',*,*,#10260,.F.);
#14907=ORIENTED_EDGE('',*,*,#10271,.T.);
#14908=ORIENTED_EDGE('',*,*,#10256,.F.);
#14909=ORIENTED_EDGE('',*,*,#10274,.T.);
#14910=ORIENTED_EDGE('',*,*,#10275,.T.);
#14911=ORIENTED_EDGE('',*,*,#10105,.T.);
#14912=ORIENTED_EDGE('',*,*,#10229,.T.);
#14913=ORIENTED_EDGE('',*,*,#10263,.T.);
#14914=ORIENTED_EDGE('',*,*,#10230,.F.);
#14915=ORIENTED_EDGE('',*,*,#10236,.T.);
#14916=ORIENTED_EDGE('',*,*,#10556,.T.);
#14917=ORIENTED_EDGE('',*,*,#10285,.F.);
#14918=ORIENTED_EDGE('',*,*,#10557,.F.);
#14919=ORIENTED_EDGE('',*,*,#10558,.T.);
#14920=ORIENTED_EDGE('',*,*,#10559,.T.);
#14921=ORIENTED_EDGE('',*,*,#10560,.T.);
#14922=ORIENTED_EDGE('',*,*,#10556,.F.);
#14923=ORIENTED_EDGE('',*,*,#10560,.F.);
#14924=ORIENTED_EDGE('',*,*,#10561,.F.);
#14925=ORIENTED_EDGE('',*,*,#9977,.T.);
#14926=ORIENTED_EDGE('',*,*,#9980,.T.);
#14927=ORIENTED_EDGE('',*,*,#9983,.T.);
#14928=ORIENTED_EDGE('',*,*,#9986,.T.);
#14929=ORIENTED_EDGE('',*,*,#9989,.T.);
#14930=ORIENTED_EDGE('',*,*,#9992,.T.);
#14931=ORIENTED_EDGE('',*,*,#9995,.T.);
#14932=ORIENTED_EDGE('',*,*,#9998,.T.);
#14933=ORIENTED_EDGE('',*,*,#10001,.T.);
#14934=ORIENTED_EDGE('',*,*,#10004,.T.);
#14935=ORIENTED_EDGE('',*,*,#10007,.T.);
#14936=ORIENTED_EDGE('',*,*,#10010,.T.);
#14937=ORIENTED_EDGE('',*,*,#10013,.T.);
#14938=ORIENTED_EDGE('',*,*,#10016,.T.);
#14939=ORIENTED_EDGE('',*,*,#10019,.T.);
#14940=ORIENTED_EDGE('',*,*,#10022,.T.);
#14941=ORIENTED_EDGE('',*,*,#10025,.T.);
#14942=ORIENTED_EDGE('',*,*,#10562,.T.);
#14943=ORIENTED_EDGE('',*,*,#10030,.T.);
#14944=ORIENTED_EDGE('',*,*,#10563,.T.);
#14945=ORIENTED_EDGE('',*,*,#10035,.T.);
#14946=ORIENTED_EDGE('',*,*,#10564,.F.);
#14947=ORIENTED_EDGE('',*,*,#10037,.F.);
#14948=ORIENTED_EDGE('',*,*,#10041,.F.);
#14949=ORIENTED_EDGE('',*,*,#10044,.F.);
#14950=ORIENTED_EDGE('',*,*,#10047,.F.);
#14951=ORIENTED_EDGE('',*,*,#10050,.F.);
#14952=ORIENTED_EDGE('',*,*,#10053,.F.);
#14953=ORIENTED_EDGE('',*,*,#10056,.F.);
#14954=ORIENTED_EDGE('',*,*,#10059,.F.);
#14955=ORIENTED_EDGE('',*,*,#10062,.F.);
#14956=ORIENTED_EDGE('',*,*,#10065,.F.);
#14957=ORIENTED_EDGE('',*,*,#10068,.F.);
#14958=ORIENTED_EDGE('',*,*,#10071,.F.);
#14959=ORIENTED_EDGE('',*,*,#10074,.F.);
#14960=ORIENTED_EDGE('',*,*,#10077,.F.);
#14961=ORIENTED_EDGE('',*,*,#10080,.F.);
#14962=ORIENTED_EDGE('',*,*,#10083,.F.);
#14963=ORIENTED_EDGE('',*,*,#10086,.F.);
#14964=ORIENTED_EDGE('',*,*,#10089,.F.);
#14965=ORIENTED_EDGE('',*,*,#10092,.F.);
#14966=ORIENTED_EDGE('',*,*,#10565,.F.);
#14967=ORIENTED_EDGE('',*,*,#10097,.F.);
#14968=ORIENTED_EDGE('',*,*,#10094,.T.);
#14969=ORIENTED_EDGE('',*,*,#10565,.T.);
#14970=ORIENTED_EDGE('',*,*,#10091,.F.);
#14971=ORIENTED_EDGE('',*,*,#10566,.F.);
#14972=ORIENTED_EDGE('',*,*,#10567,.F.);
#14973=ORIENTED_EDGE('',*,*,#10095,.T.);
#14974=ORIENTED_EDGE('',*,*,#10566,.T.);
#14975=ORIENTED_EDGE('',*,*,#10093,.T.);
#14976=ORIENTED_EDGE('',*,*,#10090,.T.);
#14977=ORIENTED_EDGE('',*,*,#10087,.T.);
#14978=ORIENTED_EDGE('',*,*,#10084,.T.);
#14979=ORIENTED_EDGE('',*,*,#10081,.T.);
#14980=ORIENTED_EDGE('',*,*,#10078,.T.);
#14981=ORIENTED_EDGE('',*,*,#10075,.T.);
#14982=ORIENTED_EDGE('',*,*,#10072,.T.);
#14983=ORIENTED_EDGE('',*,*,#10069,.T.);
#14984=ORIENTED_EDGE('',*,*,#10066,.T.);
#14985=ORIENTED_EDGE('',*,*,#10063,.T.);
#14986=ORIENTED_EDGE('',*,*,#10060,.T.);
#14987=ORIENTED_EDGE('',*,*,#10057,.T.);
#14988=ORIENTED_EDGE('',*,*,#10054,.T.);
#14989=ORIENTED_EDGE('',*,*,#10051,.T.);
#14990=ORIENTED_EDGE('',*,*,#10048,.T.);
#14991=ORIENTED_EDGE('',*,*,#10045,.T.);
#14992=ORIENTED_EDGE('',*,*,#10042,.T.);
#14993=ORIENTED_EDGE('',*,*,#10039,.T.);
#14994=ORIENTED_EDGE('',*,*,#10568,.F.);
#14995=ORIENTED_EDGE('',*,*,#10033,.F.);
#14996=ORIENTED_EDGE('',*,*,#10028,.F.);
#14997=ORIENTED_EDGE('',*,*,#10569,.F.);
#14998=ORIENTED_EDGE('',*,*,#10026,.F.);
#14999=ORIENTED_EDGE('',*,*,#10023,.F.);
#15000=ORIENTED_EDGE('',*,*,#10020,.F.);
#15001=ORIENTED_EDGE('',*,*,#10017,.F.);
#15002=ORIENTED_EDGE('',*,*,#10014,.F.);
#15003=ORIENTED_EDGE('',*,*,#10011,.F.);
#15004=ORIENTED_EDGE('',*,*,#10008,.F.);
#15005=ORIENTED_EDGE('',*,*,#10005,.F.);
#15006=ORIENTED_EDGE('',*,*,#10002,.F.);
#15007=ORIENTED_EDGE('',*,*,#9999,.F.);
#15008=ORIENTED_EDGE('',*,*,#9996,.F.);
#15009=ORIENTED_EDGE('',*,*,#9993,.F.);
#15010=ORIENTED_EDGE('',*,*,#9990,.F.);
#15011=ORIENTED_EDGE('',*,*,#9987,.F.);
#15012=ORIENTED_EDGE('',*,*,#9984,.F.);
#15013=ORIENTED_EDGE('',*,*,#9981,.F.);
#15014=ORIENTED_EDGE('',*,*,#9978,.F.);
#15015=ORIENTED_EDGE('',*,*,#9975,.F.);
#15016=ORIENTED_EDGE('',*,*,#10570,.F.);
#15017=ORIENTED_EDGE('',*,*,#10568,.T.);
#15018=ORIENTED_EDGE('',*,*,#10038,.T.);
#15019=ORIENTED_EDGE('',*,*,#10564,.T.);
#15020=ORIENTED_EDGE('',*,*,#10034,.T.);
#15021=ORIENTED_EDGE('',*,*,#10567,.T.);
#15022=ORIENTED_EDGE('',*,*,#10571,.T.);
#15023=ORIENTED_EDGE('',*,*,#9973,.T.);
#15024=ORIENTED_EDGE('',*,*,#10561,.T.);
#15025=ORIENTED_EDGE('',*,*,#10096,.T.);
#15026=ORIENTED_EDGE('',*,*,#10031,.T.);
#15027=ORIENTED_EDGE('',*,*,#10563,.F.);
#15028=ORIENTED_EDGE('',*,*,#10572,.T.);
#15029=ORIENTED_EDGE('',*,*,#10570,.T.);
#15030=ORIENTED_EDGE('',*,*,#10573,.T.);
#15031=ORIENTED_EDGE('',*,*,#10571,.F.);
#15032=ORIENTED_EDGE('',*,*,#10572,.F.);
#15033=ORIENTED_EDGE('',*,*,#10029,.F.);
#15034=ORIENTED_EDGE('',*,*,#10032,.F.);
#15035=ORIENTED_EDGE('',*,*,#10574,.T.);
#15036=ORIENTED_EDGE('',*,*,#10575,.F.);
#15037=ORIENTED_EDGE('',*,*,#10574,.F.);
#15038=ORIENTED_EDGE('',*,*,#10573,.F.);
#15039=ORIENTED_EDGE('',*,*,#9974,.F.);
#15040=ORIENTED_EDGE('',*,*,#10576,.T.);
#15041=ORIENTED_EDGE('',*,*,#10577,.F.);
#15042=ORIENTED_EDGE('',*,*,#10576,.F.);
#15043=ORIENTED_EDGE('',*,*,#10558,.F.);
#15044=ORIENTED_EDGE('',*,*,#10559,.F.);
#15045=ORIENTED_EDGE('',*,*,#10578,.T.);
#15046=ORIENTED_EDGE('',*,*,#10579,.F.);
#15047=ORIENTED_EDGE('',*,*,#10578,.F.);
#15048=ORIENTED_EDGE('',*,*,#10580,.F.);
#15049=ORIENTED_EDGE('',*,*,#10581,.T.);
#15050=ORIENTED_EDGE('',*,*,#10582,.F.);
#15051=ORIENTED_EDGE('',*,*,#10581,.F.);
#15052=ORIENTED_EDGE('',*,*,#10557,.T.);
#15053=ORIENTED_EDGE('',*,*,#10583,.T.);
#15054=ORIENTED_EDGE('',*,*,#10580,.T.);
#15055=ORIENTED_EDGE('',*,*,#10583,.F.);
#15056=ORIENTED_EDGE('',*,*,#10579,.T.);
#15057=ORIENTED_EDGE('',*,*,#10577,.T.);
#15058=ORIENTED_EDGE('',*,*,#10582,.T.);
#15059=ORIENTED_EDGE('',*,*,#10575,.T.);
#15060=ORIENTED_EDGE('',*,*,#10027,.T.);
#15061=ORIENTED_EDGE('',*,*,#10562,.F.);
#15062=ORIENTED_EDGE('',*,*,#10024,.F.);
#15063=ORIENTED_EDGE('',*,*,#10569,.T.);
#16584=PLANE('',#18850);
#16585=PLANE('',#18852);
#16586=PLANE('',#18853);
#16587=PLANE('',#18854);
#16588=PLANE('',#18855);
#16589=PLANE('',#18857);
#16590=PLANE('',#18858);
#16591=PLANE('',#18859);
#16592=PLANE('',#18860);
#16593=PLANE('',#18862);
#16594=PLANE('',#18863);
#16595=PLANE('',#18864);
#16596=PLANE('',#18865);
#16597=PLANE('',#18868);
#16598=PLANE('',#18869);
#16599=PLANE('',#18870);
#16600=PLANE('',#18874);
#16601=PLANE('',#18881);
#16602=PLANE('',#18898);
#16603=PLANE('',#18899);
#16604=PLANE('',#18900);
#16605=PLANE('',#18901);
#16606=PLANE('',#18902);
#16607=PLANE('',#18910);
#16608=PLANE('',#18924);
#16609=PLANE('',#18925);
#16610=PLANE('',#18937);
#16611=PLANE('',#18939);
#16612=PLANE('',#18942);
#16613=PLANE('',#18944);
#16614=PLANE('',#18946);
#16615=PLANE('',#18965);
#16616=PLANE('',#18966);
#16617=PLANE('',#18967);
#16618=PLANE('',#18968);
#16619=PLANE('',#18969);
#16620=PLANE('',#18970);
#16621=PLANE('',#18971);
#16622=PLANE('',#18972);
#16623=PLANE('',#18973);
#16624=PLANE('',#18974);
#16625=PLANE('',#18975);
#16626=PLANE('',#18976);
#16627=PLANE('',#18977);
#16628=PLANE('',#18978);
#16629=PLANE('',#18979);
#16630=PLANE('',#18980);
#16631=PLANE('',#18981);
#16632=PLANE('',#18982);
#16633=PLANE('',#18983);
#16634=PLANE('',#18984);
#16635=PLANE('',#18985);
#16636=PLANE('',#18986);
#16637=PLANE('',#18987);
#16638=PLANE('',#18988);
#16639=PLANE('',#18989);
#16640=PLANE('',#18990);
#16641=PLANE('',#18991);
#16642=PLANE('',#18992);
#16643=PLANE('',#18993);
#16644=PLANE('',#18994);
#16645=PLANE('',#18995);
#16646=PLANE('',#18996);
#16647=PLANE('',#18997);
#16648=PLANE('',#18998);
#16649=PLANE('',#18999);
#16650=PLANE('',#19000);
#16651=PLANE('',#19001);
#16652=PLANE('',#19002);
#16653=PLANE('',#19003);
#16654=PLANE('',#19004);
#16655=PLANE('',#19005);
#16656=PLANE('',#19006);
#16657=PLANE('',#19007);
#16658=PLANE('',#19008);
#16659=PLANE('',#19009);
#16660=PLANE('',#19010);
#16661=PLANE('',#19011);
#16662=PLANE('',#19012);
#16663=PLANE('',#19013);
#16664=PLANE('',#19014);
#16665=PLANE('',#19015);
#16666=PLANE('',#19016);
#16667=PLANE('',#19017);
#16668=PLANE('',#19018);
#16669=PLANE('',#19019);
#16670=PLANE('',#19020);
#16671=PLANE('',#19021);
#16672=PLANE('',#19022);
#16673=PLANE('',#19023);
#16674=PLANE('',#19024);
#16675=PLANE('',#19025);
#16676=PLANE('',#19026);
#16677=PLANE('',#19027);
#16678=PLANE('',#19028);
#16679=PLANE('',#19029);
#16680=PLANE('',#19030);
#16681=PLANE('',#19031);
#16682=PLANE('',#19032);
#16683=PLANE('',#19033);
#16684=PLANE('',#19034);
#16685=PLANE('',#19035);
#16686=PLANE('',#19036);
#16687=PLANE('',#19037);
#16688=PLANE('',#19038);
#16689=PLANE('',#19039);
#16690=PLANE('',#19040);
#16691=PLANE('',#19041);
#16692=PLANE('',#19042);
#16693=PLANE('',#19043);
#16694=PLANE('',#19044);
#16695=PLANE('',#19045);
#16696=PLANE('',#19046);
#16697=PLANE('',#19047);
#16698=PLANE('',#19048);
#16699=PLANE('',#19049);
#16700=PLANE('',#19050);
#16701=PLANE('',#19051);
#16702=PLANE('',#19052);
#16703=PLANE('',#19053);
#16704=PLANE('',#19054);
#16705=PLANE('',#19055);
#16706=PLANE('',#19056);
#16707=PLANE('',#19058);
#16708=PLANE('',#19060);
#16709=PLANE('',#19066);
#16710=PLANE('',#19067);
#16711=PLANE('',#19082);
#16712=PLANE('',#19083);
#17331=ADVANCED_FACE('',(#1996),#622,.F.);
#17332=ADVANCED_FACE('',(#1997),#623,.F.);
#17333=ADVANCED_FACE('',(#1998),#624,.F.);
#17334=ADVANCED_FACE('',(#1999),#625,.F.);
#17335=ADVANCED_FACE('',(#2000),#626,.F.);
#17336=ADVANCED_FACE('',(#2001),#627,.F.);
#17337=ADVANCED_FACE('',(#2002),#628,.F.);
#17338=ADVANCED_FACE('',(#2003),#629,.F.);
#17339=ADVANCED_FACE('',(#2004),#630,.F.);
#17340=ADVANCED_FACE('',(#2005),#631,.F.);
#17341=ADVANCED_FACE('',(#2006),#632,.F.);
#17342=ADVANCED_FACE('',(#2007),#633,.F.);
#17343=ADVANCED_FACE('',(#2008),#634,.F.);
#17344=ADVANCED_FACE('',(#2009),#635,.F.);
#17345=ADVANCED_FACE('',(#2010),#636,.F.);
#17346=ADVANCED_FACE('',(#2011),#637,.F.);
#17347=ADVANCED_FACE('',(#2012),#638,.F.);
#17348=ADVANCED_FACE('',(#2013),#639,.F.);
#17349=ADVANCED_FACE('',(#2014),#640,.F.);
#17350=ADVANCED_FACE('',(#2015),#641,.T.);
#17351=ADVANCED_FACE('',(#2016),#642,.F.);
#17352=ADVANCED_FACE('',(#2017),#643,.F.);
#17353=ADVANCED_FACE('',(#2018),#644,.F.);
#17354=ADVANCED_FACE('',(#2019),#645,.F.);
#17355=ADVANCED_FACE('',(#2020),#646,.F.);
#17356=ADVANCED_FACE('',(#2021),#647,.F.);
#17357=ADVANCED_FACE('',(#2022),#648,.F.);
#17358=ADVANCED_FACE('',(#2023),#649,.F.);
#17359=ADVANCED_FACE('',(#2024),#650,.F.);
#17360=ADVANCED_FACE('',(#2025),#651,.F.);
#17361=ADVANCED_FACE('',(#2026),#652,.F.);
#17362=ADVANCED_FACE('',(#2027),#653,.F.);
#17363=ADVANCED_FACE('',(#2028),#654,.F.);
#17364=ADVANCED_FACE('',(#2029),#655,.F.);
#17365=ADVANCED_FACE('',(#2030),#656,.F.);
#17366=ADVANCED_FACE('',(#2031),#657,.F.);
#17367=ADVANCED_FACE('',(#2032),#658,.F.);
#17368=ADVANCED_FACE('',(#2033),#659,.F.);
#17369=ADVANCED_FACE('',(#2034),#660,.F.);
#17370=ADVANCED_FACE('',(#2035),#661,.F.);
#17371=ADVANCED_FACE('',(#2036),#662,.T.);
#17372=ADVANCED_FACE('',(#2037),#663,.T.);
#17373=ADVANCED_FACE('',(#2038),#664,.T.);
#17374=ADVANCED_FACE('',(#2039),#665,.T.);
#17375=ADVANCED_FACE('',(#2040),#666,.T.);
#17376=ADVANCED_FACE('',(#2041),#667,.T.);
#17377=ADVANCED_FACE('',(#2042),#668,.T.);
#17378=ADVANCED_FACE('',(#2043),#669,.T.);
#17379=ADVANCED_FACE('',(#2044),#670,.T.);
#17380=ADVANCED_FACE('',(#2045),#671,.T.);
#17381=ADVANCED_FACE('',(#2046),#672,.T.);
#17382=ADVANCED_FACE('',(#2047),#673,.F.);
#17383=ADVANCED_FACE('',(#2048),#674,.F.);
#17384=ADVANCED_FACE('',(#2049),#675,.F.);
#17385=ADVANCED_FACE('',(#2050),#676,.F.);
#17386=ADVANCED_FACE('',(#2051),#677,.F.);
#17387=ADVANCED_FACE('',(#2052),#16584,.F.);
#17388=ADVANCED_FACE('',(#2053),#16585,.F.);
#17389=ADVANCED_FACE('',(#2054),#16586,.F.);
#17390=ADVANCED_FACE('',(#2055),#16587,.F.);
#17391=ADVANCED_FACE('',(#2056),#16588,.T.);
#17392=ADVANCED_FACE('',(#2057),#16589,.F.);
#17393=ADVANCED_FACE('',(#2058),#16590,.F.);
#17394=ADVANCED_FACE('',(#2059),#16591,.F.);
#17395=ADVANCED_FACE('',(#2060),#16592,.T.);
#17396=ADVANCED_FACE('',(#2061),#16593,.F.);
#17397=ADVANCED_FACE('',(#2062),#16594,.F.);
#17398=ADVANCED_FACE('',(#2063),#16595,.F.);
#17399=ADVANCED_FACE('',(#2064),#16596,.T.);
#17400=ADVANCED_FACE('',(#2065),#16597,.F.);
#17401=ADVANCED_FACE('',(#2066),#16598,.F.);
#17402=ADVANCED_FACE('',(#2067),#16599,.F.);
#17403=ADVANCED_FACE('',(#2068),#678,.T.);
#17404=ADVANCED_FACE('',(#2069),#16600,.T.);
#17405=ADVANCED_FACE('',(#2070),#679,.T.);
#17406=ADVANCED_FACE('',(#2071,#927),#16601,.T.);
#17407=ADVANCED_FACE('',(#2072),#680,.F.);
#17408=ADVANCED_FACE('',(#2073),#227,.T.);
#17409=ADVANCED_FACE('',(#2074),#184,.T.);
#17410=ADVANCED_FACE('',(#2075),#681,.T.);
#17411=ADVANCED_FACE('',(#2076),#682,.T.);
#17412=ADVANCED_FACE('',(#2077),#683,.T.);
#17413=ADVANCED_FACE('',(#2078),#16602,.T.);
#17414=ADVANCED_FACE('',(#2079),#16603,.T.);
#17415=ADVANCED_FACE('',(#2080),#16604,.T.);
#17416=ADVANCED_FACE('',(#2081),#411,.T.);
#17417=ADVANCED_FACE('',(#2082),#412,.T.);
#17418=ADVANCED_FACE('',(#2083),#16605,.F.);
#17419=ADVANCED_FACE('',(#2084,#928),#16606,.T.);
#17420=ADVANCED_FACE('',(#2085),#684,.F.);
#17421=ADVANCED_FACE('',(#2086),#685,.F.);
#17422=ADVANCED_FACE('',(#2087),#686,.T.);
#17423=ADVANCED_FACE('',(#2088),#16607,.F.);
#17424=ADVANCED_FACE('',(#2089),#228,.T.);
#17425=ADVANCED_FACE('',(#2090),#229,.T.);
#17426=ADVANCED_FACE('',(#2091),#687,.F.);
#17427=ADVANCED_FACE('',(#2092),#688,.T.);
#17428=ADVANCED_FACE('',(#2093,#929),#16608,.T.);
#17429=ADVANCED_FACE('',(#2094,#930),#16609,.F.);
#17430=ADVANCED_FACE('',(#2095),#689,.T.);
#17431=ADVANCED_FACE('',(#2096,#931),#16610,.T.);
#17432=ADVANCED_FACE('',(#2097),#16611,.F.);
#17433=ADVANCED_FACE('',(#2098),#16612,.F.);
#17434=ADVANCED_FACE('',(#2099),#16613,.F.);
#17435=ADVANCED_FACE('',(#2100),#16614,.F.);
#17436=ADVANCED_FACE('',(#2101),#690,.F.);
#17437=ADVANCED_FACE('',(#2102),#691,.F.);
#17438=ADVANCED_FACE('',(#2103),#692,.F.);
#17439=ADVANCED_FACE('',(#2104),#693,.F.);
#17440=ADVANCED_FACE('',(#2105),#694,.F.);
#17441=ADVANCED_FACE('',(#2106),#16615,.F.);
#17442=ADVANCED_FACE('',(#2107),#16616,.F.);
#17443=ADVANCED_FACE('',(#2108),#16617,.F.);
#17444=ADVANCED_FACE('',(#2109),#16618,.F.);
#17445=ADVANCED_FACE('',(#2110),#16619,.F.);
#17446=ADVANCED_FACE('',(#2111),#16620,.F.);
#17447=ADVANCED_FACE('',(#2112),#16621,.F.);
#17448=ADVANCED_FACE('',(#2113),#16622,.F.);
#17449=ADVANCED_FACE('',(#2114),#16623,.F.);
#17450=ADVANCED_FACE('',(#2115),#16624,.F.);
#17451=ADVANCED_FACE('',(#2116),#16625,.F.);
#17452=ADVANCED_FACE('',(#2117),#16626,.F.);
#17453=ADVANCED_FACE('',(#2118),#16627,.F.);
#17454=ADVANCED_FACE('',(#2119),#16628,.F.);
#17455=ADVANCED_FACE('',(#2120),#16629,.F.);
#17456=ADVANCED_FACE('',(#2121),#16630,.F.);
#17457=ADVANCED_FACE('',(#2122),#16631,.F.);
#17458=ADVANCED_FACE('',(#2123),#16632,.F.);
#17459=ADVANCED_FACE('',(#2124),#16633,.F.);
#17460=ADVANCED_FACE('',(#2125),#16634,.F.);
#17461=ADVANCED_FACE('',(#2126),#16635,.F.);
#17462=ADVANCED_FACE('',(#2127),#16636,.F.);
#17463=ADVANCED_FACE('',(#2128),#16637,.F.);
#17464=ADVANCED_FACE('',(#2129),#16638,.F.);
#17465=ADVANCED_FACE('',(#2130),#16639,.F.);
#17466=ADVANCED_FACE('',(#2131),#16640,.F.);
#17467=ADVANCED_FACE('',(#2132),#16641,.F.);
#17468=ADVANCED_FACE('',(#2133),#16642,.F.);
#17469=ADVANCED_FACE('',(#2134),#16643,.F.);
#17470=ADVANCED_FACE('',(#2135),#16644,.F.);
#17471=ADVANCED_FACE('',(#2136),#16645,.F.);
#17472=ADVANCED_FACE('',(#2137),#16646,.F.);
#17473=ADVANCED_FACE('',(#2138),#16647,.F.);
#17474=ADVANCED_FACE('',(#2139),#16648,.F.);
#17475=ADVANCED_FACE('',(#2140),#16649,.F.);
#17476=ADVANCED_FACE('',(#2141),#16650,.F.);
#17477=ADVANCED_FACE('',(#2142),#16651,.F.);
#17478=ADVANCED_FACE('',(#2143),#16652,.F.);
#17479=ADVANCED_FACE('',(#2144),#16653,.F.);
#17480=ADVANCED_FACE('',(#2145),#16654,.F.);
#17481=ADVANCED_FACE('',(#2146),#16655,.F.);
#17482=ADVANCED_FACE('',(#2147),#16656,.F.);
#17483=ADVANCED_FACE('',(#2148),#16657,.F.);
#17484=ADVANCED_FACE('',(#2149),#16658,.F.);
#17485=ADVANCED_FACE('',(#2150),#16659,.F.);
#17486=ADVANCED_FACE('',(#2151),#16660,.F.);
#17487=ADVANCED_FACE('',(#2152),#16661,.F.);
#17488=ADVANCED_FACE('',(#2153),#16662,.F.);
#17489=ADVANCED_FACE('',(#2154),#16663,.F.);
#17490=ADVANCED_FACE('',(#2155),#16664,.F.);
#17491=ADVANCED_FACE('',(#2156),#16665,.F.);
#17492=ADVANCED_FACE('',(#2157),#16666,.F.);
#17493=ADVANCED_FACE('',(#2158),#16667,.F.);
#17494=ADVANCED_FACE('',(#2159),#16668,.F.);
#17495=ADVANCED_FACE('',(#2160),#16669,.F.);
#17496=ADVANCED_FACE('',(#2161),#16670,.F.);
#17497=ADVANCED_FACE('',(#2162),#16671,.F.);
#17498=ADVANCED_FACE('',(#2163),#16672,.F.);
#17499=ADVANCED_FACE('',(#2164),#16673,.F.);
#17500=ADVANCED_FACE('',(#2165),#16674,.F.);
#17501=ADVANCED_FACE('',(#2166),#16675,.F.);
#17502=ADVANCED_FACE('',(#2167),#16676,.F.);
#17503=ADVANCED_FACE('',(#2168),#16677,.F.);
#17504=ADVANCED_FACE('',(#2169),#16678,.F.);
#17505=ADVANCED_FACE('',(#2170),#16679,.F.);
#17506=ADVANCED_FACE('',(#2171),#16680,.F.);
#17507=ADVANCED_FACE('',(#2172),#16681,.F.);
#17508=ADVANCED_FACE('',(#2173),#16682,.F.);
#17509=ADVANCED_FACE('',(#2174),#16683,.F.);
#17510=ADVANCED_FACE('',(#2175),#16684,.F.);
#17511=ADVANCED_FACE('',(#2176),#16685,.F.);
#17512=ADVANCED_FACE('',(#2177),#16686,.F.);
#17513=ADVANCED_FACE('',(#2178),#16687,.F.);
#17514=ADVANCED_FACE('',(#2179),#16688,.F.);
#17515=ADVANCED_FACE('',(#2180),#16689,.F.);
#17516=ADVANCED_FACE('',(#2181),#16690,.F.);
#17517=ADVANCED_FACE('',(#2182),#16691,.F.);
#17518=ADVANCED_FACE('',(#2183),#16692,.F.);
#17519=ADVANCED_FACE('',(#2184),#16693,.F.);
#17520=ADVANCED_FACE('',(#2185),#16694,.F.);
#17521=ADVANCED_FACE('',(#2186),#16695,.F.);
#17522=ADVANCED_FACE('',(#2187),#16696,.F.);
#17523=ADVANCED_FACE('',(#2188),#16697,.F.);
#17524=ADVANCED_FACE('',(#2189),#16698,.F.);
#17525=ADVANCED_FACE('',(#2190),#16699,.F.);
#17526=ADVANCED_FACE('',(#2191),#16700,.F.);
#17527=ADVANCED_FACE('',(#2192),#16701,.F.);
#17528=ADVANCED_FACE('',(#2193),#16702,.F.);
#17529=ADVANCED_FACE('',(#2194),#16703,.F.);
#17530=ADVANCED_FACE('',(#2195),#16704,.F.);
#17531=ADVANCED_FACE('',(#2196,#932,#933,#934,#935,#936),#16705,.T.);
#17532=ADVANCED_FACE('',(#2197,#937),#16706,.F.);
#17533=ADVANCED_FACE('',(#2198),#695,.T.);
#17534=ADVANCED_FACE('',(#2199,#938),#16707,.F.);
#17535=ADVANCED_FACE('',(#2200,#939),#16708,.T.);
#17536=ADVANCED_FACE('',(#2201),#696,.T.);
#17537=ADVANCED_FACE('',(#2202),#413,.F.);
#17538=ADVANCED_FACE('',(#2203),#697,.F.);
#17539=ADVANCED_FACE('',(#2204),#414,.F.);
#17540=ADVANCED_FACE('',(#2205),#16709,.T.);
#17541=ADVANCED_FACE('',(#2206),#16710,.T.);
#17542=ADVANCED_FACE('',(#2207),#698,.T.);
#17543=ADVANCED_FACE('',(#2208),#699,.T.);
#17544=ADVANCED_FACE('',(#2209),#185,.F.);
#17545=ADVANCED_FACE('',(#2210),#186,.F.);
#17546=ADVANCED_FACE('',(#2211),#187,.T.);
#17547=ADVANCED_FACE('',(#2212),#188,.T.);
#17548=ADVANCED_FACE('',(#2213),#700,.T.);
#17549=ADVANCED_FACE('',(#2214,#940),#16711,.F.);
#17550=ADVANCED_FACE('',(#2215,#941),#16712,.T.);
#17551=ADVANCED_FACE('',(#2216),#701,.F.);
#17799=CLOSED_SHELL('',(#17331,#17332,#17333,#17334,#17335,#17336,#17337,
#17338,#17339,#17340,#17341,#17342,#17343,#17344,#17345,#17346,#17347,#17348,
#17349,#17350,#17351,#17352,#17353,#17354,#17355,#17356,#17357,#17358,#17359,
#17360,#17361,#17362,#17363,#17364,#17365,#17366,#17367,#17368,#17369,#17370,
#17371,#17372,#17373,#17374,#17375,#17376,#17377,#17378,#17379,#17380,#17381,
#17382,#17383,#17384,#17385,#17386,#17387,#17388,#17389,#17390,#17391,#17392,
#17393,#17394,#17395,#17396,#17397,#17398,#17399,#17400,#17401,#17402,#17403,
#17404,#17405,#17406,#17407,#17408,#17409,#17410,#17411,#17412,#17413,#17414,
#17415,#17416,#17417,#17418,#17419,#17420,#17421,#17422,#17423,#17424,#17425,
#17426,#17427,#17428,#17429,#17430,#17431,#17432,#17433,#17434,#17435,#17436,
#17437,#17438,#17439,#17440,#17441,#17442,#17443,#17444,#17445,#17446,#17447,
#17448,#17449,#17450,#17451,#17452,#17453,#17454,#17455,#17456,#17457,#17458,
#17459,#17460,#17461,#17462,#17463,#17464,#17465,#17466,#17467,#17468,#17469,
#17470,#17471,#17472,#17473,#17474,#17475,#17476,#17477,#17478,#17479,#17480,
#17481,#17482,#17483,#17484,#17485,#17486,#17487,#17488,#17489,#17490,#17491,
#17492,#17493,#17494,#17495,#17496,#17497,#17498,#17499,#17500,#17501,#17502,
#17503,#17504,#17505,#17506,#17507,#17508,#17509,#17510,#17511,#17512,#17513,
#17514,#17515,#17516,#17517,#17518,#17519,#17520,#17521,#17522,#17523,#17524,
#17525,#17526,#17527,#17528,#17529,#17530,#17531,#17532,#17533,#17534,#17535,
#17536,#17537,#17538,#17539,#17540,#17541,#17542,#17543,#17544,#17545,#17546,
#17547,#17548,#17549,#17550,#17551));
#18787=AXIS2_PLACEMENT_3D('',#27554,#22045,#22046);
#18788=AXIS2_PLACEMENT_3D('',#27555,#22047,#22048);
#18789=AXIS2_PLACEMENT_3D('',#27562,#22051,#22052);
#18790=AXIS2_PLACEMENT_3D('',#27581,#22053,#22054);
#18791=AXIS2_PLACEMENT_3D('',#27657,#22056,#22057);
#18792=AXIS2_PLACEMENT_3D('',#27733,#22059,#22060);
#18793=AXIS2_PLACEMENT_3D('',#27811,#22062,#22063);
#18794=AXIS2_PLACEMENT_3D('',#27887,#22065,#22066);
#18795=AXIS2_PLACEMENT_3D('',#27963,#22068,#22069);
#18796=AXIS2_PLACEMENT_3D('',#28039,#22071,#22072);
#18797=AXIS2_PLACEMENT_3D('',#28115,#22074,#22075);
#18798=AXIS2_PLACEMENT_3D('',#28193,#22077,#22078);
#18799=AXIS2_PLACEMENT_3D('',#28269,#22080,#22081);
#18800=AXIS2_PLACEMENT_3D('',#28345,#22083,#22084);
#18801=AXIS2_PLACEMENT_3D('',#28423,#22086,#22087);
#18802=AXIS2_PLACEMENT_3D('',#28499,#22089,#22090);
#18803=AXIS2_PLACEMENT_3D('',#28575,#22092,#22093);
#18804=AXIS2_PLACEMENT_3D('',#28651,#22095,#22096);
#18805=AXIS2_PLACEMENT_3D('',#28729,#22098,#22099);
#18806=AXIS2_PLACEMENT_3D('',#28805,#22101,#22102);
#18807=AXIS2_PLACEMENT_3D('',#28881,#22104,#22105);
#18808=AXIS2_PLACEMENT_3D('',#28919,#22107,#22108);
#18809=AXIS2_PLACEMENT_3D('',#28954,#22109,#22110);
#18810=AXIS2_PLACEMENT_3D('',#28958,#22112,#22113);
#18811=AXIS2_PLACEMENT_3D('',#28960,#22114,#22115);
#18812=AXIS2_PLACEMENT_3D('',#28970,#22117,#22118);
#18813=AXIS2_PLACEMENT_3D('',#28991,#22121,#22122);
#18814=AXIS2_PLACEMENT_3D('',#29021,#22124,#22125);
#18815=AXIS2_PLACEMENT_3D('',#29051,#22127,#22128);
#18816=AXIS2_PLACEMENT_3D('',#29081,#22130,#22131);
#18817=AXIS2_PLACEMENT_3D('',#29111,#22133,#22134);
#18818=AXIS2_PLACEMENT_3D('',#29141,#22136,#22137);
#18819=AXIS2_PLACEMENT_3D('',#29171,#22139,#22140);
#18820=AXIS2_PLACEMENT_3D('',#29201,#22142,#22143);
#18821=AXIS2_PLACEMENT_3D('',#29231,#22145,#22146);
#18822=AXIS2_PLACEMENT_3D('',#29261,#22148,#22149);
#18823=AXIS2_PLACEMENT_3D('',#29291,#22151,#22152);
#18824=AXIS2_PLACEMENT_3D('',#29321,#22154,#22155);
#18825=AXIS2_PLACEMENT_3D('',#29351,#22157,#22158);
#18826=AXIS2_PLACEMENT_3D('',#29381,#22160,#22161);
#18827=AXIS2_PLACEMENT_3D('',#29411,#22163,#22164);
#18828=AXIS2_PLACEMENT_3D('',#29441,#22166,#22167);
#18829=AXIS2_PLACEMENT_3D('',#29471,#22169,#22170);
#18830=AXIS2_PLACEMENT_3D('',#29501,#22172,#22173);
#18831=AXIS2_PLACEMENT_3D('',#29531,#22175,#22176);
#18832=AXIS2_PLACEMENT_3D('',#29552,#22179,#22180);
#18833=AXIS2_PLACEMENT_3D('',#29590,#22182,#22183);
#18834=AXIS2_PLACEMENT_3D('',#29619,#22184,#22185);
#18835=AXIS2_PLACEMENT_3D('',#29695,#22187,#22188);
#18836=AXIS2_PLACEMENT_3D('',#29771,#22190,#22191);
#18837=AXIS2_PLACEMENT_3D('',#29796,#22194,#22195);
#18838=AXIS2_PLACEMENT_3D('',#29834,#22197,#22198);
#18839=AXIS2_PLACEMENT_3D('',#29872,#22200,#22201);
#18840=AXIS2_PLACEMENT_3D('',#29910,#22203,#22204);
#18841=AXIS2_PLACEMENT_3D('',#29948,#22206,#22207);
#18842=AXIS2_PLACEMENT_3D('',#29986,#22209,#22210);
#18843=AXIS2_PLACEMENT_3D('',#30024,#22212,#22213);
#18844=AXIS2_PLACEMENT_3D('',#30062,#22215,#22216);
#18845=AXIS2_PLACEMENT_3D('',#30078,#22218,#22219);
#18846=AXIS2_PLACEMENT_3D('',#30109,#22220,#22221);
#18847=AXIS2_PLACEMENT_3D('',#30187,#22223,#22224);
#18848=AXIS2_PLACEMENT_3D('',#30263,#22226,#22227);
#18849=AXIS2_PLACEMENT_3D('',#30322,#22230,#22231);
#18850=AXIS2_PLACEMENT_3D('',#30395,#22232,#22233);
#18851=AXIS2_PLACEMENT_3D('',#30398,#22234,#22235);
#18852=AXIS2_PLACEMENT_3D('',#30404,#22239,#22240);
#18853=AXIS2_PLACEMENT_3D('',#30412,#22243,#22244);
#18854=AXIS2_PLACEMENT_3D('',#30420,#22247,#22248);
#18855=AXIS2_PLACEMENT_3D('',#30428,#22251,#22252);
#18856=AXIS2_PLACEMENT_3D('',#30436,#22256,#22257);
#18857=AXIS2_PLACEMENT_3D('',#30437,#22258,#22259);
#18858=AXIS2_PLACEMENT_3D('',#30447,#22263,#22264);
#18859=AXIS2_PLACEMENT_3D('',#30453,#22266,#22267);
#18860=AXIS2_PLACEMENT_3D('',#30461,#22270,#22271);
#18861=AXIS2_PLACEMENT_3D('',#30469,#22275,#22276);
#18862=AXIS2_PLACEMENT_3D('',#30470,#22277,#22278);
#18863=AXIS2_PLACEMENT_3D('',#30480,#22282,#22283);
#18864=AXIS2_PLACEMENT_3D('',#30486,#22285,#22286);
#18865=AXIS2_PLACEMENT_3D('',#30494,#22289,#22290);
#18866=AXIS2_PLACEMENT_3D('',#30503,#22294,#22295);
#18867=AXIS2_PLACEMENT_3D('',#30504,#22296,#22297);
#18868=AXIS2_PLACEMENT_3D('',#30505,#22298,#22299);
#18869=AXIS2_PLACEMENT_3D('',#30515,#22303,#22304);
#18870=AXIS2_PLACEMENT_3D('',#30525,#22306,#22307);
#18871=AXIS2_PLACEMENT_3D('',#30533,#22310,#22311);
#18872=AXIS2_PLACEMENT_3D('',#30534,#22312,#22313);
#18873=AXIS2_PLACEMENT_3D('',#30535,#22314,#22315);
#18874=AXIS2_PLACEMENT_3D('',#30536,#22316,#22317);
#18875=AXIS2_PLACEMENT_3D('',#30537,#22318,#22319);
#18876=AXIS2_PLACEMENT_3D('',#30538,#22320,#22321);
#18877=AXIS2_PLACEMENT_3D('',#30540,#22322,#22323);
#18878=AXIS2_PLACEMENT_3D('',#30542,#22325,#22326);
#18879=AXIS2_PLACEMENT_3D('',#30543,#22327,#22328);
#18880=AXIS2_PLACEMENT_3D('',#30544,#22329,#22330);
#18881=AXIS2_PLACEMENT_3D('',#30545,#22331,#22332);
#18882=AXIS2_PLACEMENT_3D('',#30568,#22333,#22334);
#18883=AXIS2_PLACEMENT_3D('',#30570,#22335,#22336);
#18884=AXIS2_PLACEMENT_3D('',#30573,#22338,#22339);
#18885=AXIS2_PLACEMENT_3D('',#30574,#22340,#22341);
#18886=AXIS2_PLACEMENT_3D('',#30576,#22342,#22343);
#18887=AXIS2_PLACEMENT_3D('',#30577,#22344,#22345);
#18888=AXIS2_PLACEMENT_3D('',#30578,#22346,#22347);
#18889=AXIS2_PLACEMENT_3D('',#30579,#22348,#22349);
#18890=AXIS2_PLACEMENT_3D('',#30580,#22350,#22351);
#18891=AXIS2_PLACEMENT_3D('',#30582,#22353,#22354);
#18892=AXIS2_PLACEMENT_3D('',#30583,#22355,#22356);
#18893=AXIS2_PLACEMENT_3D('',#30584,#22357,#22358);
#18894=AXIS2_PLACEMENT_3D('',#30585,#22359,#22360);
#18895=AXIS2_PLACEMENT_3D('',#30586,#22361,#22362);
#18896=AXIS2_PLACEMENT_3D('',#30587,#22363,#22364);
#18897=AXIS2_PLACEMENT_3D('',#30588,#22365,#22366);
#18898=AXIS2_PLACEMENT_3D('',#30589,#22367,#22368);
#18899=AXIS2_PLACEMENT_3D('',#30590,#22369,#22370);
#18900=AXIS2_PLACEMENT_3D('',#30591,#22371,#22372);
#18901=AXIS2_PLACEMENT_3D('',#31194,#22377,#22378);
#18902=AXIS2_PLACEMENT_3D('',#31196,#22380,#22381);
#18903=AXIS2_PLACEMENT_3D('',#31198,#22382,#22383);
#18904=AXIS2_PLACEMENT_3D('',#31199,#22384,#22385);
#18905=AXIS2_PLACEMENT_3D('',#31201,#22386,#22387);
#18906=AXIS2_PLACEMENT_3D('',#31204,#22389,#22390);
#18907=AXIS2_PLACEMENT_3D('',#31205,#22391,#22392);
#18908=AXIS2_PLACEMENT_3D('',#31207,#22394,#22395);
#18909=AXIS2_PLACEMENT_3D('',#31208,#22396,#22397);
#18910=AXIS2_PLACEMENT_3D('',#31209,#22398,#22399);
#18911=AXIS2_PLACEMENT_3D('',#31210,#22400,#22401);
#18912=AXIS2_PLACEMENT_3D('',#31211,#22402,#22403);
#18913=AXIS2_PLACEMENT_3D('',#31212,#22404,#22405);
#18914=AXIS2_PLACEMENT_3D('',#31214,#22406,#22407);
#18915=AXIS2_PLACEMENT_3D('',#31216,#22408,#22409);
#18916=AXIS2_PLACEMENT_3D('',#31218,#22410,#22411);
#18917=AXIS2_PLACEMENT_3D('',#31219,#22412,#22413);
#18918=AXIS2_PLACEMENT_3D('',#31220,#22414,#22415);
#18919=AXIS2_PLACEMENT_3D('',#31222,#22416,#22417);
#18920=AXIS2_PLACEMENT_3D('',#31225,#22419,#22420);
#18921=AXIS2_PLACEMENT_3D('',#31226,#22421,#22422);
#18922=AXIS2_PLACEMENT_3D('',#31228,#22423,#22424);
#18923=AXIS2_PLACEMENT_3D('',#31231,#22426,#22427);
#18924=AXIS2_PLACEMENT_3D('',#31232,#22428,#22429);
#18925=AXIS2_PLACEMENT_3D('',#31233,#22430,#22431);
#18926=AXIS2_PLACEMENT_3D('',#31235,#22432,#22433);
#18927=AXIS2_PLACEMENT_3D('',#31236,#22434,#22435);
#18928=AXIS2_PLACEMENT_3D('',#31239,#22436,#22437);
#18929=AXIS2_PLACEMENT_3D('',#31241,#22438,#22439);
#18930=AXIS2_PLACEMENT_3D('',#31243,#22440,#22441);
#18931=AXIS2_PLACEMENT_3D('',#31245,#22442,#22443);
#18932=AXIS2_PLACEMENT_3D('',#31247,#22444,#22445);
#18933=AXIS2_PLACEMENT_3D('',#31250,#22447,#22448);
#18934=AXIS2_PLACEMENT_3D('',#31252,#22449,#22450);
#18935=AXIS2_PLACEMENT_3D('',#31254,#22451,#22452);
#18936=AXIS2_PLACEMENT_3D('',#31255,#22453,#22454);
#18937=AXIS2_PLACEMENT_3D('',#31256,#22455,#22456);
#18938=AXIS2_PLACEMENT_3D('',#31257,#22457,#22458);
#18939=AXIS2_PLACEMENT_3D('',#31258,#22459,#22460);
#18940=AXIS2_PLACEMENT_3D('',#31260,#22461,#22462);
#18941=AXIS2_PLACEMENT_3D('',#31261,#22463,#22464);
#18942=AXIS2_PLACEMENT_3D('',#31262,#22465,#22466);
#18943=AXIS2_PLACEMENT_3D('',#31263,#22467,#22468);
#18944=AXIS2_PLACEMENT_3D('',#31264,#22469,#22470);
#18945=AXIS2_PLACEMENT_3D('',#31265,#22471,#22472);
#18946=AXIS2_PLACEMENT_3D('',#31266,#22473,#22474);
#18947=AXIS2_PLACEMENT_3D('',#31267,#22475,#22476);
#18948=AXIS2_PLACEMENT_3D('',#31268,#22477,#22478);
#18949=AXIS2_PLACEMENT_3D('',#31270,#22479,#22480);
#18950=AXIS2_PLACEMENT_3D('',#31272,#22482,#22483);
#18951=AXIS2_PLACEMENT_3D('',#31273,#22484,#22485);
#18952=AXIS2_PLACEMENT_3D('',#31275,#22486,#22487);
#18953=AXIS2_PLACEMENT_3D('',#31278,#22489,#22490);
#18954=AXIS2_PLACEMENT_3D('',#31279,#22491,#22492);
#18955=AXIS2_PLACEMENT_3D('',#31280,#22493,#22494);
#18956=AXIS2_PLACEMENT_3D('',#31282,#22495,#22496);
#18957=AXIS2_PLACEMENT_3D('',#31285,#22498,#22499);
#18958=AXIS2_PLACEMENT_3D('',#31286,#22500,#22501);
#18959=AXIS2_PLACEMENT_3D('',#31287,#22502,#22503);
#18960=AXIS2_PLACEMENT_3D('',#31289,#22504,#22505);
#18961=AXIS2_PLACEMENT_3D('',#31292,#22507,#22508);
#18962=AXIS2_PLACEMENT_3D('',#31293,#22509,#22510);
#18963=AXIS2_PLACEMENT_3D('',#31294,#22511,#22512);
#18964=AXIS2_PLACEMENT_3D('',#31297,#22514,#22515);
#18965=AXIS2_PLACEMENT_3D('',#31298,#22516,#22517);
#18966=AXIS2_PLACEMENT_3D('',#31307,#22522,#22523);
#18967=AXIS2_PLACEMENT_3D('',#31313,#22527,#22528);
#18968=AXIS2_PLACEMENT_3D('',#31319,#22532,#22533);
#18969=AXIS2_PLACEMENT_3D('',#31325,#22537,#22538);
#18970=AXIS2_PLACEMENT_3D('',#31331,#22542,#22543);
#18971=AXIS2_PLACEMENT_3D('',#31337,#22547,#22548);
#18972=AXIS2_PLACEMENT_3D('',#31343,#22552,#22553);
#18973=AXIS2_PLACEMENT_3D('',#31349,#22557,#22558);
#18974=AXIS2_PLACEMENT_3D('',#31355,#22562,#22563);
#18975=AXIS2_PLACEMENT_3D('',#31361,#22567,#22568);
#18976=AXIS2_PLACEMENT_3D('',#31367,#22572,#22573);
#18977=AXIS2_PLACEMENT_3D('',#31373,#22577,#22578);
#18978=AXIS2_PLACEMENT_3D('',#31379,#22582,#22583);
#18979=AXIS2_PLACEMENT_3D('',#31385,#22587,#22588);
#18980=AXIS2_PLACEMENT_3D('',#31391,#22592,#22593);
#18981=AXIS2_PLACEMENT_3D('',#31397,#22597,#22598);
#18982=AXIS2_PLACEMENT_3D('',#31403,#22602,#22603);
#18983=AXIS2_PLACEMENT_3D('',#31409,#22607,#22608);
#18984=AXIS2_PLACEMENT_3D('',#31415,#22612,#22613);
#18985=AXIS2_PLACEMENT_3D('',#31421,#22617,#22618);
#18986=AXIS2_PLACEMENT_3D('',#31427,#22622,#22623);
#18987=AXIS2_PLACEMENT_3D('',#31433,#22627,#22628);
#18988=AXIS2_PLACEMENT_3D('',#31439,#22632,#22633);
#18989=AXIS2_PLACEMENT_3D('',#31445,#22637,#22638);
#18990=AXIS2_PLACEMENT_3D('',#31451,#22642,#22643);
#18991=AXIS2_PLACEMENT_3D('',#31457,#22647,#22648);
#18992=AXIS2_PLACEMENT_3D('',#31463,#22652,#22653);
#18993=AXIS2_PLACEMENT_3D('',#31469,#22657,#22658);
#18994=AXIS2_PLACEMENT_3D('',#31475,#22662,#22663);
#18995=AXIS2_PLACEMENT_3D('',#31481,#22667,#22668);
#18996=AXIS2_PLACEMENT_3D('',#31487,#22672,#22673);
#18997=AXIS2_PLACEMENT_3D('',#31493,#22677,#22678);
#18998=AXIS2_PLACEMENT_3D('',#31499,#22682,#22683);
#18999=AXIS2_PLACEMENT_3D('',#31505,#22687,#22688);
#19000=AXIS2_PLACEMENT_3D('',#31511,#22692,#22693);
#19001=AXIS2_PLACEMENT_3D('',#31517,#22697,#22698);
#19002=AXIS2_PLACEMENT_3D('',#31523,#22702,#22703);
#19003=AXIS2_PLACEMENT_3D('',#31529,#22707,#22708);
#19004=AXIS2_PLACEMENT_3D('',#31535,#22712,#22713);
#19005=AXIS2_PLACEMENT_3D('',#31541,#22717,#22718);
#19006=AXIS2_PLACEMENT_3D('',#31547,#22722,#22723);
#19007=AXIS2_PLACEMENT_3D('',#31553,#22727,#22728);
#19008=AXIS2_PLACEMENT_3D('',#31559,#22732,#22733);
#19009=AXIS2_PLACEMENT_3D('',#31565,#22737,#22738);
#19010=AXIS2_PLACEMENT_3D('',#31571,#22742,#22743);
#19011=AXIS2_PLACEMENT_3D('',#31577,#22747,#22748);
#19012=AXIS2_PLACEMENT_3D('',#31583,#22752,#22753);
#19013=AXIS2_PLACEMENT_3D('',#31589,#22757,#22758);
#19014=AXIS2_PLACEMENT_3D('',#31595,#22762,#22763);
#19015=AXIS2_PLACEMENT_3D('',#31601,#22767,#22768);
#19016=AXIS2_PLACEMENT_3D('',#31607,#22772,#22773);
#19017=AXIS2_PLACEMENT_3D('',#31613,#22777,#22778);
#19018=AXIS2_PLACEMENT_3D('',#31619,#22782,#22783);
#19019=AXIS2_PLACEMENT_3D('',#31625,#22787,#22788);
#19020=AXIS2_PLACEMENT_3D('',#31631,#22792,#22793);
#19021=AXIS2_PLACEMENT_3D('',#31637,#22797,#22798);
#19022=AXIS2_PLACEMENT_3D('',#31643,#22802,#22803);
#19023=AXIS2_PLACEMENT_3D('',#31649,#22807,#22808);
#19024=AXIS2_PLACEMENT_3D('',#31655,#22812,#22813);
#19025=AXIS2_PLACEMENT_3D('',#31661,#22817,#22818);
#19026=AXIS2_PLACEMENT_3D('',#31667,#22822,#22823);
#19027=AXIS2_PLACEMENT_3D('',#31673,#22827,#22828);
#19028=AXIS2_PLACEMENT_3D('',#31679,#22832,#22833);
#19029=AXIS2_PLACEMENT_3D('',#31685,#22837,#22838);
#19030=AXIS2_PLACEMENT_3D('',#31691,#22842,#22843);
#19031=AXIS2_PLACEMENT_3D('',#31697,#22847,#22848);
#19032=AXIS2_PLACEMENT_3D('',#31703,#22852,#22853);
#19033=AXIS2_PLACEMENT_3D('',#31709,#22857,#22858);
#19034=AXIS2_PLACEMENT_3D('',#31715,#22862,#22863);
#19035=AXIS2_PLACEMENT_3D('',#31721,#22867,#22868);
#19036=AXIS2_PLACEMENT_3D('',#31727,#22872,#22873);
#19037=AXIS2_PLACEMENT_3D('',#31733,#22877,#22878);
#19038=AXIS2_PLACEMENT_3D('',#31739,#22882,#22883);
#19039=AXIS2_PLACEMENT_3D('',#31745,#22887,#22888);
#19040=AXIS2_PLACEMENT_3D('',#31751,#22892,#22893);
#19041=AXIS2_PLACEMENT_3D('',#31757,#22897,#22898);
#19042=AXIS2_PLACEMENT_3D('',#31763,#22902,#22903);
#19043=AXIS2_PLACEMENT_3D('',#31769,#22907,#22908);
#19044=AXIS2_PLACEMENT_3D('',#31775,#22912,#22913);
#19045=AXIS2_PLACEMENT_3D('',#31781,#22917,#22918);
#19046=AXIS2_PLACEMENT_3D('',#31787,#22922,#22923);
#19047=AXIS2_PLACEMENT_3D('',#31793,#22927,#22928);
#19048=AXIS2_PLACEMENT_3D('',#31799,#22932,#22933);
#19049=AXIS2_PLACEMENT_3D('',#31805,#22937,#22938);
#19050=AXIS2_PLACEMENT_3D('',#31811,#22942,#22943);
#19051=AXIS2_PLACEMENT_3D('',#31817,#22947,#22948);
#19052=AXIS2_PLACEMENT_3D('',#31823,#22952,#22953);
#19053=AXIS2_PLACEMENT_3D('',#31829,#22957,#22958);
#19054=AXIS2_PLACEMENT_3D('',#31835,#22962,#22963);
#19055=AXIS2_PLACEMENT_3D('',#31838,#22966,#22967);
#19056=AXIS2_PLACEMENT_3D('',#31839,#22968,#22969);
#19057=AXIS2_PLACEMENT_3D('',#31840,#22970,#22971);
#19058=AXIS2_PLACEMENT_3D('',#31841,#22972,#22973);
#19059=AXIS2_PLACEMENT_3D('',#31843,#22974,#22975);
#19060=AXIS2_PLACEMENT_3D('',#31844,#22976,#22977);
#19061=AXIS2_PLACEMENT_3D('',#31846,#22978,#22979);
#19062=AXIS2_PLACEMENT_3D('',#31847,#22980,#22981);
#19063=AXIS2_PLACEMENT_3D('',#31850,#22982,#22983);
#19064=AXIS2_PLACEMENT_3D('',#31851,#22984,#22985);
#19065=AXIS2_PLACEMENT_3D('',#32397,#22989,#22990);
#19066=AXIS2_PLACEMENT_3D('',#32941,#22993,#22994);
#19067=AXIS2_PLACEMENT_3D('',#32942,#22995,#22996);
#19068=AXIS2_PLACEMENT_3D('',#32944,#22998,#22999);
#19069=AXIS2_PLACEMENT_3D('',#32945,#23000,#23001);
#19070=AXIS2_PLACEMENT_3D('',#32946,#23002,#23003);
#19071=AXIS2_PLACEMENT_3D('',#32947,#23004,#23005);
#19072=AXIS2_PLACEMENT_3D('',#32948,#23006,#23007);
#19073=AXIS2_PLACEMENT_3D('',#32951,#23009,#23010);
#19074=AXIS2_PLACEMENT_3D('',#32952,#23011,#23012);
#19075=AXIS2_PLACEMENT_3D('',#32955,#23014,#23015);
#19076=AXIS2_PLACEMENT_3D('',#32956,#23016,#23017);
#19077=AXIS2_PLACEMENT_3D('',#32959,#23019,#23020);
#19078=AXIS2_PLACEMENT_3D('',#32960,#23021,#23022);
#19079=AXIS2_PLACEMENT_3D('',#32962,#23023,#23024);
#19080=AXIS2_PLACEMENT_3D('',#32965,#23026,#23027);
#19081=AXIS2_PLACEMENT_3D('',#32966,#23028,#23029);
#19082=AXIS2_PLACEMENT_3D('',#32968,#23031,#23032);
#19083=AXIS2_PLACEMENT_3D('',#32969,#23033,#23034);
#19084=AXIS2_PLACEMENT_3D('',#32970,#23035,#23036);
#22045=DIRECTION('axis',(0.,0.,1.));
#22046=DIRECTION('refdir',(1.,0.,0.));
#22047=DIRECTION('center_axis',(7.09000435319733E-16,2.91501601757459E-15,
-1.));
#22048=DIRECTION('ref_axis',(0.236333478439908,0.971672005858198,3.E-15));
#22049=DIRECTION('',(7.09000435319733E-16,2.91501601757459E-15,-1.));
#22050=DIRECTION('',(-7.09000435319733E-16,-2.91501601757459E-15,1.));
#22051=DIRECTION('center_axis',(7.09000435319733E-16,2.91501601757459E-15,
-1.));
#22052=DIRECTION('ref_axis',(-0.236333478439908,-0.971672005858198,-3.E-15));
#22053=DIRECTION('center_axis',(7.09000435319733E-16,2.91501601757459E-15,
-1.));
#22054=DIRECTION('ref_axis',(0.236333478439908,0.971672005858198,3.E-15));
#22055=DIRECTION('',(7.09000435319733E-16,2.91501601757459E-15,-1.));
#22056=DIRECTION('center_axis',(7.09000435319733E-16,2.91501601757459E-15,
-1.));
#22057=DIRECTION('ref_axis',(0.236333478439908,0.971672005858198,3.E-15));
#22058=DIRECTION('',(7.09000435319733E-16,2.91501601757459E-15,-1.));
#22059=DIRECTION('center_axis',(7.09000435319733E-16,2.91501601757459E-15,
-1.));
#22060=DIRECTION('ref_axis',(0.236333478439908,0.971672005858198,3.E-15));
#22061=DIRECTION('',(7.09000435319733E-16,2.91501601757459E-15,-1.));
#22062=DIRECTION('center_axis',(7.09000435319733E-16,2.91501601757459E-15,
-1.));
#22063=DIRECTION('ref_axis',(0.236333478439908,0.971672005858198,3.E-15));
#22064=DIRECTION('',(7.09000435319733E-16,2.91501601757459E-15,-1.));
#22065=DIRECTION('center_axis',(7.09000435319733E-16,2.91501601757459E-15,
-1.));
#22066=DIRECTION('ref_axis',(0.236333478439908,0.971672005858198,3.E-15));
#22067=DIRECTION('',(7.09000435319733E-16,2.91501601757459E-15,-1.));
#22068=DIRECTION('center_axis',(7.09000435319733E-16,2.91501601757459E-15,
-1.));
#22069=DIRECTION('ref_axis',(0.236333478439908,0.971672005858198,3.E-15));
#22070=DIRECTION('',(7.09000435319733E-16,2.91501601757459E-15,-1.));
#22071=DIRECTION('center_axis',(7.09000435319733E-16,2.91501601757459E-15,
-1.));
#22072=DIRECTION('ref_axis',(0.236333478439908,0.971672005858198,3.E-15));
#22073=DIRECTION('',(7.09000435319733E-16,2.91501601757459E-15,-1.));
#22074=DIRECTION('center_axis',(7.09000435319733E-16,2.91501601757459E-15,
-1.));
#22075=DIRECTION('ref_axis',(0.236333478439908,0.971672005858198,3.E-15));
#22076=DIRECTION('',(7.09000435319733E-16,2.91501601757459E-15,-1.));
#22077=DIRECTION('center_axis',(7.09000435319733E-16,2.91501601757459E-15,
-1.));
#22078=DIRECTION('ref_axis',(0.236333478439908,0.971672005858198,3.E-15));
#22079=DIRECTION('',(7.09000435319733E-16,2.91501601757459E-15,-1.));
#22080=DIRECTION('center_axis',(7.09000435319733E-16,2.91501601757459E-15,
-1.));
#22081=DIRECTION('ref_axis',(0.236333478439908,0.971672005858198,3.E-15));
#22082=DIRECTION('',(7.09000435319733E-16,2.91501601757459E-15,-1.));
#22083=DIRECTION('center_axis',(7.09000435319733E-16,2.91501601757459E-15,
-1.));
#22084=DIRECTION('ref_axis',(0.236333478439908,0.971672005858198,3.E-15));
#22085=DIRECTION('',(7.09000435319733E-16,2.91501601757459E-15,-1.));
#22086=DIRECTION('center_axis',(7.09000435319733E-16,2.91501601757459E-15,
-1.));
#22087=DIRECTION('ref_axis',(0.236333478439908,0.971672005858198,3.E-15));
#22088=DIRECTION('',(7.09000435319733E-16,2.91501601757459E-15,-1.));
#22089=DIRECTION('center_axis',(7.09000435319733E-16,2.91501601757459E-15,
-1.));
#22090=DIRECTION('ref_axis',(0.236333478439908,0.971672005858198,3.E-15));
#22091=DIRECTION('',(7.09000435319733E-16,2.91501601757459E-15,-1.));
#22092=DIRECTION('center_axis',(7.09000435319733E-16,2.91501601757459E-15,
-1.));
#22093=DIRECTION('ref_axis',(0.236333478439908,0.971672005858198,3.E-15));
#22094=DIRECTION('',(7.09000435319733E-16,2.91501601757459E-15,-1.));
#22095=DIRECTION('center_axis',(7.09000435319733E-16,2.91501601757459E-15,
-1.));
#22096=DIRECTION('ref_axis',(0.236333478439908,0.971672005858198,3.E-15));
#22097=DIRECTION('',(7.09000435319733E-16,2.91501601757459E-15,-1.));
#22098=DIRECTION('center_axis',(7.09000435319733E-16,2.91501601757459E-15,
-1.));
#22099=DIRECTION('ref_axis',(0.236333478439908,0.971672005858198,3.E-15));
#22100=DIRECTION('',(7.09000435319733E-16,2.91501601757459E-15,-1.));
#22101=DIRECTION('center_axis',(7.09000435319733E-16,2.91501601757459E-15,
-1.));
#22102=DIRECTION('ref_axis',(0.236333478439908,0.971672005858198,3.E-15));
#22103=DIRECTION('',(7.09000435319733E-16,2.91501601757459E-15,-1.));
#22104=DIRECTION('center_axis',(7.09000435319733E-16,2.91501601757459E-15,
-1.));
#22105=DIRECTION('ref_axis',(0.236333478439908,0.971672005858198,3.E-15));
#22106=DIRECTION('',(7.09000435319733E-16,2.91501601757459E-15,-1.));
#22107=DIRECTION('center_axis',(-7.09000435319733E-16,-2.91501601757459E-15,
1.));
#22108=DIRECTION('ref_axis',(-0.236333478439908,-0.971672005858198,-3.E-15));
#22109=DIRECTION('center_axis',(-9.36335395655066E-14,2.27738783980021E-14,
1.));
#22110=DIRECTION('ref_axis',(-0.236333478439913,-0.971672005858196,0.));
#22111=DIRECTION('',(-9.36335395655066E-14,2.27738783980021E-14,1.));
#22112=DIRECTION('center_axis',(-7.09000435319733E-16,-2.91501601757459E-15,
1.));
#22113=DIRECTION('ref_axis',(-0.236333478439908,-0.971672005858198,-3.E-15));
#22114=DIRECTION('center_axis',(-0.0526028585739488,0.0502161354828127,
0.997352133906085));
#22115=DIRECTION('ref_axis',(0.721410631826286,-0.688678429526452,0.0727235930972822));
#22116=DIRECTION('',(7.09000435319733E-16,2.91501601757459E-15,-1.));
#22117=DIRECTION('center_axis',(0.,0.,1.));
#22118=DIRECTION('ref_axis',(-0.236333478439877,-0.971672005858205,0.));
#22119=DIRECTION('',(0.,0.,1.));
#22120=DIRECTION('',(-7.09000435319733E-16,-2.91501601757459E-15,1.));
#22121=DIRECTION('center_axis',(0.,0.,1.));
#22122=DIRECTION('ref_axis',(-0.236333478439877,-0.971672005858205,0.));
#22123=DIRECTION('',(0.,0.,1.));
#22124=DIRECTION('center_axis',(0.,0.,1.));
#22125=DIRECTION('ref_axis',(-0.236333478439877,-0.971672005858205,0.));
#22126=DIRECTION('',(0.,0.,1.));
#22127=DIRECTION('center_axis',(0.,0.,1.));
#22128=DIRECTION('ref_axis',(-0.236333478439877,-0.971672005858205,0.));
#22129=DIRECTION('',(0.,0.,1.));
#22130=DIRECTION('center_axis',(0.,0.,1.));
#22131=DIRECTION('ref_axis',(-0.236333478439877,-0.971672005858205,0.));
#22132=DIRECTION('',(0.,0.,1.));
#22133=DIRECTION('center_axis',(0.,0.,1.));
#22134=DIRECTION('ref_axis',(-0.236333478439877,-0.971672005858205,0.));
#22135=DIRECTION('',(0.,0.,1.));
#22136=DIRECTION('center_axis',(0.,0.,1.));
#22137=DIRECTION('ref_axis',(-0.236333478439877,-0.971672005858205,0.));
#22138=DIRECTION('',(0.,0.,1.));
#22139=DIRECTION('center_axis',(0.,0.,1.));
#22140=DIRECTION('ref_axis',(-0.236333478439877,-0.971672005858205,0.));
#22141=DIRECTION('',(0.,0.,1.));
#22142=DIRECTION('center_axis',(0.,0.,1.));
#22143=DIRECTION('ref_axis',(-0.236333478439877,-0.971672005858205,0.));
#22144=DIRECTION('',(0.,0.,1.));
#22145=DIRECTION('center_axis',(0.,0.,1.));
#22146=DIRECTION('ref_axis',(-0.236333478439877,-0.971672005858205,0.));
#22147=DIRECTION('',(0.,0.,1.));
#22148=DIRECTION('center_axis',(0.,0.,1.));
#22149=DIRECTION('ref_axis',(-0.236333478439877,-0.971672005858205,0.));
#22150=DIRECTION('',(0.,0.,1.));
#22151=DIRECTION('center_axis',(0.,0.,1.));
#22152=DIRECTION('ref_axis',(-0.236333478439877,-0.971672005858205,0.));
#22153=DIRECTION('',(0.,0.,1.));
#22154=DIRECTION('center_axis',(0.,0.,1.));
#22155=DIRECTION('ref_axis',(-0.236333478439877,-0.971672005858205,0.));
#22156=DIRECTION('',(0.,0.,1.));
#22157=DIRECTION('center_axis',(0.,0.,1.));
#22158=DIRECTION('ref_axis',(-0.236333478439877,-0.971672005858205,0.));
#22159=DIRECTION('',(0.,0.,1.));
#22160=DIRECTION('center_axis',(0.,0.,1.));
#22161=DIRECTION('ref_axis',(-0.236333478439877,-0.971672005858205,0.));
#22162=DIRECTION('',(0.,0.,1.));
#22163=DIRECTION('center_axis',(0.,0.,1.));
#22164=DIRECTION('ref_axis',(-0.236333478439877,-0.971672005858205,0.));
#22165=DIRECTION('',(0.,0.,1.));
#22166=DIRECTION('center_axis',(0.,0.,1.));
#22167=DIRECTION('ref_axis',(-0.236333478439877,-0.971672005858205,0.));
#22168=DIRECTION('',(0.,0.,1.));
#22169=DIRECTION('center_axis',(0.,0.,1.));
#22170=DIRECTION('ref_axis',(-0.236333478439877,-0.971672005858205,0.));
#22171=DIRECTION('',(0.,0.,1.));
#22172=DIRECTION('center_axis',(0.,0.,1.));
#22173=DIRECTION('ref_axis',(-0.236333478439877,-0.971672005858205,0.));
#22174=DIRECTION('',(0.,0.,1.));
#22175=DIRECTION('center_axis',(0.,0.,1.));
#22176=DIRECTION('ref_axis',(-0.236333478439877,-0.971672005858205,0.));
#22177=DIRECTION('',(0.,0.,1.));
#22178=DIRECTION('',(7.09000435319733E-16,2.91501601757459E-15,-1.));
#22179=DIRECTION('center_axis',(-7.09000435319733E-16,-2.91501601757459E-15,
1.));
#22180=DIRECTION('ref_axis',(-0.236333478439911,-0.971672005858197,-3.E-15));
#22181=DIRECTION('',(7.09000435319733E-16,2.91501601757459E-15,-1.));
#22182=DIRECTION('center_axis',(0.,0.,1.));
#22183=DIRECTION('ref_axis',(1.,0.,0.));
#22184=DIRECTION('center_axis',(-7.09000435319733E-16,-2.91501601757459E-15,
1.));
#22185=DIRECTION('ref_axis',(-0.236333478439911,-0.971672005858197,-3.E-15));
#22186=DIRECTION('',(7.09000435319733E-16,2.91501601757459E-15,-1.));
#22187=DIRECTION('center_axis',(-7.09000435319733E-16,-2.91501601757459E-15,
1.));
#22188=DIRECTION('ref_axis',(-0.236333478439911,-0.971672005858197,-3.E-15));
#22189=DIRECTION('',(7.09000435319733E-16,2.91501601757459E-15,-1.));
#22190=DIRECTION('center_axis',(0.,0.,-1.));
#22191=DIRECTION('ref_axis',(-0.236333478439914,-0.971672005858196,0.));
#22192=DIRECTION('',(0.,0.,1.));
#22193=DIRECTION('',(-7.09000435319733E-16,-2.91501601757459E-15,1.));
#22194=DIRECTION('center_axis',(0.,0.,-1.));
#22195=DIRECTION('ref_axis',(-0.236333478439914,-0.971672005858196,0.));
#22196=DIRECTION('',(0.,0.,1.));
#22197=DIRECTION('center_axis',(0.,0.,-1.));
#22198=DIRECTION('ref_axis',(-0.236333478439914,-0.971672005858196,0.));
#22199=DIRECTION('',(0.,0.,1.));
#22200=DIRECTION('center_axis',(0.,0.,-1.));
#22201=DIRECTION('ref_axis',(-0.236333478439914,-0.971672005858196,0.));
#22202=DIRECTION('',(0.,0.,1.));
#22203=DIRECTION('center_axis',(0.,0.,-1.));
#22204=DIRECTION('ref_axis',(-0.236333478439914,-0.971672005858196,0.));
#22205=DIRECTION('',(0.,0.,1.));
#22206=DIRECTION('center_axis',(0.,0.,-1.));
#22207=DIRECTION('ref_axis',(-0.236333478439914,-0.971672005858196,0.));
#22208=DIRECTION('',(0.,0.,1.));
#22209=DIRECTION('center_axis',(0.,0.,-1.));
#22210=DIRECTION('ref_axis',(-0.236333478439914,-0.971672005858196,0.));
#22211=DIRECTION('',(0.,0.,1.));
#22212=DIRECTION('center_axis',(0.,0.,-1.));
#22213=DIRECTION('ref_axis',(-0.236333478439914,-0.971672005858196,0.));
#22214=DIRECTION('',(0.,0.,1.));
#22215=DIRECTION('center_axis',(0.,0.,1.));
#22216=DIRECTION('ref_axis',(0.851485939575788,-0.524377435350471,0.));
#22217=DIRECTION('',(0.,0.,1.));
#22218=DIRECTION('center_axis',(0.,0.,1.));
#22219=DIRECTION('ref_axis',(0.851485939575788,-0.524377435350471,0.));
#22220=DIRECTION('center_axis',(0.,0.,1.));
#22221=DIRECTION('ref_axis',(0.851485939575788,-0.524377435350471,0.));
#22222=DIRECTION('',(0.,0.,1.));
#22223=DIRECTION('center_axis',(0.,0.,1.));
#22224=DIRECTION('ref_axis',(0.851485939575788,-0.524377435350471,0.));
#22225=DIRECTION('',(0.,0.,1.));
#22226=DIRECTION('center_axis',(0.,0.,1.));
#22227=DIRECTION('ref_axis',(0.851485939575788,-0.524377435350471,0.));
#22228=DIRECTION('',(0.,0.,1.));
#22229=DIRECTION('',(0.,0.,-1.));
#22230=DIRECTION('center_axis',(0.,0.,1.));
#22231=DIRECTION('ref_axis',(0.851485939575788,-0.524377435350471,0.));
#22232=DIRECTION('center_axis',(0.,0.,1.));
#22233=DIRECTION('ref_axis',(0.851485939575788,-0.524377435350472,0.));
#22234=DIRECTION('center_axis',(0.,0.,-1.));
#22235=DIRECTION('ref_axis',(0.85148593957579,-0.524377435350467,0.));
#22236=DIRECTION('',(0.524377435350472,0.851485939575788,0.));
#22237=DIRECTION('',(0.851485939575788,-0.524377435350471,0.));
#22238=DIRECTION('',(-0.524377435350472,-0.851485939575788,0.));
#22239=DIRECTION('center_axis',(-0.524377435350472,-0.851485939575788,0.));
#22240=DIRECTION('ref_axis',(-0.851485939575788,0.524377435350472,0.));
#22241=DIRECTION('',(0.,0.,1.));
#22242=DIRECTION('',(0.,0.,1.));
#22243=DIRECTION('center_axis',(0.851485939575788,-0.524377435350471,0.));
#22244=DIRECTION('ref_axis',(-0.524377435350472,-0.851485939575788,0.));
#22245=DIRECTION('',(0.524377435350472,0.851485939575788,0.));
#22246=DIRECTION('',(0.,0.,-1.));
#22247=DIRECTION('center_axis',(-0.851485939575788,0.524377435350471,0.));
#22248=DIRECTION('ref_axis',(-0.524377435350472,-0.851485939575788,0.));
#22249=DIRECTION('',(0.,0.,1.));
#22250=DIRECTION('',(-0.524377435350472,-0.851485939575788,0.));
#22251=DIRECTION('center_axis',(0.,0.,-1.));
#22252=DIRECTION('ref_axis',(0.524377435350472,0.851485939575788,0.));
#22253=DIRECTION('',(0.851485939575786,-0.524377435350475,0.));
#22254=DIRECTION('',(-0.524377435350475,-0.851485939575786,0.));
#22255=DIRECTION('',(-0.851485939575786,0.524377435350475,0.));
#22256=DIRECTION('center_axis',(0.,0.,1.));
#22257=DIRECTION('ref_axis',(-0.851485939575788,0.524377435350472,0.));
#22258=DIRECTION('center_axis',(0.524377435350475,0.851485939575786,0.));
#22259=DIRECTION('ref_axis',(-0.851485939575786,0.524377435350475,0.));
#22260=DIRECTION('',(0.,0.,1.));
#22261=DIRECTION('',(-0.851485939575786,0.524377435350475,0.));
#22262=DIRECTION('',(0.,0.,1.));
#22263=DIRECTION('center_axis',(-0.851485939575786,0.524377435350475,0.));
#22264=DIRECTION('ref_axis',(0.,0.,1.));
#22265=DIRECTION('',(0.,0.,1.));
#22266=DIRECTION('center_axis',(-0.524377435350475,-0.851485939575786,0.));
#22267=DIRECTION('ref_axis',(-0.851485939575786,0.524377435350475,0.));
#22268=DIRECTION('',(0.851485939575786,-0.524377435350475,0.));
#22269=DIRECTION('',(0.,0.,-1.));
#22270=DIRECTION('center_axis',(0.,0.,-1.));
#22271=DIRECTION('ref_axis',(0.524377435350472,0.851485939575788,0.));
#22272=DIRECTION('',(-0.524377435350471,-0.851485939575788,0.));
#22273=DIRECTION('',(-0.851485939575788,0.524377435350472,0.));
#22274=DIRECTION('',(0.524377435350472,0.851485939575788,0.));
#22275=DIRECTION('center_axis',(0.,0.,1.));
#22276=DIRECTION('ref_axis',(-0.851485939575788,0.524377435350472,0.));
#22277=DIRECTION('center_axis',(0.851485939575788,-0.524377435350471,0.));
#22278=DIRECTION('ref_axis',(-0.524377435350472,-0.851485939575788,0.));
#22279=DIRECTION('',(0.,0.,1.));
#22280=DIRECTION('',(0.524377435350472,0.851485939575788,0.));
#22281=DIRECTION('',(0.,0.,1.));
#22282=DIRECTION('center_axis',(0.524377435350472,0.851485939575788,0.));
#22283=DIRECTION('ref_axis',(0.,0.,-1.));
#22284=DIRECTION('',(0.,0.,1.));
#22285=DIRECTION('center_axis',(-0.851485939575788,0.524377435350471,0.));
#22286=DIRECTION('ref_axis',(-0.524377435350471,-0.851485939575788,0.));
#22287=DIRECTION('',(-0.524377435350471,-0.851485939575788,0.));
#22288=DIRECTION('',(0.,0.,-1.));
#22289=DIRECTION('center_axis',(0.,0.,-1.));
#22290=DIRECTION('ref_axis',(0.524377435350472,0.851485939575788,0.));
#22291=DIRECTION('',(-0.851485939575788,0.524377435350471,0.));
#22292=DIRECTION('',(0.524377435350472,0.851485939575788,0.));
#22293=DIRECTION('',(0.851485939575788,-0.524377435350471,0.));
#22294=DIRECTION('center_axis',(0.,0.,1.));
#22295=DIRECTION('ref_axis',(-0.851485939575788,0.524377435350472,0.));
#22296=DIRECTION('center_axis',(0.,0.,1.));
#22297=DIRECTION('ref_axis',(-0.851485939575788,0.524377435350472,0.));
#22298=DIRECTION('center_axis',(-0.524377435350471,-0.851485939575788,0.));
#22299=DIRECTION('ref_axis',(0.,0.,1.));
#22300=DIRECTION('',(0.,0.,1.));
#22301=DIRECTION('',(0.851485939575788,-0.524377435350471,0.));
#22302=DIRECTION('',(0.,0.,1.));
#22303=DIRECTION('center_axis',(0.851485939575788,-0.524377435350472,0.));
#22304=DIRECTION('ref_axis',(0.,0.,-1.));
#22305=DIRECTION('',(0.,0.,1.));
#22306=DIRECTION('center_axis',(0.524377435350471,0.851485939575788,0.));
#22307=DIRECTION('ref_axis',(-0.851485939575788,0.524377435350471,0.));
#22308=DIRECTION('',(-0.851485939575788,0.524377435350471,0.));
#22309=DIRECTION('',(0.,0.,-1.));
#22310=DIRECTION('center_axis',(0.,0.,1.));
#22311=DIRECTION('ref_axis',(0.851485939575788,-0.524377435350471,0.));
#22312=DIRECTION('center_axis',(0.,0.,1.));
#22313=DIRECTION('ref_axis',(0.851485939575788,-0.524377435350471,0.));
#22314=DIRECTION('center_axis',(0.,0.,1.));
#22315=DIRECTION('ref_axis',(0.851485939575788,-0.524377435350471,0.));
#22316=DIRECTION('center_axis',(0.,0.,1.));
#22317=DIRECTION('ref_axis',(0.851485939575788,-0.524377435350472,0.));
#22318=DIRECTION('center_axis',(0.,0.,1.));
#22319=DIRECTION('ref_axis',(0.851485939575788,-0.524377435350472,0.));
#22320=DIRECTION('center_axis',(0.,0.,1.));
#22321=DIRECTION('ref_axis',(0.851485939575788,-0.524377435350472,0.));
#22322=DIRECTION('center_axis',(0.,0.,1.));
#22323=DIRECTION('ref_axis',(0.851485939575788,-0.524377435350472,0.));
#22324=DIRECTION('',(0.,0.,-1.));
#22325=DIRECTION('center_axis',(0.,0.,1.));
#22326=DIRECTION('ref_axis',(0.851485939575788,-0.524377435350472,0.));
#22327=DIRECTION('center_axis',(0.,0.,1.));
#22328=DIRECTION('ref_axis',(0.851485939575788,-0.524377435350472,0.));
#22329=DIRECTION('center_axis',(0.,0.,1.));
#22330=DIRECTION('ref_axis',(0.851485939575788,-0.524377435350472,0.));
#22331=DIRECTION('center_axis',(0.,0.,1.));
#22332=DIRECTION('ref_axis',(0.851485939575788,-0.524377435350472,0.));
#22333=DIRECTION('center_axis',(0.,0.,1.));
#22334=DIRECTION('ref_axis',(0.851485939575788,-0.524377435350471,0.));
#22335=DIRECTION('center_axis',(0.,0.,1.));
#22336=DIRECTION('ref_axis',(0.851485939575788,-0.524377435350471,0.));
#22337=DIRECTION('',(0.,0.,1.));
#22338=DIRECTION('center_axis',(-7.09000435319733E-16,-2.91501601757459E-15,
1.));
#22339=DIRECTION('ref_axis',(3.62723386184346E-31,1.,2.91501601757459E-15));
#22340=DIRECTION('center_axis',(0.,0.,1.));
#22341=DIRECTION('ref_axis',(0.851485939575787,-0.524377435350472,0.));
#22342=DIRECTION('center_axis',(0.,0.,1.));
#22343=DIRECTION('ref_axis',(0.851485939575787,-0.524377435350472,0.));
#22344=DIRECTION('center_axis',(-0.524377435350472,-0.851485939575788,0.));
#22345=DIRECTION('ref_axis',(-0.851485939575788,0.524377435350472,0.));
#22346=DIRECTION('center_axis',(0.,0.,1.));
#22347=DIRECTION('ref_axis',(0.851485939575788,-0.524377435350471,0.));
#22348=DIRECTION('center_axis',(0.,0.,1.));
#22349=DIRECTION('ref_axis',(0.851485939575788,-0.524377435350471,0.));
#22350=DIRECTION('center_axis',(0.,0.,1.));
#22351=DIRECTION('ref_axis',(0.851485939575788,-0.524377435350471,0.));
#22352=DIRECTION('',(0.671291577386942,-0.413406891836534,-0.615192945271162));
#22353=DIRECTION('center_axis',(0.,0.,1.));
#22354=DIRECTION('ref_axis',(0.851485939575788,-0.524377435350471,0.));
#22355=DIRECTION('center_axis',(0.,0.,1.));
#22356=DIRECTION('ref_axis',(0.851485939575788,-0.524377435350471,0.));
#22357=DIRECTION('center_axis',(0.,0.,1.));
#22358=DIRECTION('ref_axis',(0.851485939575788,-0.524377435350471,0.));
#22359=DIRECTION('center_axis',(0.,0.,1.));
#22360=DIRECTION('ref_axis',(0.851485939575788,-0.524377435350471,0.));
#22361=DIRECTION('center_axis',(0.,0.,1.));
#22362=DIRECTION('ref_axis',(0.851485939575788,-0.524377435350471,0.));
#22363=DIRECTION('center_axis',(0.,0.,1.));
#22364=DIRECTION('ref_axis',(0.851485939575788,-0.524377435350471,0.));
#22365=DIRECTION('center_axis',(0.,0.,1.));
#22366=DIRECTION('ref_axis',(0.851485939575788,-0.524377435350471,0.));
#22367=DIRECTION('center_axis',(0.,0.,1.));
#22368=DIRECTION('ref_axis',(0.851485939575788,-0.524377435350472,0.));
#22369=DIRECTION('center_axis',(0.,0.,1.));
#22370=DIRECTION('ref_axis',(0.851485939575788,-0.524377435350472,0.));
#22371=DIRECTION('center_axis',(0.,0.,1.));
#22372=DIRECTION('ref_axis',(0.851485939575788,-0.524377435350472,0.));
#22373=DIRECTION('',(0.204670796093705,0.841492641219382,-0.499999999999997));
#22374=DIRECTION('',(-0.204670796093705,-0.841492641219382,0.499999999999997));
#22375=DIRECTION('',(0.204670796093705,0.841492641219379,0.500000000000002));
#22376=DIRECTION('',(-0.204670796093705,-0.841492641219379,-0.500000000000002));
#22377=DIRECTION('center_axis',(-0.971672005858197,0.236333478439911,0.));
#22378=DIRECTION('ref_axis',(7.09000435319733E-16,2.91501601757459E-15,
-1.));
#22379=DIRECTION('',(7.09000435319733E-16,2.91501601757459E-15,-1.));
#22380=DIRECTION('center_axis',(7.09000435319733E-16,2.91501601757459E-15,
-1.));
#22381=DIRECTION('ref_axis',(-0.971672005858197,0.236333478439911,-1.18897715061811E-32));
#22382=DIRECTION('center_axis',(-7.09000435319733E-16,-2.91501601757459E-15,
1.));
#22383=DIRECTION('ref_axis',(0.23633347843991,0.971672005858197,3.E-15));
#22384=DIRECTION('center_axis',(7.09000435319733E-16,2.91501601757459E-15,
-1.));
#22385=DIRECTION('ref_axis',(0.236333478439911,0.971672005858197,3.E-15));
#22386=DIRECTION('center_axis',(0.,0.,-1.));
#22387=DIRECTION('ref_axis',(1.,0.,0.));
#22388=DIRECTION('',(7.09000435319733E-16,2.91501601757459E-15,-1.));
#22389=DIRECTION('center_axis',(7.09000435319733E-16,2.91501601757459E-15,
-1.));
#22390=DIRECTION('ref_axis',(0.236333478439911,0.971672005858197,3.E-15));
#22391=DIRECTION('center_axis',(-7.09000435319733E-16,-2.91501601757459E-15,
1.));
#22392=DIRECTION('ref_axis',(-0.153499123700145,0.988148783849521,2.7716385871436E-15));
#22393=DIRECTION('',(7.09000435319733E-16,2.91501601757459E-15,-1.));
#22394=DIRECTION('center_axis',(7.09000435319733E-16,2.91501601757459E-15,
-1.));
#22395=DIRECTION('ref_axis',(0.236333478439911,0.971672005858197,3.E-15));
#22396=DIRECTION('center_axis',(0.,0.,-1.));
#22397=DIRECTION('ref_axis',(-0.236333478439914,-0.971672005858196,0.));
#22398=DIRECTION('center_axis',(0.971672005858197,-0.236333478439911,0.));
#22399=DIRECTION('ref_axis',(-0.236333478439911,-0.971672005858197,-3.E-15));
#22400=DIRECTION('center_axis',(7.09000435319733E-16,2.91501601757459E-15,
-1.));
#22401=DIRECTION('ref_axis',(0.236333478439912,0.971672005858197,4.30631961066728E-15));
#22402=DIRECTION('center_axis',(-0.971672005858197,0.236333478439911,2.95822839457879E-31));
#22403=DIRECTION('ref_axis',(-0.236333478439911,-0.971672005858197,-5.38289951333409E-15));
#22404=DIRECTION('center_axis',(7.09000435319733E-16,2.91501601757459E-15,
-1.));
#22405=DIRECTION('ref_axis',(0.236333478439911,0.971672005858197,2.8421709430404E-15));
#22406=DIRECTION('center_axis',(7.09000435319733E-16,2.91501601757459E-15,
-1.));
#22407=DIRECTION('ref_axis',(0.236333478439912,0.971672005858197,3.E-15));
#22408=DIRECTION('center_axis',(-0.971672005858197,0.236333478439911,-4.93038065763132E-31));
#22409=DIRECTION('ref_axis',(-0.236333478439911,-0.971672005858197,-3.5527136788005E-15));
#22410=DIRECTION('center_axis',(-7.09000435319733E-16,-2.91501601757459E-15,
1.));
#22411=DIRECTION('ref_axis',(0.236333478439911,0.971672005858197,3.E-15));
#22412=DIRECTION('center_axis',(-7.09000435319733E-16,-2.91501601757459E-15,
1.));
#22413=DIRECTION('ref_axis',(0.236333478439911,0.971672005858197,3.E-15));
#22414=DIRECTION('center_axis',(7.09000435319733E-16,2.91501601757459E-15,
-1.));
#22415=DIRECTION('ref_axis',(0.236333478439911,0.971672005858197,3.E-15));
#22416=DIRECTION('center_axis',(-7.09000435319733E-16,-2.91501601757459E-15,
1.));
#22417=DIRECTION('ref_axis',(-0.236333478439911,-0.971672005858197,-3.E-15));
#22418=DIRECTION('',(7.09000435319733E-16,2.91501601757459E-15,-1.));
#22419=DIRECTION('center_axis',(-7.09000435319733E-16,-2.91501601757459E-15,
1.));
#22420=DIRECTION('ref_axis',(-0.236333478439911,-0.971672005858197,-3.E-15));
#22421=DIRECTION('center_axis',(7.09000435319733E-16,2.91501601757459E-15,
-1.));
#22422=DIRECTION('ref_axis',(0.236333478439912,0.971672005858197,3.E-15));
#22423=DIRECTION('center_axis',(-7.09000435319733E-16,-2.91501601757459E-15,
1.));
#22424=DIRECTION('ref_axis',(-0.236333478439912,-0.971672005858197,-3.E-15));
#22425=DIRECTION('',(-7.09000435319733E-16,-2.91501601757459E-15,1.));
#22426=DIRECTION('center_axis',(-7.09000435319733E-16,-2.91501601757459E-15,
1.));
#22427=DIRECTION('ref_axis',(-0.236333478439912,-0.971672005858197,-3.E-15));
#22428=DIRECTION('center_axis',(-7.09000435319733E-16,-2.91501601757459E-15,
1.));
#22429=DIRECTION('ref_axis',(-0.236333478439911,-0.971672005858197,-3.E-15));
#22430=DIRECTION('center_axis',(-7.09000435319733E-16,-2.91501601757459E-15,
1.));
#22431=DIRECTION('ref_axis',(-0.236333478439911,-0.971672005858197,-3.E-15));
#22432=DIRECTION('center_axis',(-7.09000435319733E-16,-2.91501601757459E-15,
1.));
#22433=DIRECTION('ref_axis',(-0.236333478439911,-0.971672005858197,-3.E-15));
#22434=DIRECTION('center_axis',(-7.09000435319733E-16,-2.91501601757459E-15,
1.));
#22435=DIRECTION('ref_axis',(-0.236333478439911,-0.971672005858197,-3.E-15));
#22436=DIRECTION('center_axis',(7.09000435319733E-16,2.91501601757459E-15,
-1.));
#22437=DIRECTION('ref_axis',(0.236333478439911,0.971672005858197,3.E-15));
#22438=DIRECTION('center_axis',(7.09000435319733E-16,2.91501601757459E-15,
-1.));
#22439=DIRECTION('ref_axis',(0.236333478439911,0.971672005858197,3.E-15));
#22440=DIRECTION('center_axis',(7.09000435319733E-16,2.91501601757459E-15,
-1.));
#22441=DIRECTION('ref_axis',(0.236333478439911,0.971672005858197,3.E-15));
#22442=DIRECTION('center_axis',(7.09000435319733E-16,2.91501601757459E-15,
-1.));
#22443=DIRECTION('ref_axis',(0.236333478439911,0.971672005858197,3.E-15));
#22444=DIRECTION('center_axis',(7.09000435319733E-16,2.91501601757459E-15,
-1.));
#22445=DIRECTION('ref_axis',(0.236333478439911,0.971672005858197,3.E-15));
#22446=DIRECTION('',(7.09000435319733E-16,2.91501601757459E-15,-1.));
#22447=DIRECTION('center_axis',(7.09000435319733E-16,2.91501601757459E-15,
-1.));
#22448=DIRECTION('ref_axis',(0.236333478439911,0.971672005858197,3.E-15));
#22449=DIRECTION('center_axis',(7.09000435319733E-16,2.91501601757459E-15,
-1.));
#22450=DIRECTION('ref_axis',(0.236333478439911,0.971672005858197,3.E-15));
#22451=DIRECTION('center_axis',(7.09000435319733E-16,2.91501601757459E-15,
-1.));
#22452=DIRECTION('ref_axis',(0.236333478439911,0.971672005858197,3.E-15));
#22453=DIRECTION('center_axis',(7.09000435319733E-16,2.91501601757459E-15,
-1.));
#22454=DIRECTION('ref_axis',(0.236333478439911,0.971672005858197,3.E-15));
#22455=DIRECTION('center_axis',(7.09000435319733E-16,2.91501601757459E-15,
-1.));
#22456=DIRECTION('ref_axis',(-0.971672005858197,0.236333478439911,-1.18897715061811E-32));
#22457=DIRECTION('center_axis',(7.09000435319733E-16,2.91501601757459E-15,
-1.));
#22458=DIRECTION('ref_axis',(0.236333478439911,0.971672005858197,3.E-15));
#22459=DIRECTION('center_axis',(7.09000435319733E-16,2.91501601757459E-15,
-1.));
#22460=DIRECTION('ref_axis',(-0.971672005858197,0.236333478439911,-1.18897715061811E-32));
#22461=DIRECTION('center_axis',(-7.09000435319733E-16,-2.91501601757459E-15,
1.));
#22462=DIRECTION('ref_axis',(-0.236333478439916,-0.971672005858196,-3.E-15));
#22463=DIRECTION('center_axis',(-7.09000435319733E-16,-2.91501601757459E-15,
1.));
#22464=DIRECTION('ref_axis',(-0.236333478439916,-0.971672005858196,-3.E-15));
#22465=DIRECTION('center_axis',(7.09000435319733E-16,2.91501601757459E-15,
-1.));
#22466=DIRECTION('ref_axis',(-0.971672005858197,0.236333478439911,-1.18897715061811E-32));
#22467=DIRECTION('center_axis',(-7.09000435319733E-16,-2.91501601757459E-15,
1.));
#22468=DIRECTION('ref_axis',(-0.236333478439908,-0.971672005858198,-3.E-15));
#22469=DIRECTION('center_axis',(7.09000435319733E-16,2.91501601757459E-15,
-1.));
#22470=DIRECTION('ref_axis',(-0.971672005858197,0.236333478439911,-1.18897715061811E-32));
#22471=DIRECTION('center_axis',(-7.09000435319733E-16,-2.91501601757459E-15,
1.));
#22472=DIRECTION('ref_axis',(-0.236333478439909,-0.971672005858198,-3.E-15));
#22473=DIRECTION('center_axis',(7.09000435319733E-16,2.91501601757459E-15,
-1.));
#22474=DIRECTION('ref_axis',(-0.971672005858197,0.236333478439911,-1.18897715061811E-32));
#22475=DIRECTION('center_axis',(-7.09000435319733E-16,-2.91501601757459E-15,
1.));
#22476=DIRECTION('ref_axis',(-0.236333478439911,-0.971672005858197,-3.E-15));
#22477=DIRECTION('center_axis',(7.09000435319733E-16,2.91501601757459E-15,
-1.));
#22478=DIRECTION('ref_axis',(0.236333478439916,0.971672005858196,3.E-15));
#22479=DIRECTION('center_axis',(-7.09000435319733E-16,-2.91501601757459E-15,
1.));
#22480=DIRECTION('ref_axis',(-0.236333478439916,-0.971672005858196,-3.E-15));
#22481=DIRECTION('',(7.09000435319733E-16,2.91501601757459E-15,-1.));
#22482=DIRECTION('center_axis',(-7.09000435319733E-16,-2.91501601757459E-15,
1.));
#22483=DIRECTION('ref_axis',(-0.236333478439916,-0.971672005858196,-3.E-15));
#22484=DIRECTION('center_axis',(7.09000435319733E-16,2.91501601757459E-15,
-1.));
#22485=DIRECTION('ref_axis',(0.236333478439908,0.971672005858198,3.E-15));
#22486=DIRECTION('center_axis',(-7.09000435319733E-16,-2.91501601757459E-15,
1.));
#22487=DIRECTION('ref_axis',(-0.236333478439908,-0.971672005858198,-3.E-15));
#22488=DIRECTION('',(7.09000435319733E-16,2.91501601757459E-15,-1.));
#22489=DIRECTION('center_axis',(-7.09000435319733E-16,-2.91501601757459E-15,
1.));
#22490=DIRECTION('ref_axis',(-0.236333478439908,-0.971672005858198,-3.E-15));
#22491=DIRECTION('center_axis',(-7.09000435319733E-16,-2.91501601757459E-15,
1.));
#22492=DIRECTION('ref_axis',(-0.236333478439908,-0.971672005858198,-3.E-15));
#22493=DIRECTION('center_axis',(7.09000435319733E-16,2.91501601757459E-15,
-1.));
#22494=DIRECTION('ref_axis',(0.236333478439909,0.971672005858198,3.E-15));
#22495=DIRECTION('center_axis',(-7.09000435319733E-16,-2.91501601757459E-15,
1.));
#22496=DIRECTION('ref_axis',(-0.236333478439909,-0.971672005858198,-3.E-15));
#22497=DIRECTION('',(7.09000435319733E-16,2.91501601757459E-15,-1.));
#22498=DIRECTION('center_axis',(-7.09000435319733E-16,-2.91501601757459E-15,
1.));
#22499=DIRECTION('ref_axis',(-0.236333478439909,-0.971672005858198,-3.E-15));
#22500=DIRECTION('center_axis',(-7.09000435319733E-16,-2.91501601757459E-15,
1.));
#22501=DIRECTION('ref_axis',(-0.236333478439909,-0.971672005858198,-3.E-15));
#22502=DIRECTION('center_axis',(7.09000435319733E-16,2.91501601757459E-15,
-1.));
#22503=DIRECTION('ref_axis',(0.236333478439911,0.971672005858197,3.E-15));
#22504=DIRECTION('center_axis',(-7.09000435319733E-16,-2.91501601757459E-15,
1.));
#22505=DIRECTION('ref_axis',(-0.236333478439911,-0.971672005858197,-3.E-15));
#22506=DIRECTION('',(7.09000435319733E-16,2.91501601757459E-15,-1.));
#22507=DIRECTION('center_axis',(-7.09000435319733E-16,-2.91501601757459E-15,
1.));
#22508=DIRECTION('ref_axis',(-0.236333478439911,-0.971672005858197,-3.E-15));
#22509=DIRECTION('center_axis',(-7.09000435319733E-16,-2.91501601757459E-15,
1.));
#22510=DIRECTION('ref_axis',(-0.236333478439911,-0.971672005858197,-3.E-15));
#22511=DIRECTION('center_axis',(7.09000435319733E-16,2.91501601757459E-15,
-1.));
#22512=DIRECTION('ref_axis',(0.236333478439911,0.971672005858197,3.E-15));
#22513=DIRECTION('',(7.09000435319733E-16,2.91501601757459E-15,-1.));
#22514=DIRECTION('center_axis',(0.,0.,-1.));
#22515=DIRECTION('ref_axis',(1.,0.,0.));
#22516=DIRECTION('center_axis',(0.236333478439914,0.971672005858196,3.E-15));
#22517=DIRECTION('ref_axis',(-7.09000435319733E-16,-2.91501601757459E-15,
1.));
#22518=DIRECTION('',(0.971672005858196,-0.236333478439914,-9.36576430249746E-30));
#22519=DIRECTION('',(7.09000435319733E-16,2.91501601757459E-15,-1.));
#22520=DIRECTION('',(0.971672005858196,-0.236333478439914,-9.36576430249746E-30));
#22521=DIRECTION('',(7.09000435319733E-16,2.91501601757459E-15,-1.));
#22522=DIRECTION('center_axis',(-0.920977002765036,-0.389616940568464,-1.78871271835535E-15));
#22523=DIRECTION('ref_axis',(7.09000435319733E-16,2.91501601757459E-15,
-1.));
#22524=DIRECTION('',(-0.389616940568464,0.920977002765036,2.40842413440694E-15));
#22525=DIRECTION('',(-0.389616940568464,0.920977002765036,2.40842413440694E-15));
#22526=DIRECTION('',(7.09000435319733E-16,2.91501601757459E-15,-1.));
#22527=DIRECTION('center_axis',(0.36926410344504,0.929324497636284,2.97080420622471E-15));
#22528=DIRECTION('ref_axis',(-7.09000435319733E-16,-2.91501601757459E-15,
1.));
#22529=DIRECTION('',(0.929324497636283,-0.36926410344504,-4.17519302880196E-16));
#22530=DIRECTION('',(0.929324497636283,-0.36926410344504,-4.17519302880196E-16));
#22531=DIRECTION('',(7.09000435319733E-16,2.91501601757459E-15,-1.));
#22532=DIRECTION('center_axis',(-0.966238315689019,-0.257649989898017,-1.43611723392677E-15));
#22533=DIRECTION('ref_axis',(7.09000435319733E-16,2.91501601757459E-15,
-1.));
#22534=DIRECTION('',(-0.257649989898017,0.966238315689019,2.63392621202997E-15));
#22535=DIRECTION('',(-0.257649989898017,0.966238315689019,2.63392621202997E-15));
#22536=DIRECTION('',(7.09000435319733E-16,2.91501601757459E-15,-1.));
#22537=DIRECTION('center_axis',(0.495007422708304,0.868888745158828,2.88378508781496E-15));
#22538=DIRECTION('ref_axis',(-7.09000435319733E-16,-2.91501601757459E-15,
1.));
#22539=DIRECTION('',(0.868888745158828,-0.495007422708304,-8.26912067450997E-16));
#22540=DIRECTION('',(0.868888745158828,-0.495007422708304,-8.26912067450997E-16));
#22541=DIRECTION('',(7.09000435319733E-16,2.91501601757459E-15,-1.));
#22542=DIRECTION('center_axis',(-0.992692898877909,-0.120668175246722,-1.05556936109894E-15));
#22543=DIRECTION('ref_axis',(7.09000435319733E-16,2.91501601757459E-15,
-1.));
#22544=DIRECTION('',(-0.120668175246722,0.992692898877909,2.80816191198249E-15));
#22545=DIRECTION('',(-0.120668175246722,0.992692898877909,2.80816191198249E-15));
#22546=DIRECTION('',(7.09000435319733E-16,2.91501601757459E-15,-1.));
#22547=DIRECTION('center_axis',(0.611115985551149,0.791541061603154,2.7406363729278E-15));
#22548=DIRECTION('ref_axis',(-7.09000435319733E-16,-2.91501601757459E-15,
1.));
#22549=DIRECTION('',(0.791541061603154,-0.611115985551148,-1.2202099292274E-15));
#22550=DIRECTION('',(0.791541061603154,-0.611115985551148,-1.2202099292274E-15));
#22551=DIRECTION('',(7.09000435319733E-16,2.91501601757459E-15,-1.));
#22552=DIRECTION('center_axis',(-0.999825843961577,0.0186623081777341,-6.54476031349669E-16));
#22553=DIRECTION('ref_axis',(7.09000435319733E-16,2.91501601757459E-15,
-1.));
#22554=DIRECTION('',(0.0186623081777341,0.999825843961577,2.92773993455511E-15));
#22555=DIRECTION('',(0.0186623081777341,0.999825843961577,2.92773993455511E-15));
#22556=DIRECTION('',(7.09000435319733E-16,2.91501601757459E-15,-1.));
#22557=DIRECTION('center_axis',(0.71532987086937,0.698786931647988,2.54414428846928E-15));
#22558=DIRECTION('ref_axis',(-7.09000435319733E-16,-2.91501601757459E-15,
1.));
#22559=DIRECTION('',(0.698786931647988,-0.71532987086937,-1.58975779269962E-15));
#22560=DIRECTION('',(0.698786931647988,-0.71532987086937,-1.58975779269962E-15));
#22561=DIRECTION('',(7.09000435319733E-16,2.91501601757459E-15,-1.));
#22562=DIRECTION('center_axis',(-0.987498316277574,0.157629551001571,-2.40644070105632E-16));
#22563=DIRECTION('ref_axis',(7.09000435319733E-16,2.91501601757459E-15,
-1.));
#22564=DIRECTION('',(0.157629551001571,0.987498316277574,2.99033282955644E-15));
#22565=DIRECTION('',(0.157629551001571,0.987498316277574,2.99033282955644E-15));
#22566=DIRECTION('',(7.09000435319733E-16,2.91501601757459E-15,-1.));
#22567=DIRECTION('center_axis',(0.805620673926787,0.592431708926649,2.29813332935694E-15));
#22568=DIRECTION('ref_axis',(-7.09000435319733E-16,-2.91501601757459E-15,
1.));
#22569=DIRECTION('',(0.592431708926649,-0.805620673926787,-1.92836282905961E-15));
#22570=DIRECTION('',(0.592431708926649,-0.805620673926787,-1.92836282905961E-15));
#22571=DIRECTION('',(7.09000435319733E-16,2.91501601757459E-15,-1.));
#22572=DIRECTION('center_axis',(-0.955950257129914,0.293528713916121,1.77871754234442E-16));
#22573=DIRECTION('ref_axis',(0.293528713916121,0.955950257129914,2.99472229748362E-15));
#22574=DIRECTION('',(0.293528713916121,0.955950257129914,2.99472229748362E-15));
#22575=DIRECTION('',(0.293528713916121,0.955950257129914,2.99472229748362E-15));
#22576=DIRECTION('',(7.09000435319733E-16,2.91501601757459E-15,-1.));
#22577=DIRECTION('center_axis',(0.880230986946155,0.474545476872131,2.00739181907658E-15));
#22578=DIRECTION('ref_axis',(-7.09000435319733E-16,-2.91501601757459E-15,
1.));
#22579=DIRECTION('',(0.474545476872131,-0.880230986946155,-2.22943447643218E-15));
#22580=DIRECTION('',(0.474545476872131,-0.880230986946155,-2.22943447643218E-15));
#22581=DIRECTION('',(7.09000435319733E-16,2.91501601757459E-15,-1.));
#22582=DIRECTION('center_axis',(-0.905795713604521,0.423714674298256,5.92925507204465E-16));
#22583=DIRECTION('ref_axis',(0.423714674298256,0.90579571360452,2.94082290233641E-15));
#22584=DIRECTION('',(0.423714674298256,0.905795713604521,2.94082290233641E-15));
#22585=DIRECTION('',(0.423714674298256,0.905795713604521,2.94082290233641E-15));
#22586=DIRECTION('',(7.09000435319733E-16,2.91501601757459E-15,-1.));
#22587=DIRECTION('center_axis',(0.937708605052523,0.347422756897777,1.67757871041224E-15));
#22588=DIRECTION('ref_axis',(-7.09000435319733E-16,-2.91501601757459E-15,
1.));
#22589=DIRECTION('',(0.347422756897777,-0.937708605052523,-2.48711271766512E-15));
#22590=DIRECTION('',(0.347422756897777,-0.937708605052523,-2.48711271766512E-15));
#22591=DIRECTION('',(7.09000435319733E-16,2.91501601757459E-15,-1.));
#22592=DIRECTION('center_axis',(-0.838010886841169,0.545653510513474,9.96438639619516E-16));
#22593=DIRECTION('ref_axis',(0.545653510513474,0.838010886841169,2.82968373453169E-15));
#22594=DIRECTION('',(0.545653510513474,0.838010886841169,2.82968373453169E-15));
#22595=DIRECTION('',(0.545653510513474,0.838010886841169,2.82968373453169E-15));
#22596=DIRECTION('',(7.09000435319733E-16,2.91501601757459E-15,-1.));
#22597=DIRECTION('center_axis',(0.976934791789272,0.213537848147936,1.31511344036723E-15));
#22598=DIRECTION('ref_axis',(-7.09000435319733E-16,-2.91501601757459E-15,
1.));
#22599=DIRECTION('',(0.213537848147936,-0.976934791789272,-2.6963821388975E-15));
#22600=DIRECTION('',(0.213537848147936,-0.976934791789272,-2.6963821388975E-15));
#22601=DIRECTION('',(7.09000435319733E-16,2.91501601757459E-15,-1.));
#22602=DIRECTION('center_axis',(-0.753915131388709,0.656971821818216,1.38055722734653E-15));
#22603=DIRECTION('ref_axis',(0.656971821818216,0.753915131388709,2.66346799155185E-15));
#22604=DIRECTION('',(0.656971821818216,0.753915131388709,2.66346799155185E-15));
#22605=DIRECTION('',(0.656971821818216,0.753915131388709,2.66346799155185E-15));
#22606=DIRECTION('',(7.09000435319733E-16,2.91501601757459E-15,-1.));
#22607=DIRECTION('center_axis',(0.997146054050699,0.0754966680795983,9.27050983124841E-16));
#22608=DIRECTION('ref_axis',(-7.09000435319733E-16,-2.91501601757459E-15,
1.));
#22609=DIRECTION('',(0.0754966680795983,-0.997146054050699,-2.85316954888546E-15));
#22610=DIRECTION('',(0.0754966680795983,-0.997146054050699,-2.85316954888546E-15));
#22611=DIRECTION('',(7.09000435319733E-16,2.91501601757459E-15,-1.));
#22612=DIRECTION('center_axis',(-0.65514527546952,0.755502923905637,1.73780483900381E-15));
#22613=DIRECTION('ref_axis',(0.755502923905637,0.65514527546952,2.4454108737664E-15));
#22614=DIRECTION('',(0.755502923905637,0.65514527546952,2.4454108737664E-15));
#22615=DIRECTION('',(0.755502923905637,0.65514527546952,2.4454108737664E-15));
#22616=DIRECTION('',(7.09000435319733E-16,2.91501601757459E-15,-1.));
#22617=DIRECTION('center_axis',(0.997949002606853,-0.064013968756721,5.20944533000791E-16));
#22618=DIRECTION('ref_axis',(-7.09000435319733E-16,-2.91501601757459E-15,
1.));
#22619=DIRECTION('',(-0.0640139687567209,-0.997949002606853,-2.95442325903662E-15));
#22620=DIRECTION('',(-0.0640139687567209,-0.997949002606853,-2.95442325903662E-15));
#22621=DIRECTION('',(7.09000435319733E-16,2.91501601757459E-15,-1.));
#22622=DIRECTION('center_axis',(-0.543623761980021,0.839329020951075,2.0612280561936E-15));
#22623=DIRECTION('ref_axis',(0.839329020951075,0.543623761980021,2.17975661493672E-15));
#22624=DIRECTION('',(0.839329020951074,0.543623761980021,2.17975661493672E-15));
#22625=DIRECTION('',(0.839329020951074,0.543623761980021,2.17975661493672E-15));
#22626=DIRECTION('',(7.09000435319733E-16,2.91501601757459E-15,-1.));
#22627=DIRECTION('center_axis',(0.979328008977431,-0.202278646506002,1.04698490107502E-16));
#22628=DIRECTION('ref_axis',(-7.09000435319733E-16,-2.91501601757459E-15,
1.));
#22629=DIRECTION('',(-0.202278646506002,-0.979328008977431,-2.99817248105729E-15));
#22630=DIRECTION('',(-0.202278646506002,-0.979328008977431,-2.99817248105729E-15));
#22631=DIRECTION('',(7.09000435319733E-16,2.91501601757459E-15,-1.));
#22632=DIRECTION('center_axis',(-0.421521230326446,0.90681853332631,2.34453181388173E-15));
#22633=DIRECTION('ref_axis',(0.90681853332631,0.421521230326446,1.87167587303369E-15));
#22634=DIRECTION('',(0.90681853332631,0.421521230326446,1.87167587303369E-15));
#22635=DIRECTION('',(0.90681853332631,0.421521230326446,1.87167587303369E-15));
#22636=DIRECTION('',(7.09000435319733E-16,2.91501601757459E-15,-1.));
#22637=DIRECTION('center_axis',(0.941645509622363,-0.336606200489593,-3.13585389802961E-16));
#22638=DIRECTION('ref_axis',(7.09000435319733E-16,2.91501601757459E-15,
-1.));
#22639=DIRECTION('',(-0.336606200489593,-0.941645509622363,-2.98356568610482E-15));
#22640=DIRECTION('',(-0.336606200489593,-0.941645509622363,-2.98356568610482E-15));
#22641=DIRECTION('',(7.09000435319733E-16,2.91501601757459E-15,-1.));
#22642=DIRECTION('center_axis',(-0.29121426739786,0.956657854441141,2.58220192667807E-15));
#22643=DIRECTION('ref_axis',(0.956657854441141,0.29121426739786,1.52716508926182E-15));
#22644=DIRECTION('',(0.956657854441142,0.291214267397859,1.52716508926182E-15));
#22645=DIRECTION('',(0.956657854441142,0.291214267397859,1.52716508926182E-15));
#22646=DIRECTION('',(7.09000435319733E-16,2.91501601757459E-15,-1.));
#22647=DIRECTION('center_axis',(0.885634951528387,-0.464382097664533,-7.25765686799004E-16));
#22648=DIRECTION('ref_axis',(7.09000435319733E-16,2.91501601757459E-15,
-1.));
#22649=DIRECTION('',(-0.464382097664533,-0.885634951528387,-2.91088717882799E-15));
#22650=DIRECTION('',(-0.464382097664533,-0.885634951528387,-2.91088717882799E-15));
#22651=DIRECTION('',(7.09000435319733E-16,2.91501601757459E-15,-1.));
#22652=DIRECTION('center_axis',(-0.155239150005693,0.987876918601457,2.76961241618278E-15));
#22653=DIRECTION('ref_axis',(0.987876918601457,0.155239150005693,1.15292977415201E-15));
#22654=DIRECTION('',(0.987876918601457,0.155239150005693,1.15292977415201E-15));
#22655=DIRECTION('',(0.987876918601457,0.155239150005693,1.15292977415201E-15));
#22656=DIRECTION('',(7.09000435319733E-16,2.91501601757459E-15,-1.));
#22657=DIRECTION('center_axis',(0.812386516497737,-0.583119325535239,-1.12381978024774E-15));
#22658=DIRECTION('ref_axis',(7.09000435319733E-16,2.91501601757459E-15,
-1.));
#22659=DIRECTION('',(-0.583119325535239,-0.812386516497737,-2.78155156370036E-15));
#22660=DIRECTION('',(-0.583119325535239,-0.812386516497737,-2.78155156370036E-15));
#22661=DIRECTION('',(7.09000435319733E-16,2.91501601757459E-15,-1.));
#22662=DIRECTION('center_axis',(-0.0162424791405826,0.999868082234535,2.90311555039392E-15));
#22663=DIRECTION('ref_axis',(0.999868082234536,0.0162424791405826,7.56253992426512E-16));
#22664=DIRECTION('',(0.999868082234535,0.0162424791405826,7.56253992426512E-16));
#22665=DIRECTION('',(0.999868082234535,0.0162424791405826,7.56253992426512E-16));
#22666=DIRECTION('',(7.09000435319733E-16,2.91501601757459E-15,-1.));
#22667=DIRECTION('center_axis',(0.723325901999425,-0.690506799022803,-1.5E-15));
#22668=DIRECTION('ref_axis',(7.09000435319733E-16,2.91501601757459E-15,
-1.));
#22669=DIRECTION('',(-0.690506799022803,-0.723325901999425,-2.59807621135332E-15));
#22670=DIRECTION('',(-0.690506799022803,-0.723325901999425,-2.59807621135332E-15));
#22671=DIRECTION('',(7.09000435319733E-16,2.91501601757459E-15,-1.));
#22672=DIRECTION('center_axis',(0.123070333105456,0.992397950980005,2.98011284266163E-15));
#22673=DIRECTION('ref_axis',(0.992397950980005,-0.123070333105456,3.4485858696459E-16));
#22674=DIRECTION('',(0.992397950980005,-0.123070333105456,3.4485858696459E-16));
#22675=DIRECTION('',(0.992397950980005,-0.123070333105456,3.4485858696459E-16));
#22676=DIRECTION('',(7.09000435319733E-16,2.91501601757459E-15,-1.));
#22677=DIRECTION('center_axis',(0.620186571589713,-0.784454343107231,-1.84698442597697E-15));
#22678=DIRECTION('ref_axis',(7.09000435319733E-16,2.91501601757459E-15,
-1.));
#22679=DIRECTION('',(-0.784454343107231,-0.620186571589714,-2.36403226082017E-15));
#22680=DIRECTION('',(-0.784454343107231,-0.620186571589714,-2.36403226082017E-15));
#22681=DIRECTION('',(7.09000435319733E-16,2.91501601757459E-15,-1.));
#22682=DIRECTION('center_axis',(0.259987721308024,0.965611922445586,2.99910562827505E-15));
#22683=DIRECTION('ref_axis',(-7.09000435319733E-16,-2.91501601757459E-15,
1.));
#22684=DIRECTION('',(0.965611922445586,-0.259987721308024,-7.32490986217644E-17));
#22685=DIRECTION('',(0.965611922445586,-0.259987721308024,-7.32490986217644E-17));
#22686=DIRECTION('',(7.09000435319733E-16,2.91501601757459E-15,-1.));
#22687=DIRECTION('center_axis',(0.504976015015775,-0.863133375706668,-2.15801940101596E-15));
#22688=DIRECTION('ref_axis',(7.09000435319733E-16,2.91501601757459E-15,
-1.));
#22689=DIRECTION('',(-0.863133375706668,-0.504976015015775,-2.08397511137699E-15));
#22690=DIRECTION('',(-0.863133375706668,-0.504976015015775,-2.08397511137699E-15));
#22691=DIRECTION('',(7.09000435319733E-16,2.91501601757459E-15,-1.));
#22692=DIRECTION('center_axis',(0.391844744246979,0.920031356208048,2.95972423426619E-15));
#22693=DIRECTION('ref_axis',(-7.09000435319733E-16,-2.91501601757459E-15,
1.));
#22694=DIRECTION('',(0.920031356208048,-0.391844744246979,-4.89931073823054E-16));
#22695=DIRECTION('',(0.920031356208048,-0.391844744246979,-4.89931073823054E-16));
#22696=DIRECTION('',(7.09000435319733E-16,2.91501601757459E-15,-1.));
#22697=DIRECTION('center_axis',(0.37993667471126,-0.925012498947636,-2.42705098312484E-15));
#22698=DIRECTION('ref_axis',(7.09000435319733E-16,2.91501601757459E-15,
-1.));
#22699=DIRECTION('',(-0.925012498947636,-0.37993667471126,-1.76335575687742E-15));
#22700=DIRECTION('',(-0.925012498947636,-0.37993667471126,-1.76335575687742E-15));
#22701=DIRECTION('',(7.09000435319733E-16,2.91501601757459E-15,-1.));
#22702=DIRECTION('center_axis',(0.516074954955961,0.856543426142074,2.86273517467375E-15));
#22703=DIRECTION('ref_axis',(-7.09000435319733E-16,-2.91501601757459E-15,
1.));
#22704=DIRECTION('',(0.856543426142074,-0.516074954955961,-8.97077097960726E-16));
#22705=DIRECTION('',(0.856543426142074,-0.516074954955961,-8.97077097960726E-16));
#22706=DIRECTION('',(7.09000435319733E-16,2.91501601757459E-15,-1.));
#22707=DIRECTION('center_axis',(0.247502299205053,-0.968887306082711,-2.64884277857678E-15));
#22708=DIRECTION('ref_axis',(7.09000435319733E-16,2.91501601757459E-15,
-1.));
#22709=DIRECTION('',(-0.968887306082711,-0.247502299205053,-1.40841468835767E-15));
#22710=DIRECTION('',(-0.968887306082711,-0.247502299205053,-1.40841468835767E-15));
#22711=DIRECTION('',(7.09000435319733E-16,2.91501601757459E-15,-1.));
#22712=DIRECTION('center_axis',(0.630260353693282,0.776383852589954,2.71002623121929E-15));
#22713=DIRECTION('ref_axis',(-7.09000435319733E-16,-2.91501601757459E-15,
1.));
#22714=DIRECTION('',(0.776383852589954,-0.630260353693282,-1.28676253679666E-15));
#22715=DIRECTION('',(0.776383852589954,-0.630260353693282,-1.28676253679666E-15));
#22716=DIRECTION('',(7.09000435319733E-16,2.91501601757459E-15,-1.));
#22717=DIRECTION('center_axis',(0.110250572974511,-0.993903823897862,-2.81907786235772E-15));
#22718=DIRECTION('ref_axis',(7.09000435319733E-16,2.91501601757459E-15,
-1.));
#22719=DIRECTION('',(-0.993903823897862,-0.110250572974511,-1.02606042997701E-15));
#22720=DIRECTION('',(-0.993903823897862,-0.110250572974511,-1.02606042997701E-15));
#22721=DIRECTION('',(7.09000435319733E-16,2.91501601757459E-15,-1.));
#22722=DIRECTION('center_axis',(0.732178451556494,0.68111285047071,2.50456970978329E-15));
#22723=DIRECTION('ref_axis',(-7.09000435319733E-16,-2.91501601757459E-15,
1.));
#22724=DIRECTION('',(0.68111285047071,-0.732178451556494,-1.65140260652454E-15));
#22725=DIRECTION('',(0.68111285047071,-0.732178451556494,-1.65140260652454E-15));
#22726=DIRECTION('',(7.09000435319733E-16,2.91501601757459E-15,-1.));
#22727=DIRECTION('center_axis',(-0.029147055250812,-0.999575134329684,-2.93444280220142E-15));
#22728=DIRECTION('ref_axis',(7.09000435319733E-16,2.91501601757459E-15,
-1.));
#22729=DIRECTION('',(-0.999575134329684,0.029147055250812,-6.23735072453278E-16));
#22730=DIRECTION('',(-0.999575134329684,0.029147055250812,-6.23735072453278E-16));
#22731=DIRECTION('',(7.09000435319733E-16,2.91501601757459E-15,-1.));
#22732=DIRECTION('center_axis',(0.819845528700799,0.572584761471442,2.25036458785218E-15));
#22733=DIRECTION('ref_axis',(-7.09000435319733E-16,-2.91501601757459E-15,
1.));
#22734=DIRECTION('',(0.572584761471442,-0.819845528700799,-1.98390000295904E-15));
#22735=DIRECTION('',(0.572584761471442,-0.819845528700799,-1.98390000295904E-15));
#22736=DIRECTION('',(7.09000435319733E-16,2.91501601757459E-15,-1.));
#22737=DIRECTION('center_axis',(-0.167977369199961,-0.985790851771642,-2.99269215077947E-15));
#22738=DIRECTION('ref_axis',(7.09000435319733E-16,2.91501601757459E-15,
-1.));
#22739=DIRECTION('',(-0.985790851771642,0.167977369199961,-2.09269421232377E-16));
#22740=DIRECTION('',(-0.985790851771642,0.167977369199961,-2.09269421232377E-16));
#22741=DIRECTION('',(7.09000435319733E-16,2.91501601757459E-15,-1.));
#22742=DIRECTION('center_axis',(0.891555245189413,0.45291196139564,1.9523586789703E-15));
#22743=DIRECTION('ref_axis',(-7.09000435319733E-16,-2.91501601757459E-15,
1.));
#22744=DIRECTION('',(0.45291196139564,-0.891555245189413,-2.27778304248876E-15));
#22745=DIRECTION('',(0.45291196139564,-0.891555245189413,-2.27778304248876E-15));
#22746=DIRECTION('',(7.09000435319733E-16,2.91501601757459E-15,-1.));
#22747=DIRECTION('center_axis',(-0.303538194729059,-0.952819271604339,-2.99269215077947E-15));
#22748=DIRECTION('ref_axis',(7.09000435319733E-16,2.91501601757459E-15,
-1.));
#22749=DIRECTION('',(-0.952819271604339,0.303538194729059,2.09269421232376E-16));
#22750=DIRECTION('',(-0.952819271604339,0.303538194729059,2.09269421232376E-16));
#22751=DIRECTION('',(7.09000435319733E-16,2.91501601757459E-15,-1.));
#22752=DIRECTION('center_axis',(0.945911852959474,0.324423745170996,1.61635232917735E-15));
#22753=DIRECTION('ref_axis',(-7.09000435319733E-16,-2.91501601757459E-15,
1.));
#22754=DIRECTION('',(0.324423745170996,-0.945911852959474,-2.52733162603623E-15));
#22755=DIRECTION('',(0.324423745170996,-0.945911852959474,-2.52733162603623E-15));
#22756=DIRECTION('',(7.09000435319733E-16,2.91501601757459E-15,-1.));
#22757=DIRECTION('center_axis',(-0.433190994567335,-0.901302148131115,-2.93444280220142E-15));
#22758=DIRECTION('ref_axis',(7.09000435319733E-16,2.91501601757459E-15,
-1.));
#22759=DIRECTION('',(-0.901302148131115,0.433190994567335,6.23735072453278E-16));
#22760=DIRECTION('',(-0.901302148131115,0.433190994567335,6.23735072453278E-16));
#22761=DIRECTION('',(7.09000435319733E-16,2.91501601757459E-15,-1.));
#22762=DIRECTION('center_axis',(0.981857362470463,0.18962098977314,1.24888551987049E-15));
#22763=DIRECTION('ref_axis',(-7.09000435319733E-16,-2.91501601757459E-15,
1.));
#22764=DIRECTION('',(0.18962098977314,-0.981857362470463,-2.72768857428003E-15));
#22765=DIRECTION('',(0.18962098977314,-0.981857362470463,-2.72768857428003E-15));
#22766=DIRECTION('',(7.09000435319733E-16,2.91501601757459E-15,-1.));
#22767=DIRECTION('center_axis',(-0.554412224443811,-0.832242203560517,-2.81907786235773E-15));
#22768=DIRECTION('ref_axis',(7.09000435319733E-16,2.91501601757459E-15,
-1.));
#22769=DIRECTION('',(-0.832242203560517,0.554412224443811,1.02606042997701E-15));
#22770=DIRECTION('',(-0.832242203560517,0.554412224443811,1.02606042997701E-15));
#22771=DIRECTION('',(7.09000435319733E-16,2.91501601757459E-15,-1.));
#22772=DIRECTION('center_axis',(0.998692135267162,0.0511274775000253,8.5711057450557E-16));
#22773=DIRECTION('ref_axis',(-7.09000435319733E-16,-2.91501601757459E-15,
1.));
#22774=DIRECTION('',(0.0511274775000253,-0.998692135267162,-2.87495416712523E-15));
#22775=DIRECTION('',(0.0511274775000253,-0.998692135267162,-2.87495416712523E-15));
#22776=DIRECTION('',(7.09000435319733E-16,2.91501601757459E-15,-1.));
#22777=DIRECTION('center_axis',(-0.664842451006046,-0.74698361115909,-2.64884277857678E-15));
#22778=DIRECTION('ref_axis',(7.09000435319733E-16,2.91501601757459E-15,
-1.));
#22779=DIRECTION('',(-0.746983611159089,0.664842451006046,1.40841468835767E-15));
#22780=DIRECTION('',(-0.746983611159089,0.664842451006046,1.40841468835767E-15));
#22781=DIRECTION('',(7.09000435319733E-16,2.91501601757459E-15,-1.));
#22782=DIRECTION('center_axis',(0.996088501646353,-0.0883611729659795,4.48652946756736E-16));
#22783=DIRECTION('ref_axis',(-7.09000435319733E-16,-2.91501601757459E-15,
1.));
#22784=DIRECTION('',(-0.0883611729659795,-0.996088501646353,-2.96626204731923E-15));
#22785=DIRECTION('',(-0.0883611729659795,-0.996088501646353,-2.96626204731923E-15));
#22786=DIRECTION('',(7.09000435319733E-16,2.91501601757459E-15,-1.));
#22787=DIRECTION('center_axis',(-0.762332275506527,-0.647185832447714,-2.42705098312484E-15));
#22788=DIRECTION('ref_axis',(7.09000435319733E-16,2.91501601757459E-15,
-1.));
#22789=DIRECTION('',(-0.647185832447714,0.762332275506527,1.76335575687742E-15));
#22790=DIRECTION('',(-0.647185832447714,0.762332275506527,1.76335575687742E-15));
#22791=DIRECTION('',(7.09000435319733E-16,2.91501601757459E-15,-1.));
#22792=DIRECTION('center_axis',(0.974097138374874,-0.22612997370955,3.14627997344311E-17));
#22793=DIRECTION('ref_axis',(-7.09000435319733E-16,-2.91501601757459E-15,
1.));
#22794=DIRECTION('',(-0.22612997370955,-0.974097138374874,-2.99983501083524E-15));
#22795=DIRECTION('',(-0.22612997370955,-0.974097138374874,-2.99983501083524E-15));
#22796=DIRECTION('',(7.09000435319733E-16,2.91501601757459E-15,-1.));
#22797=DIRECTION('center_axis',(-0.844984169404384,-0.534791317670718,-2.15801940101595E-15));
#22798=DIRECTION('ref_axis',(7.09000435319733E-16,2.91501601757459E-15,
-1.));
#22799=DIRECTION('',(-0.534791317670718,0.844984169404384,2.08397511137699E-15));
#22800=DIRECTION('',(-0.534791317670718,0.844984169404384,2.08397511137699E-15));
#22801=DIRECTION('',(7.09000435319733E-16,2.91501601757459E-15,-1.));
#22802=DIRECTION('center_axis',(0.933146082324,-0.359497411733896,-3.86339734896295E-16));
#22803=DIRECTION('ref_axis',(7.09000435319733E-16,2.91501601757459E-15,
-1.));
#22804=DIRECTION('',(-0.359497411733896,-0.933146082324,-2.97501959812709E-15));
#22805=DIRECTION('',(-0.359497411733896,-0.933146082324,-2.97501959812709E-15));
#22806=DIRECTION('',(7.09000435319733E-16,2.91501601757459E-15,-1.));
#22807=DIRECTION('center_axis',(-0.911189407600033,-0.411987698211368,-1.84698442597698E-15));
#22808=DIRECTION('ref_axis',(7.09000435319733E-16,2.91501601757459E-15,
-1.));
#22809=DIRECTION('',(-0.411987698211368,0.911189407600033,2.36403226082016E-15));
#22810=DIRECTION('',(-0.411987698211368,0.911189407600033,2.36403226082016E-15));
#22811=DIRECTION('',(7.09000435319733E-16,2.91501601757459E-15,-1.));
#22812=DIRECTION('center_axis',(0.874032399218628,-0.485867641561083,-7.96622606042188E-16));
#22813=DIRECTION('ref_axis',(7.09000435319733E-16,2.91501601757459E-15,
-1.));
#22814=DIRECTION('',(-0.485867641561083,-0.874032399218628,-2.89229881297603E-15));
#22815=DIRECTION('',(-0.485867641561083,-0.874032399218628,-2.89229881297603E-15));
#22816=DIRECTION('',(7.09000435319733E-16,2.91501601757459E-15,-1.));
#22817=DIRECTION('center_axis',(-0.959659380439336,-0.281165206835394,-1.5E-15));
#22818=DIRECTION('ref_axis',(7.09000435319733E-16,2.91501601757459E-15,
-1.));
#22819=DIRECTION('',(-0.281165206835394,0.959659380439336,2.59807621135332E-15));
#22820=DIRECTION('',(-0.281165206835394,0.959659380439336,2.59807621135332E-15));
#22821=DIRECTION('',(7.09000435319733E-16,2.91501601757459E-15,-1.));
#22822=DIRECTION('center_axis',(0.797906669659581,-0.60278101041154,-1.19140012430627E-15));
#22823=DIRECTION('ref_axis',(7.09000435319733E-16,2.91501601757459E-15,
-1.));
#22824=DIRECTION('',(-0.60278101041154,-0.797906669659581,-2.75328272137153E-15));
#22825=DIRECTION('',(-0.60278101041154,-0.797906669659581,-2.75328272137153E-15));
#22826=DIRECTION('',(7.09000435319733E-16,2.91501601757459E-15,-1.));
#22827=DIRECTION('center_axis',(-0.989450675034753,-0.144870154529051,-1.12381978024773E-15));
#22828=DIRECTION('ref_axis',(7.09000435319733E-16,2.91501601757459E-15,
-1.));
#22829=DIRECTION('',(-0.144870154529051,0.989450675034753,2.78155156370036E-15));
#22830=DIRECTION('',(-0.144870154529051,0.989450675034753,2.78155156370036E-15));
#22831=DIRECTION('',(7.09000435319733E-16,2.91501601757459E-15,-1.));
#22832=DIRECTION('center_axis',(0.706250594380995,-0.707961932547571,-1.56298839434829E-15));
#22833=DIRECTION('ref_axis',(7.09000435319733E-16,2.91501601757459E-15,
-1.));
#22834=DIRECTION('',(-0.707961932547571,-0.706250594380995,-2.5606771134082E-15));
#22835=DIRECTION('',(-0.707961932547571,-0.706250594380995,-2.5606771134082E-15));
#22836=DIRECTION('',(7.09000435319733E-16,2.91501601757459E-15,-1.));
#22837=DIRECTION('center_axis',(-0.99998343772408,-0.00575536945216082,
-7.25765686799004E-16));
#22838=DIRECTION('ref_axis',(7.09000435319733E-16,2.91501601757459E-15,
-1.));
#22839=DIRECTION('',(-0.00575536945216082,0.99998343772408,2.91088717882799E-15));
#22840=DIRECTION('',(-0.00575536945216082,0.99998343772408,2.91088717882799E-15));
#22841=DIRECTION('',(7.09000435319733E-16,2.91501601757459E-15,-1.));
#22842=DIRECTION('center_axis',(0.600848154630927,-0.799363180961326,-1.90415487316725E-15));
#22843=DIRECTION('ref_axis',(7.09000435319733E-16,2.91501601757459E-15,
-1.));
#22844=DIRECTION('',(-0.799363180961326,-0.600848154630927,-2.31823083815943E-15));
#22845=DIRECTION('',(-0.799363180961326,-0.600848154630927,-2.31823083815943E-15));
#22846=DIRECTION('',(7.09000435319733E-16,2.91501601757459E-15,-1.));
#22847=DIRECTION('center_axis',(-0.991052660262409,0.133471437344482,-3.1358538980296E-16));
#22848=DIRECTION('ref_axis',(7.09000435319733E-16,2.91501601757459E-15,
-1.));
#22849=DIRECTION('',(0.133471437344482,0.991052660262409,2.98356568610482E-15));
#22850=DIRECTION('',(0.133471437344482,0.991052660262409,2.98356568610482E-15));
#22851=DIRECTION('',(7.09000435319733E-16,2.91501601757459E-15,-1.));
#22852=DIRECTION('center_axis',(0.483750889005616,-0.875205734319809,-2.20825914332409E-15));
#22853=DIRECTION('ref_axis',(7.09000435319733E-16,2.91501601757459E-15,
-1.));
#22854=DIRECTION('',(-0.875205734319809,-0.483750889005616,-2.03066283659439E-15));
#22855=DIRECTION('',(-0.875205734319809,-0.483750889005616,-2.03066283659439E-15));
#22856=DIRECTION('',(7.09000435319733E-16,2.91501601757459E-15,-1.));
#22857=DIRECTION('center_axis',(-0.962832170074423,0.270100374434723,1.04698490107504E-16));
#22858=DIRECTION('ref_axis',(0.270100374434723,0.962832170074423,2.99817248105729E-15));
#22859=DIRECTION('',(0.270100374434723,0.962832170074423,2.99817248105729E-15));
#22860=DIRECTION('',(0.270100374434723,0.962832170074423,2.99817248105729E-15));
#22861=DIRECTION('',(7.09000435319733E-16,2.91501601757459E-15,-1.));
#22862=DIRECTION('center_axis',(0.357237962584293,-0.934013403591524,-2.46938216111366E-15));
#22863=DIRECTION('ref_axis',(7.09000435319733E-16,2.91501601757459E-15,
-1.));
#22864=DIRECTION('',(-0.934013403591524,-0.357237962584293,-1.70357029275978E-15));
#22865=DIRECTION('',(-0.934013403591524,-0.357237962584293,-1.70357029275978E-15));
#22866=DIRECTION('',(7.09000435319733E-16,2.91501601757459E-15,-1.));
#22867=DIRECTION('center_axis',(-0.915871246901299,0.401472114971214,5.20944533000789E-16));
#22868=DIRECTION('ref_axis',(0.401472114971214,0.915871246901299,2.95442325903663E-15));
#22869=DIRECTION('',(0.401472114971214,0.915871246901299,2.95442325903662E-15));
#22870=DIRECTION('',(0.401472114971214,0.915871246901299,2.95442325903662E-15));
#22871=DIRECTION('',(7.09000435319733E-16,2.91501601757459E-15,-1.));
#22872=DIRECTION('center_axis',(0.223771805573421,-0.974641564386832,-2.68244146401773E-15));
#22873=DIRECTION('ref_axis',(7.09000435319733E-16,2.91501601757459E-15,
-1.));
#22874=DIRECTION('',(-0.974641564386832,-0.223771805573421,-1.34331969095908E-15));
#22875=DIRECTION('',(-0.974641564386832,-0.223771805573421,-1.34331969095908E-15));
#22876=DIRECTION('',(7.09000435319733E-16,2.91501601757459E-15,-1.));
#22877=DIRECTION('center_axis',(-0.851083931695343,0.525029657457554,9.27050983124842E-16));
#22878=DIRECTION('ref_axis',(0.525029657457554,0.851083931695343,2.85316954888546E-15));
#22879=DIRECTION('',(0.525029657457554,0.851083931695343,2.85316954888546E-15));
#22880=DIRECTION('',(0.525029657457554,0.851083931695343,2.85316954888546E-15));
#22881=DIRECTION('',(7.09000435319733E-16,2.91501601757459E-15,-1.));
#22882=DIRECTION('center_axis',(0.0859501849037209,-0.996299435769697,-2.84329009505664E-15));
#22883=DIRECTION('ref_axis',(7.09000435319733E-16,2.91501601757459E-15,
-1.));
#22884=DIRECTION('',(-0.996299435769697,-0.0859501849037209,-9.56922899377364E-16));
#22885=DIRECTION('',(-0.996299435769697,-0.0859501849037209,-9.56922899377364E-16));
#22886=DIRECTION('',(7.09000435319733E-16,2.91501601757459E-15,-1.));
#22887=DIRECTION('center_axis',(-0.769731235852561,0.638368094873866,1.31511344036723E-15));
#22888=DIRECTION('ref_axis',(0.638368094873866,0.769731235852561,2.6963821388975E-15));
#22889=DIRECTION('',(0.638368094873865,0.769731235852561,2.6963821388975E-15));
#22890=DIRECTION('',(0.638368094873865,0.769731235852561,2.6963821388975E-15));
#22891=DIRECTION('',(7.09000435319733E-16,2.91501601757459E-15,-1.));
#22892=DIRECTION('center_axis',(-0.0535443583482437,-0.998565471909116,
-2.94879731858982E-15));
#22893=DIRECTION('ref_axis',(7.09000435319733E-16,2.91501601757459E-15,
-1.));
#22894=DIRECTION('',(-0.998565471909116,0.0535443583482437,-5.51900692042934E-16));
#22895=DIRECTION('',(-0.998565471909116,0.0535443583482437,-5.51900692042934E-16));
#22896=DIRECTION('',(7.09000435319733E-16,2.91501601757459E-15,-1.));
#22897=DIRECTION('center_axis',(-0.673396597060212,0.739281423456404,1.67757871041224E-15));
#22898=DIRECTION('ref_axis',(0.739281423456404,0.673396597060212,2.48711271766512E-15));
#22899=DIRECTION('',(0.739281423456404,0.673396597060212,2.48711271766512E-15));
#22900=DIRECTION('',(0.739281423456404,0.673396597060212,2.48711271766512E-15));
#22901=DIRECTION('',(7.09000435319733E-16,2.91501601757459E-15,-1.));
#22902=DIRECTION('center_axis',(-0.191996721570762,-0.981395566989213,-2.99690955652389E-15));
#22903=DIRECTION('ref_axis',(7.09000435319733E-16,2.91501601757459E-15,
-1.));
#22904=DIRECTION('',(-0.981395566989213,0.191996721570762,-1.36136365515628E-16));
#22905=DIRECTION('',(-0.981395566989213,0.191996721570762,-1.36136365515628E-16));
#22906=DIRECTION('',(7.09000435319733E-16,2.91501601757459E-15,-1.));
#22907=DIRECTION('center_axis',(-0.563955059483364,0.825805480051516,2.00739181907657E-15));
#22908=DIRECTION('ref_axis',(0.825805480051516,0.563955059483364,2.22943447643218E-15));
#22909=DIRECTION('',(0.825805480051516,0.563955059483364,2.22943447643218E-15));
#22910=DIRECTION('',(0.825805480051516,0.563955059483364,2.22943447643218E-15));
#22911=DIRECTION('',(7.09000435319733E-16,2.91501601757459E-15,-1.));
#22912=DIRECTION('center_axis',(-0.326712087000944,-0.945123913678777,-2.98669035887431E-15));
#22913=DIRECTION('ref_axis',(7.09000435319733E-16,2.91501601757459E-15,
-1.));
#22914=DIRECTION('',(-0.945123913678776,0.326712087000944,2.82277700513634E-16));
#22915=DIRECTION('',(-0.945123913678776,0.326712087000944,2.82277700513634E-16));
#22916=DIRECTION('',(7.09000435319733E-16,2.91501601757459E-15,-1.));
#22917=DIRECTION('center_axis',(-0.443536778163045,0.896256172317238,2.29813332935693E-15));
#22918=DIRECTION('ref_axis',(0.896256172317238,0.443536778163045,1.92836282905962E-15));
#22919=DIRECTION('',(0.896256172317238,0.443536778163045,1.92836282905962E-15));
#22920=DIRECTION('',(0.896256172317238,0.443536778163045,1.92836282905962E-15));
#22921=DIRECTION('',(7.09000435319733E-16,2.91501601757459E-15,-1.));
#22922=DIRECTION('center_axis',(-0.455068373287141,-0.890456498451101,-2.91833863069917E-15));
#22923=DIRECTION('ref_axis',(7.09000435319733E-16,2.91501601757459E-15,
-1.));
#22924=DIRECTION('',(-0.890456498451101,0.455068373287141,6.95197552188514E-16));
#22925=DIRECTION('',(-0.890456498451101,0.455068373287141,6.95197552188514E-16));
#22926=DIRECTION('',(7.09000435319733E-16,2.91501601757459E-15,-1.));
#22927=DIRECTION('center_axis',(-0.314485557971386,0.949262257665091,2.54414428846928E-15));
#22928=DIRECTION('ref_axis',(0.949262257665091,0.314485557971386,1.58975779269962E-15));
#22929=DIRECTION('',(0.949262257665091,0.314485557971386,1.58975779269961E-15));
#22930=DIRECTION('',(0.949262257665091,0.314485557971386,1.58975779269961E-15));
#22931=DIRECTION('',(7.09000435319733E-16,2.91501601757459E-15,-1.));
#22932=DIRECTION('center_axis',(-0.574567271319908,-0.818457360360328,-2.79318476063846E-15));
#22933=DIRECTION('ref_axis',(7.09000435319733E-16,2.91501601757459E-15,
-1.));
#22934=DIRECTION('',(-0.818457360360328,0.574567271319907,1.09458617428554E-15));
#22935=DIRECTION('',(-0.818457360360328,0.574567271319907,1.09458617428554E-15));
#22936=DIRECTION('',(7.09000435319733E-16,2.91501601757459E-15,-1.));
#22937=DIRECTION('center_axis',(-0.179313234115836,0.983792032937307,2.7406363729278E-15));
#22938=DIRECTION('ref_axis',(0.983792032937307,0.179313234115836,1.2202099292274E-15));
#22939=DIRECTION('',(0.983792032937307,0.179313234115836,1.2202099292274E-15));
#22940=DIRECTION('',(0.983792032937307,0.179313234115836,1.2202099292274E-15));
#22941=DIRECTION('',(7.09000435319733E-16,2.91501601757459E-15,-1.));
#22942=DIRECTION('center_axis',(-0.682882870977016,-0.73052788073159,-2.6136647264125E-15));
#22943=DIRECTION('ref_axis',(7.09000435319733E-16,2.91501601757459E-15,
-1.));
#22944=DIRECTION('',(-0.73052788073159,0.682882870977016,1.47266992157342E-15));
#22945=DIRECTION('',(-0.73052788073159,0.682882870977016,1.47266992157342E-15));
#22946=DIRECTION('',(7.09000435319733E-16,2.91501601757459E-15,-1.));
#22947=DIRECTION('center_axis',(-0.0406507821240025,0.99917341533525,2.88378508781496E-15));
#22948=DIRECTION('ref_axis',(0.99917341533525,0.0406507821240025,8.26912067450998E-16));
#22949=DIRECTION('',(0.999173415335249,0.0406507821240025,8.26912067450998E-16));
#22950=DIRECTION('',(0.999173415335249,0.0406507821240025,8.26912067450998E-16));
#22951=DIRECTION('',(7.09000435319733E-16,2.91501601757459E-15,-1.));
#22952=DIRECTION('center_axis',(-0.777906932318306,-0.628379506867564,-2.38327268128649E-15));
#22953=DIRECTION('ref_axis',(7.09000435319733E-16,2.91501601757459E-15,
-1.));
#22954=DIRECTION('',(-0.628379506867564,0.777906932318306,1.82208982397507E-15));
#22955=DIRECTION('',(-0.628379506867564,0.777906932318306,1.82208982397507E-15));
#22956=DIRECTION('',(7.09000435319733E-16,2.91501601757459E-15,-1.));
#22957=DIRECTION('center_axis',(0.0988028911022945,0.995107023746606,2.97080420622471E-15));
#22958=DIRECTION('ref_axis',(0.995107023746606,-0.0988028911022945,4.17519302880201E-16));
#22959=DIRECTION('',(0.995107023746606,-0.0988028911022945,4.17519302880201E-16));
#22960=DIRECTION('',(0.995107023746606,-0.0988028911022945,4.17519302880201E-16));
#22961=DIRECTION('',(7.09000435319733E-16,2.91501601757459E-15,-1.));
#22962=DIRECTION('center_axis',(-0.857789920078043,-0.514000440673454,-2.10649294435173E-15));
#22963=DIRECTION('ref_axis',(7.09000435319733E-16,2.91501601757459E-15,
-1.));
#22964=DIRECTION('',(-0.514000440673454,0.857789920078043,2.13604482054951E-15));
#22965=DIRECTION('',(-0.514000440673454,0.857789920078043,2.13604482054951E-15));
#22966=DIRECTION('center_axis',(-7.09000435319733E-16,-2.91501601757459E-15,
1.));
#22967=DIRECTION('ref_axis',(-0.236333478439911,-0.971672005858197,-3.E-15));
#22968=DIRECTION('center_axis',(-7.09000435319733E-16,-2.91501601757459E-15,
1.));
#22969=DIRECTION('ref_axis',(-0.236333478439911,-0.971672005858197,-3.E-15));
#22970=DIRECTION('center_axis',(-7.09000435319733E-16,-2.91501601757459E-15,
1.));
#22971=DIRECTION('ref_axis',(-0.236333478439911,-0.971672005858197,-3.E-15));
#22972=DIRECTION('center_axis',(0.,0.,1.));
#22973=DIRECTION('ref_axis',(1.,0.,0.));
#22974=DIRECTION('center_axis',(0.,0.,1.));
#22975=DIRECTION('ref_axis',(1.,0.,0.));
#22976=DIRECTION('center_axis',(0.,0.,1.));
#22977=DIRECTION('ref_axis',(1.,0.,0.));
#22978=DIRECTION('center_axis',(0.,0.,1.));
#22979=DIRECTION('ref_axis',(1.,0.,0.));
#22980=DIRECTION('center_axis',(7.09000435319733E-16,2.91501601757459E-15,
-1.));
#22981=DIRECTION('ref_axis',(0.236333478439911,0.971672005858197,3.E-15));
#22982=DIRECTION('center_axis',(-7.09000435319733E-16,-2.91501601757459E-15,
1.));
#22983=DIRECTION('ref_axis',(-0.236333478439911,-0.971672005858197,-3.E-15));
#22984=DIRECTION('center_axis',(-7.09000435319733E-16,-2.91501601757459E-15,
1.));
#22985=DIRECTION('ref_axis',(-0.236333478439911,-0.971672005858197,-3.E-15));
#22986=DIRECTION('',(-7.09000435319733E-16,-2.91501601757459E-15,1.));
#22987=DIRECTION('',(0.204670796093705,0.841492641219382,-0.499999999999997));
#22988=DIRECTION('',(-0.204670796093705,-0.841492641219382,0.499999999999997));
#22989=DIRECTION('center_axis',(0.,0.,1.));
#22990=DIRECTION('ref_axis',(-0.236333478439877,-0.971672005858205,0.));
#22991=DIRECTION('',(-0.204670796093705,-0.841492641219379,-0.500000000000002));
#22992=DIRECTION('',(0.204670796093705,0.841492641219379,0.500000000000002));
#22993=DIRECTION('center_axis',(0.971672005858197,-0.236333478439911,0.));
#22994=DIRECTION('ref_axis',(-0.236333478439911,-0.971672005858197,-3.E-15));
#22995=DIRECTION('center_axis',(-0.971672005858197,0.236333478439911,0.));
#22996=DIRECTION('ref_axis',(7.09000435319733E-16,2.91501601757459E-15,
-1.));
#22997=DIRECTION('',(-7.09000435319733E-16,-2.91501601757459E-15,1.));
#22998=DIRECTION('center_axis',(-9.36335395655066E-14,2.27738783980021E-14,
1.));
#22999=DIRECTION('ref_axis',(-0.236333478439913,-0.971672005858196,0.));
#23000=DIRECTION('center_axis',(-7.09000435319733E-16,-2.91501601757459E-15,
1.));
#23001=DIRECTION('ref_axis',(-0.236333478439908,-0.971672005858198,-3.E-15));
#23002=DIRECTION('center_axis',(-9.36335395655066E-14,2.27738783980021E-14,
1.));
#23003=DIRECTION('ref_axis',(0.999921424989944,-0.0125357028554228,9.39116688816566E-14));
#23004=DIRECTION('center_axis',(7.09000435319733E-16,2.91501601757459E-15,
-1.));
#23005=DIRECTION('ref_axis',(-0.236333478439908,-0.971672005858198,-3.E-15));
#23006=DIRECTION('center_axis',(-7.09000435319733E-16,-2.91501601757459E-15,
1.));
#23007=DIRECTION('ref_axis',(-0.236333478439908,-0.971672005858198,-3.E-15));
#23008=DIRECTION('',(0.167113005226264,0.687075864431466,0.707106781186548));
#23009=DIRECTION('center_axis',(7.09000435319733E-16,2.91501601757459E-15,
-1.));
#23010=DIRECTION('ref_axis',(-0.236333478439911,-0.971672005858197,-3.E-15));
#23011=DIRECTION('center_axis',(7.09000435319733E-16,2.91501601757459E-15,
-1.));
#23012=DIRECTION('ref_axis',(0.236333478439911,0.971672005858197,3.E-15));
#23013=DIRECTION('',(-0.167113005226266,-0.687075864431464,-0.707106781186549));
#23014=DIRECTION('center_axis',(-7.09000435319733E-16,-2.91501601757459E-15,
1.));
#23015=DIRECTION('ref_axis',(-0.236333478439911,-0.971672005858197,-3.E-15));
#23016=DIRECTION('center_axis',(-7.09000435319733E-16,-2.91501601757459E-15,
1.));
#23017=DIRECTION('ref_axis',(-0.236333478439911,-0.971672005858197,-3.E-15));
#23018=DIRECTION('',(-0.167113005226266,-0.687075864431467,-0.707106781186547));
#23019=DIRECTION('center_axis',(7.09000435319733E-16,2.91501601757459E-15,
-1.));
#23020=DIRECTION('ref_axis',(-0.23633347843991,-0.971672005858197,-3.E-15));
#23021=DIRECTION('center_axis',(7.09000435319733E-16,2.91501601757459E-15,
-1.));
#23022=DIRECTION('ref_axis',(0.23633347843991,0.971672005858197,3.E-15));
#23023=DIRECTION('center_axis',(7.09000435319733E-16,2.91501601757459E-15,
-1.));
#23024=DIRECTION('ref_axis',(-0.236333478439911,-0.971672005858197,-3.E-15));
#23025=DIRECTION('',(0.167113005226265,0.687075864431463,0.70710678118655));
#23026=DIRECTION('center_axis',(-7.09000435319733E-16,-2.91501601757459E-15,
1.));
#23027=DIRECTION('ref_axis',(-0.23633347843991,-0.971672005858197,-3.E-15));
#23028=DIRECTION('center_axis',(7.09000435319733E-16,2.91501601757459E-15,
-1.));
#23029=DIRECTION('ref_axis',(0.236333478439911,0.971672005858197,3.E-15));
#23030=DIRECTION('',(-7.09000435319733E-16,-2.91501601757459E-15,1.));
#23031=DIRECTION('center_axis',(-7.09000435319733E-16,-2.91501601757459E-15,
1.));
#23032=DIRECTION('ref_axis',(-0.236333478439911,-0.971672005858197,-3.E-15));
#23033=DIRECTION('center_axis',(-7.09000435319733E-16,-2.91501601757459E-15,
1.));
#23034=DIRECTION('ref_axis',(-0.236333478439911,-0.971672005858197,-3.E-15));
#23035=DIRECTION('center_axis',(7.09000435319733E-16,2.91501601757459E-15,
-1.));
#23036=DIRECTION('ref_axis',(0.236333478439908,0.971672005858198,3.E-15));
#27554=CARTESIAN_POINT('',(0.,0.,0.));
#27555=CARTESIAN_POINT('Origin',(77.215862801455,80.368869783441,212.));
#27556=CARTESIAN_POINT('',(76.8377292359511,78.8141945740679,198.4));
#27557=CARTESIAN_POINT('',(76.8377292359511,78.8141945740679,198.312499998088));
#27558=CARTESIAN_POINT('',(76.8377292359511,78.8141945740678,212.));
#27559=CARTESIAN_POINT('',(76.8377292359511,78.8141945740679,198.1));
#27560=CARTESIAN_POINT('',(76.8377292359511,78.8141945740679,198.006249999044));
#27561=CARTESIAN_POINT('',(76.8768229089103,81.9325359726461,198.1));
#27562=CARTESIAN_POINT('Origin',(77.215862801455,80.368869783441,198.1));
#27563=CARTESIAN_POINT('Ctrl Pts',(76.8377292359512,78.8141945740679,198.4));
#27564=CARTESIAN_POINT('Ctrl Pts',(76.8306919936837,78.8159061968518,198.399542658881));
#27565=CARTESIAN_POINT('Ctrl Pts',(76.8236645970994,78.8176660326881,198.399083409546));
#27566=CARTESIAN_POINT('Ctrl Pts',(76.6110740000279,78.8724418439445,198.385112914876));
#27567=CARTESIAN_POINT('Ctrl Pts',(76.4181464081622,78.9657791947612,198.370237944061));
#27568=CARTESIAN_POINT('Ctrl Pts',(76.0829345406545,79.2199759547389,198.339759359453));
#27569=CARTESIAN_POINT('Ctrl Pts',(75.9429889506103,79.3772603708408,198.324459092766));
#27570=CARTESIAN_POINT('Ctrl Pts',(75.7339714702803,79.7321991446286,198.295564011952));
#27571=CARTESIAN_POINT('Ctrl Pts',(75.6651563328787,79.9254175659732,198.283141851207));
#27572=CARTESIAN_POINT('Ctrl Pts',(75.6018680703669,80.3382054162985,198.254986009091));
#27573=CARTESIAN_POINT('Ctrl Pts',(75.6122792966977,80.5543572171928,198.239492006727));
#27574=CARTESIAN_POINT('Ctrl Pts',(75.7155422448449,80.9617434362757,198.208848757408));
#27575=CARTESIAN_POINT('Ctrl Pts',(75.8042954983089,81.1498759107796,198.193989913992));
#27576=CARTESIAN_POINT('Ctrl Pts',(76.038522207399,81.4687760552142,198.167359146374));
#27577=CARTESIAN_POINT('Ctrl Pts',(76.1769316856716,81.6003554294599,198.155785245017));
#27578=CARTESIAN_POINT('Ctrl Pts',(76.5001429204423,81.8134379281221,198.128799947654));
#27579=CARTESIAN_POINT('Ctrl Pts',(76.6837837988249,81.8906805180791,198.114366048253));
#27580=CARTESIAN_POINT('Ctrl Pts',(76.8768229089103,81.9325359726461,198.1));
#27581=CARTESIAN_POINT('Origin',(77.215862801455,80.368869783441,212.));
#27582=CARTESIAN_POINT('',(76.8377292359509,78.8141945740679,199.1));
#27583=CARTESIAN_POINT('',(76.8377292359516,78.8141945740678,199.012499998088));
#27584=CARTESIAN_POINT('',(76.8377292359511,78.8141945740678,212.));
#27585=CARTESIAN_POINT('Ctrl Pts',(76.8377292359511,78.8141945740679,198.312499998088));
#27586=CARTESIAN_POINT('Ctrl Pts',(76.9720481847989,78.7815250475093,198.321229209914));
#27587=CARTESIAN_POINT('Ctrl Pts',(77.1100034492629,78.7664077184876,198.330572722172));
#27588=CARTESIAN_POINT('Ctrl Pts',(77.3912490807052,78.772083398796,198.350369291815));
#27589=CARTESIAN_POINT('Ctrl Pts',(77.5333074426643,78.7941606892817,198.360762469305));
#27590=CARTESIAN_POINT('Ctrl Pts',(77.8761650962969,78.8957753239252,198.386837255165));
#27591=CARTESIAN_POINT('Ctrl Pts',(78.0675144740926,78.997472028618,198.402311907275));
#27592=CARTESIAN_POINT('Ctrl Pts',(78.3899087615022,79.2630351083584,198.430315976051));
#27593=CARTESIAN_POINT('Ctrl Pts',(78.5206414445282,79.4208075667966,198.442813555558));
#27594=CARTESIAN_POINT('Ctrl Pts',(78.7189000424947,79.7819394290783,198.471816660304));
#27595=CARTESIAN_POINT('Ctrl Pts',(78.7825859666829,79.982896651337,198.487152174499));
#27596=CARTESIAN_POINT('Ctrl Pts',(78.8295412717651,80.4012094693317,198.517599255318));
#27597=CARTESIAN_POINT('Ctrl Pts',(78.8110498611063,80.6147063508936,198.532407084758));
#27598=CARTESIAN_POINT('Ctrl Pts',(78.6942808378984,81.0135564815686,198.558653809128));
#27599=CARTESIAN_POINT('Ctrl Pts',(78.600431543102,81.1961693227667,198.572795109126));
#27600=CARTESIAN_POINT('Ctrl Pts',(78.3443394345243,81.5226463654582,198.602739991542));
#27601=CARTESIAN_POINT('Ctrl Pts',(78.1822431448,81.6614556920644,198.618278331139));
#27602=CARTESIAN_POINT('Ctrl Pts',(77.8161878865673,81.8665246944038,198.647910117927));
#27603=CARTESIAN_POINT('Ctrl Pts',(77.6164722828377,81.9318335405764,198.660757313471));
#27604=CARTESIAN_POINT('Ctrl Pts',(77.2054327727601,81.9820302740299,198.688490755413));
#27605=CARTESIAN_POINT('Ctrl Pts',(76.9981836939206,81.9672995861781,198.703295046626));
#27606=CARTESIAN_POINT('Ctrl Pts',(76.5928838188948,81.8580539426185,198.733895685235));
#27607=CARTESIAN_POINT('Ctrl Pts',(76.3995268294322,81.7614929603439,198.749405529619));
#27608=CARTESIAN_POINT('Ctrl Pts',(76.0704528171171,81.5044202670635,198.777702946476));
#27609=CARTESIAN_POINT('Ctrl Pts',(75.9354522947806,81.349683608691,198.790073141041));
#27610=CARTESIAN_POINT('Ctrl Pts',(75.7282528365861,80.993697573892,198.818865733043));
#27611=CARTESIAN_POINT('Ctrl Pts',(75.6596351655703,80.7949368475463,198.834130610186));
#27612=CARTESIAN_POINT('Ctrl Pts',(75.6018825845919,80.3784602743984,198.864633656738));
#27613=CARTESIAN_POINT('Ctrl Pts',(75.6148283713537,80.1645110358893,198.879569101951));
#27614=CARTESIAN_POINT('Ctrl Pts',(75.7211303911452,79.7630956612239,198.906177950839));
#27615=CARTESIAN_POINT('Ctrl Pts',(75.8099594347692,79.5784884263048,198.919811057053));
#27616=CARTESIAN_POINT('Ctrl Pts',(76.0566259187301,79.2461087993588,198.949556000229));
#27617=CARTESIAN_POINT('Ctrl Pts',(76.2144478184568,79.1033283836519,198.965068839922));
#27618=CARTESIAN_POINT('Ctrl Pts',(76.5332172535871,78.9129289906697,198.991468046714));
#27619=CARTESIAN_POINT('Ctrl Pts',(76.6823153024518,78.8519948968934,199.002399850954));
#27620=CARTESIAN_POINT('Ctrl Pts',(76.837729235952,78.8141945740677,199.012499998088));
#27621=CARTESIAN_POINT('Ctrl Pts',(76.8377292359507,78.814194574068,199.1));
#27622=CARTESIAN_POINT('Ctrl Pts',(76.803254858159,78.822579553332,199.097759555529));
#27623=CARTESIAN_POINT('Ctrl Pts',(76.7690280068441,78.8321188092932,199.095474049025));
#27624=CARTESIAN_POINT('Ctrl Pts',(76.532562538695,78.9066126046754,199.079251543903));
#27625=CARTESIAN_POINT('Ctrl Pts',(76.3447869226595,79.0100914642844,199.064137681813));
#27626=CARTESIAN_POINT('Ctrl Pts',(76.024305592285,79.2811061032762,199.033589251734));
#27627=CARTESIAN_POINT('Ctrl Pts',(75.8934314734524,79.4446211161594,199.018453730095));
#27628=CARTESIAN_POINT('Ctrl Pts',(75.7027394696539,79.8100007830423,198.989999487709));
#27629=CARTESIAN_POINT('Ctrl Pts',(75.6437512894612,80.0078414436886,198.977670895753));
#27630=CARTESIAN_POINT('Ctrl Pts',(75.6026562880355,80.423595255991,198.948922463328));
#27631=CARTESIAN_POINT('Ctrl Pts',(75.6242867916757,80.6377408622658,198.933377264154));
#27632=CARTESIAN_POINT('Ctrl Pts',(75.7477523210465,81.0372197979956,198.902946110429));
#27633=CARTESIAN_POINT('Ctrl Pts',(75.8454052288813,81.219707520826,198.888333839163));
#27634=CARTESIAN_POINT('Ctrl Pts',(76.1078081931828,81.5421385341799,198.860967354125));
#27635=CARTESIAN_POINT('Ctrl Pts',(76.2716666646728,81.6776381830664,198.847571727011));
#27636=CARTESIAN_POINT('Ctrl Pts',(76.6424477897895,81.8773440853991,198.817531960833));
#27637=CARTESIAN_POINT('Ctrl Pts',(76.8456364090363,81.939611578871,198.802037218959));
#27638=CARTESIAN_POINT('Ctrl Pts',(77.2569926218215,81.9811692267037,198.772400501348));
#27639=CARTESIAN_POINT('Ctrl Pts',(77.4608895405315,81.9629520640054,198.759004513137));
#27640=CARTESIAN_POINT('Ctrl Pts',(77.8600269118437,81.8487800120576,198.732204504379));
#27641=CARTESIAN_POINT('Ctrl Pts',(78.0504551467755,81.7503507672924,198.71720498185));
#27642=CARTESIAN_POINT('Ctrl Pts',(78.3784297681607,81.4876632826046,198.686680604441));
#27643=CARTESIAN_POINT('Ctrl Pts',(78.5138862290576,81.3272088530237,198.671457497262));
#27644=CARTESIAN_POINT('Ctrl Pts',(78.7137859745099,80.9670331217066,198.642779630751));
#27645=CARTESIAN_POINT('Ctrl Pts',(78.7777254334594,80.7715523859113,198.630445530054));
#27646=CARTESIAN_POINT('Ctrl Pts',(78.8300314602077,80.3572395924842,198.601992391047));
#27647=CARTESIAN_POINT('Ctrl Pts',(78.8140435325791,80.1420106726523,198.586467674468));
#27648=CARTESIAN_POINT('Ctrl Pts',(78.7007132113641,79.7384164908133,198.555919607586));
#27649=CARTESIAN_POINT('Ctrl Pts',(78.6075117625974,79.5530263026121,198.541178403936));
#27650=CARTESIAN_POINT('Ctrl Pts',(78.353950676021,79.2250085562103,198.513568461787));
#27651=CARTESIAN_POINT('Ctrl Pts',(78.1950310205265,79.0863276432054,198.500556585232));
#27652=CARTESIAN_POINT('Ctrl Pts',(77.8309453443636,78.8768184961485,198.470784351695));
#27653=CARTESIAN_POINT('Ctrl Pts',(77.6289911909212,78.808785940305,198.455257798593));
#27654=CARTESIAN_POINT('Ctrl Pts',(77.2251848651683,78.7569260165313,198.425938172113));
#27655=CARTESIAN_POINT('Ctrl Pts',(77.0279400750016,78.7679308256438,198.41236155226));
#27656=CARTESIAN_POINT('Ctrl Pts',(76.8377292359511,78.8141945740679,198.4));
#27657=CARTESIAN_POINT('Origin',(77.215862801455,80.368869783441,212.));
#27658=CARTESIAN_POINT('',(76.8377292359509,78.8141945740679,199.8));
#27659=CARTESIAN_POINT('',(76.8377292359513,78.8141945740678,199.712499998088));
#27660=CARTESIAN_POINT('',(76.8377292359511,78.8141945740678,212.));
#27661=CARTESIAN_POINT('Ctrl Pts',(76.837729235952,78.8141945740677,199.012499998088));
#27662=CARTESIAN_POINT('Ctrl Pts',(76.8854116654775,78.8025970860652,199.01559881647));
#27663=CARTESIAN_POINT('Ctrl Pts',(76.9336787715119,78.793180648293,199.01878326277));
#27664=CARTESIAN_POINT('Ctrl Pts',(77.1855842440625,78.756024231363,199.035648622212));
#27665=CARTESIAN_POINT('Ctrl Pts',(77.3926167754525,78.7654644547276,199.050329297338));
#27666=CARTESIAN_POINT('Ctrl Pts',(77.7995590980122,78.8639346257316,199.080823951734));
#27667=CARTESIAN_POINT('Ctrl Pts',(77.9948655479242,78.9551114350834,199.096359825612));
#27668=CARTESIAN_POINT('Ctrl Pts',(78.3308066382515,79.203277166845,199.124955160147));
#27669=CARTESIAN_POINT('Ctrl Pts',(78.4702842926093,79.3548996297549,199.137276119643));
#27670=CARTESIAN_POINT('Ctrl Pts',(78.6866319321173,79.7055359348698,199.165847324901));
#27671=CARTESIAN_POINT('Ctrl Pts',(78.7602426169992,79.9019169960723,199.181029643047));
#27672=CARTESIAN_POINT('Ctrl Pts',(78.8290181862994,80.3162153276788,199.21156831412));
#27673=CARTESIAN_POINT('Ctrl Pts',(78.8217807425611,80.530474385319,199.226624080228));
#27674=CARTESIAN_POINT('Ctrl Pts',(78.726245797459,80.9344243060637,199.253598049677));
#27675=CARTESIAN_POINT('Ctrl Pts',(78.6424980783076,81.1211153781538,199.266797489178));
#27676=CARTESIAN_POINT('Ctrl Pts',(78.4053938550654,81.4593741057634,199.296334104196));
#27677=CARTESIAN_POINT('Ctrl Pts',(78.2519971062266,81.6060477692569,199.311809573208));
#27678=CARTESIAN_POINT('Ctrl Pts',(77.8961673620155,81.8324027003303,199.341973775574));
#27679=CARTESIAN_POINT('Ctrl Pts',(77.6970230333772,81.9093834757634,199.355581024474));
#27680=CARTESIAN_POINT('Ctrl Pts',(77.2868111534351,81.9803742875688,199.382830240369));
#27681=CARTESIAN_POINT('Ctrl Pts',(77.0801287919668,81.9762018850526,199.397378413386));
#27682=CARTESIAN_POINT('Ctrl Pts',(76.6718245501323,81.8885129175043,199.427747336064));
#27683=CARTESIAN_POINT('Ctrl Pts',(76.4747143841974,81.8027505106219,199.44329842119));
#27684=CARTESIAN_POINT('Ctrl Pts',(76.1319973254571,81.5635600273011,199.472183898001));
#27685=CARTESIAN_POINT('Ctrl Pts',(75.9880079185057,81.4150152807634,199.484538648629));
#27686=CARTESIAN_POINT('Ctrl Pts',(75.7626694496214,81.069717485316,199.512886550503));
#27687=CARTESIAN_POINT('Ctrl Pts',(75.6842121064397,80.8758026150676,199.527977657111));
#27688=CARTESIAN_POINT('Ctrl Pts',(75.6046455222828,80.4639390682683,199.558529778817));
#27689=CARTESIAN_POINT('Ctrl Pts',(75.6062483704505,80.2495284388588,199.57369338296));
#27690=CARTESIAN_POINT('Ctrl Pts',(75.6911465663229,79.8431810619917,199.601020514144));
#27691=CARTESIAN_POINT('Ctrl Pts',(75.7699483324182,79.6543955980109,199.613878886283));
#27692=CARTESIAN_POINT('Ctrl Pts',(75.997737645633,79.3105102645591,199.643207506063));
#27693=CARTESIAN_POINT('Ctrl Pts',(76.1467436708089,79.1601790240112,199.658635554281));
#27694=CARTESIAN_POINT('Ctrl Pts',(76.4781611250778,78.9363914345893,199.68738292686));
#27695=CARTESIAN_POINT('Ctrl Pts',(76.6533187883288,78.8590475309139,199.700515405639));
#27696=CARTESIAN_POINT('Ctrl Pts',(76.8377292359514,78.8141945740678,199.712499998088));
#27697=CARTESIAN_POINT('Ctrl Pts',(76.8377292359506,78.814194574068,199.8));
#27698=CARTESIAN_POINT('Ctrl Pts',(76.7776741872748,78.8288013739613,199.796097101373));
#27699=CARTESIAN_POINT('Ctrl Pts',(76.7184087914351,78.8469012544151,199.792059976321));
#27700=CARTESIAN_POINT('Ctrl Pts',(76.4610472853451,78.9422062861736,199.773687527242));
#27701=CARTESIAN_POINT('Ctrl Pts',(76.2785728993196,79.054880815752,199.758390268385));
#27702=CARTESIAN_POINT('Ctrl Pts',(75.9725918263895,79.3408108169731,199.727855637987));
#27703=CARTESIAN_POINT('Ctrl Pts',(75.8504158980802,79.5096772799917,199.712909438187));
#27704=CARTESIAN_POINT('Ctrl Pts',(75.676982149273,79.8846035228494,199.684884774663));
#27705=CARTESIAN_POINT('Ctrl Pts',(75.6273887810091,80.0870447359082,199.672341226034));
#27706=CARTESIAN_POINT('Ctrl Pts',(75.6076404521229,80.5052218226292,199.643053242266));
#27707=CARTESIAN_POINT('Ctrl Pts',(75.6398499221955,80.7169201980688,199.627499128428));
#27708=CARTESIAN_POINT('Ctrl Pts',(75.7821746261454,81.1079086270507,199.597344542763));
#27709=CARTESIAN_POINT('Ctrl Pts',(75.8880358148982,81.2845991936081,199.583001555874));
#27710=CARTESIAN_POINT('Ctrl Pts',(76.1672426335115,81.596175520434,199.556114562209));
#27711=CARTESIAN_POINT('Ctrl Pts',(76.3408411165774,81.7254472456341,199.541751069757));
#27712=CARTESIAN_POINT('Ctrl Pts',(76.7242979855457,81.9058138191048,199.511220804094));
#27713=CARTESIAN_POINT('Ctrl Pts',(76.9294188839191,81.956884191104,199.495820409909));
#27714=CARTESIAN_POINT('Ctrl Pts',(77.3412033851244,81.9768040425828,199.466597332834));
#27715=CARTESIAN_POINT('Ctrl Pts',(77.5437899955011,81.947983517883,199.45387847663));
#27716=CARTESIAN_POINT('Ctrl Pts',(77.9364767053395,81.8131073340246,199.426376250234));
#27717=CARTESIAN_POINT('Ctrl Pts',(78.1215613870327,81.704825229225,199.411162474011));
#27718=CARTESIAN_POINT('Ctrl Pts',(78.4346104381944,81.425978658953,199.380611707556));
#27719=CARTESIAN_POINT('Ctrl Pts',(78.560999860468,81.2596317542165,199.365570135878));
#27720=CARTESIAN_POINT('Ctrl Pts',(78.742763478423,80.8892780219466,199.337336357528));
#27721=CARTESIAN_POINT('Ctrl Pts',(78.7969110191719,80.6890886408464,199.324933502818));
#27722=CARTESIAN_POINT('Ctrl Pts',(78.8270160600529,80.2720320582584,199.295903381569));
#27723=CARTESIAN_POINT('Ctrl Pts',(78.7999100530586,80.0590843417189,199.280348696751));
#27724=CARTESIAN_POINT('Ctrl Pts',(78.6666596808023,79.6638718993203,199.250051209934));
#27725=CARTESIAN_POINT('Ctrl Pts',(78.5647355517841,79.4843259782325,199.235573764053));
#27726=CARTESIAN_POINT('Ctrl Pts',(78.2936759395128,79.1674473164975,199.208451492165));
#27727=CARTESIAN_POINT('Ctrl Pts',(78.1248579471808,79.0351226849919,199.194596427885));
#27728=CARTESIAN_POINT('Ctrl Pts',(77.7475358028786,78.8452611117838,199.164300777613));
#27729=CARTESIAN_POINT('Ctrl Pts',(77.5432819887802,78.7887246013366,199.148848993046));
#27730=CARTESIAN_POINT('Ctrl Pts',(77.1671515670854,78.7608898413889,199.12195854748));
#27731=CARTESIAN_POINT('Ctrl Pts',(76.9997653690582,78.7747835765921,199.110530515177));
#27732=CARTESIAN_POINT('Ctrl Pts',(76.8377292359507,78.814194574068,199.1));
#27733=CARTESIAN_POINT('Origin',(77.215862801455,80.368869783441,212.));
#27734=CARTESIAN_POINT('',(76.8377292359511,78.8141945740679,200.5));
#27735=CARTESIAN_POINT('',(76.8377292359511,78.8141945740679,200.412499998088));
#27736=CARTESIAN_POINT('',(76.8377292359511,78.8141945740678,212.));
#27737=CARTESIAN_POINT('Ctrl Pts',(76.8377292359514,78.8141945740678,199.712499998088));
#27738=CARTESIAN_POINT('Ctrl Pts',(76.8601595856551,78.8087389856222,199.713957717014));
#27739=CARTESIAN_POINT('Ctrl Pts',(76.8827246653436,78.8037647658874,199.715434732537));
#27740=CARTESIAN_POINT('Ctrl Pts',(77.1059319935505,78.7596160590715,199.730148581308));
#27741=CARTESIAN_POINT('Ctrl Pts',(77.3121533169625,78.7587557394075,199.744561314105));
#27742=CARTESIAN_POINT('Ctrl Pts',(77.7215015090649,78.8360958232994,199.774791118394));
#27743=CARTESIAN_POINT('Ctrl Pts',(77.920205761451,78.9166352832053,199.790346671055));
#27744=CARTESIAN_POINT('Ctrl Pts',(78.2693460365696,79.1471396865218,199.819503534684));
#27745=CARTESIAN_POINT('Ctrl Pts',(78.4176997359322,79.2927498245599,199.831966567357));
#27746=CARTESIAN_POINT('Ctrl Pts',(78.6515343010296,79.6329329489428,199.86009849949));
#27747=CARTESIAN_POINT('Ctrl Pts',(78.7345089081834,79.8244045688921,199.875094343593));
#27748=CARTESIAN_POINT('Ctrl Pts',(78.8242168733294,80.2337018624852,199.905639406342));
#27749=CARTESIAN_POINT('Ctrl Pts',(78.8279518622446,80.4481151143427,199.920895181364));
#27750=CARTESIAN_POINT('Ctrl Pts',(78.7531522647425,80.8566382418602,199.948550492446));
#27751=CARTESIAN_POINT('Ctrl Pts',(78.6789862693489,81.0474474543987,199.961163870517));
#27752=CARTESIAN_POINT('Ctrl Pts',(78.459921675685,81.3965165483435,199.990293326169));
#27753=CARTESIAN_POINT('Ctrl Pts',(78.3150937441767,81.5501499381234,200.005667272635));
#27754=CARTESIAN_POINT('Ctrl Pts',(77.9719250383511,81.7948674721432,200.036088247044));
#27755=CARTESIAN_POINT('Ctrl Pts',(77.7762937142079,81.8824471403564,200.050586284423));
#27756=CARTESIAN_POINT('Ctrl Pts',(77.3705955233945,81.9743643288998,200.077090629358));
#27757=CARTESIAN_POINT('Ctrl Pts',(77.1650557512591,81.9809886005648,200.091337500084));
#27758=CARTESIAN_POINT('Ctrl Pts',(76.7548241561411,81.9155604084609,200.121384907449));
#27759=CARTESIAN_POINT('Ctrl Pts',(76.5544508890402,81.8410637828125,200.136933361737));
#27760=CARTESIAN_POINT('Ctrl Pts',(76.1980154936663,81.6206631837517,200.166393558143));
#27761=CARTESIAN_POINT('Ctrl Pts',(76.044579685092,81.4784120954065,200.179072034181));
#27762=CARTESIAN_POINT('Ctrl Pts',(75.8011131179273,81.1441180710667,200.20695270211));
#27763=CARTESIAN_POINT('Ctrl Pts',(75.7130966242145,80.9555460879553,200.221829988864));
#27764=CARTESIAN_POINT('Ctrl Pts',(75.6114955338623,80.5475615615859,200.252486990691));
#27765=CARTESIAN_POINT('Ctrl Pts',(75.6020022505719,80.3312717497537,200.267974952688));
#27766=CARTESIAN_POINT('Ctrl Pts',(75.6670900122648,79.9187442358169,200.29608133955));
#27767=CARTESIAN_POINT('Ctrl Pts',(75.7367070491808,79.7258918308971,200.308525861151));
#27768=CARTESIAN_POINT('Ctrl Pts',(75.9472279372274,79.3718247070364,200.337456348369));
#27769=CARTESIAN_POINT('Ctrl Pts',(76.0879086041414,79.2150761562445,200.352768404332));
#27770=CARTESIAN_POINT('Ctrl Pts',(76.4242954096651,78.9623022207994,200.383237319686));
#27771=CARTESIAN_POINT('Ctrl Pts',(76.6176225724446,78.8698127731646,200.398090673413));
#27772=CARTESIAN_POINT('Ctrl Pts',(76.8281845736508,78.8165393565164,200.41187853009));
#27773=CARTESIAN_POINT('Ctrl Pts',(76.8329546462495,78.8153558665467,200.412189703783));
#27774=CARTESIAN_POINT('Ctrl Pts',(76.8377292359511,78.8141945740679,200.412499998088));
#27775=CARTESIAN_POINT('Ctrl Pts',(76.8377292359511,78.8141945740679,200.5));
#27776=CARTESIAN_POINT('Ctrl Pts',(76.7505355862406,78.8354021198341,200.494333399385));
#27777=CARTESIAN_POINT('Ctrl Pts',(76.6651008066216,78.8639490172179,200.488390033652));
#27778=CARTESIAN_POINT('Ctrl Pts',(76.3862547297379,78.9841881185334,200.467629017513));
#27779=CARTESIAN_POINT('Ctrl Pts',(76.2091073795797,79.1071214080758,200.452096196954));
#27780=CARTESIAN_POINT('Ctrl Pts',(75.919134425438,79.4093510209623,200.421585198431));
#27781=CARTESIAN_POINT('Ctrl Pts',(75.8067701191103,79.5835831991175,200.40688632741));
#27782=CARTESIAN_POINT('Ctrl Pts',(75.6525829641113,79.9688219410575,200.379357548924));
#27783=CARTESIAN_POINT('Ctrl Pts',(75.6136850892892,80.1766846348362,200.366226292963));
#27784=CARTESIAN_POINT('Ctrl Pts',(75.6182428396301,80.5970629377492,200.336363492498));
#27785=CARTESIAN_POINT('Ctrl Pts',(75.6621865959909,80.8053862221654,200.320846294675));
#27786=CARTESIAN_POINT('Ctrl Pts',(75.8252971031959,81.1859474327836,200.29107229427));
#27787=CARTESIAN_POINT('Ctrl Pts',(75.9401458805879,81.3556580291316,200.277371065842));
#27788=CARTESIAN_POINT('Ctrl Pts',(76.233558924232,81.6495534276981,200.250814105619));
#27789=CARTESIAN_POINT('Ctrl Pts',(76.4119220403041,81.7684056311527,200.235896453611));
#27790=CARTESIAN_POINT('Ctrl Pts',(76.8009446034018,81.9281170529271,200.205400191864));
#27791=CARTESIAN_POINT('Ctrl Pts',(77.0073123858077,81.9688481803144,200.19012451813));
#27792=CARTESIAN_POINT('Ctrl Pts',(77.4192074068678,81.968890864281,200.161301221737));
#27793=CARTESIAN_POINT('Ctrl Pts',(77.6207820272753,81.9301026773435,200.14891743278));
#27794=CARTESIAN_POINT('Ctrl Pts',(78.0085391862507,81.7751067411898,200.120662184743));
#27795=CARTESIAN_POINT('Ctrl Pts',(78.1893481759911,81.6565546605442,200.105156831585));
#27796=CARTESIAN_POINT('Ctrl Pts',(78.4877824315008,81.3611459774882,200.074542992852));
#27797=CARTESIAN_POINT('Ctrl Pts',(78.6048141413239,81.1893810893234,200.059722177943));
#27798=CARTESIAN_POINT('Ctrl Pts',(78.7681363382764,80.8089933634251,200.031955840391));
#27799=CARTESIAN_POINT('Ctrl Pts',(78.8121438676005,80.603740298022,200.019148982569));
#27800=CARTESIAN_POINT('Ctrl Pts',(78.8191876057905,80.1843363761557,199.989555142443));
#27801=CARTESIAN_POINT('Ctrl Pts',(78.7807999465509,79.9743261369516,199.974014168319));
#27802=CARTESIAN_POINT('Ctrl Pts',(78.6275505276573,79.588778510458,199.944056807623));
#27803=CARTESIAN_POINT('Ctrl Pts',(78.5169813912986,79.4156945765352,199.929888224154));
#27804=CARTESIAN_POINT('Ctrl Pts',(78.2309703296968,79.114066650814,199.903588830355));
#27805=CARTESIAN_POINT('Ctrl Pts',(78.0557946210714,78.9906074099691,199.888851074689));
#27806=CARTESIAN_POINT('Ctrl Pts',(77.6703909382835,78.8206350131503,199.858397677972));
#27807=CARTESIAN_POINT('Ctrl Pts',(77.4646014622763,78.7745778735927,199.843053279394));
#27808=CARTESIAN_POINT('Ctrl Pts',(77.1147609741259,78.7658493783967,199.818394185781));
#27809=CARTESIAN_POINT('Ctrl Pts',(76.9742473029973,78.7809901702562,199.808872129625));
#27810=CARTESIAN_POINT('Ctrl Pts',(76.8377292359505,78.814194574068,199.8));
#27811=CARTESIAN_POINT('Origin',(77.215862801455,80.368869783441,212.));
#27812=CARTESIAN_POINT('',(76.8377292359512,78.8141945740679,201.2));
#27813=CARTESIAN_POINT('',(76.8377292359509,78.8141945740679,201.112499998088));
#27814=CARTESIAN_POINT('',(76.8377292359511,78.8141945740678,212.));
#27815=CARTESIAN_POINT('Ctrl Pts',(76.8377292359511,78.8141945740679,200.412499998088));
#27816=CARTESIAN_POINT('Ctrl Pts',(77.0302999172219,78.7673568565296,200.42501491339));
#27817=CARTESIAN_POINT('Ctrl Pts',(77.2300555439046,78.7566661871331,200.438773669814));
#27818=CARTESIAN_POINT('Ctrl Pts',(77.6361104560006,78.8106757494655,200.468294712584));
#27819=CARTESIAN_POINT('Ctrl Pts',(77.8378433339808,78.8796670859991,200.483825438466));
#27820=CARTESIAN_POINT('Ctrl Pts',(78.2008039851846,79.0907979449742,200.513552195936));
#27821=CARTESIAN_POINT('Ctrl Pts',(78.3589068259797,79.2300077242772,200.526508063946));
#27822=CARTESIAN_POINT('Ctrl Pts',(78.6109832588704,79.5589553219541,200.554158302549));
#27823=CARTESIAN_POINT('Ctrl Pts',(78.703428825977,79.7448224249829,200.568920270287));
#27824=CARTESIAN_POINT('Ctrl Pts',(78.8150442280174,80.1490831036783,200.599486006593));
#27825=CARTESIAN_POINT('Ctrl Pts',(78.8300802458321,80.3644798764053,200.615006211804));
#27826=CARTESIAN_POINT('Ctrl Pts',(78.7758931794791,80.778539343366,200.643408987059));
#27827=CARTESIAN_POINT('Ctrl Pts',(78.7111206404444,80.9736291058694,200.655752309459));
#27828=CARTESIAN_POINT('Ctrl Pts',(78.5096661593118,81.332917790401,200.684467514317));
#27829=CARTESIAN_POINT('Ctrl Pts',(78.3734406131165,81.4928414257531,200.699704459788));
#27830=CARTESIAN_POINT('Ctrl Pts',(78.0442186723007,81.7540980926201,200.730222583063));
#27831=CARTESIAN_POINT('Ctrl Pts',(77.8533551387306,81.8516653507143,200.745201663778));
#27832=CARTESIAN_POINT('Ctrl Pts',(77.4536802563094,81.9640479505271,200.771939924285));
#27833=CARTESIAN_POINT('Ctrl Pts',(77.2496582900372,81.9813454348773,200.785410107944));
#27834=CARTESIAN_POINT('Ctrl Pts',(76.8383554720865,81.9378904779783,200.815081987171));
#27835=CARTESIAN_POINT('Ctrl Pts',(76.6353644890328,81.8746461163417,200.83058292681));
#27836=CARTESIAN_POINT('Ctrl Pts',(76.2657096289213,81.6732724609816,200.860578074065));
#27837=CARTESIAN_POINT('Ctrl Pts',(76.1026914420365,81.5372332627568,200.873903071189));
#27838=CARTESIAN_POINT('Ctrl Pts',(75.841776819832,81.2138559265676,200.901310956148));
#27839=CARTESIAN_POINT('Ctrl Pts',(75.7448670750718,81.0308722814056,200.915945557379));
#27840=CARTESIAN_POINT('Ctrl Pts',(75.6230979451896,80.630683292351,200.946397785694));
#27841=CARTESIAN_POINT('Ctrl Pts',(75.602413902907,80.4163453535111,200.961940301802));
#27842=CARTESIAN_POINT('Ctrl Pts',(75.6453970655154,80.0008258998951,200.99063959164));
#27843=CARTESIAN_POINT('Ctrl Pts',(75.7052176842617,79.8033862428561,201.002963231553));
#27844=CARTESIAN_POINT('Ctrl Pts',(75.8974535098298,79.4388732188919,201.031455263981));
#27845=CARTESIAN_POINT('Ctrl Pts',(76.0290990402504,79.2758614084399,201.046606135839));
#27846=CARTESIAN_POINT('Ctrl Pts',(76.3508490844663,79.0062252356137,201.077152076056));
#27847=CARTESIAN_POINT('Ctrl Pts',(76.5390782250257,78.9035862586545,201.092247570537));
#27848=CARTESIAN_POINT('Ctrl Pts',(76.7735964358505,78.8308509783593,201.108278832138));
#27849=CARTESIAN_POINT('Ctrl Pts',(76.8055554972657,78.8220199838071,201.110409069127));
#27850=CARTESIAN_POINT('Ctrl Pts',(76.8377292359507,78.814194574068,201.112499998088));
#27851=CARTESIAN_POINT('Ctrl Pts',(76.8377292359512,78.8141945740679,201.2));
#27852=CARTESIAN_POINT('Ctrl Pts',(76.7230577379177,78.8420853786241,201.192547650162));
#27853=CARTESIAN_POINT('Ctrl Pts',(76.6115947990365,78.8826276152677,201.184627535099));
#27854=CARTESIAN_POINT('Ctrl Pts',(76.3150545531594,79.0295937708904,201.161587591416));
#27855=CARTESIAN_POINT('Ctrl Pts',(76.145434372447,79.1608629281559,201.146032066305));
#27856=CARTESIAN_POINT('Ctrl Pts',(75.8726108484588,79.4758742834271,201.115782018085));
#27857=CARTESIAN_POINT('Ctrl Pts',(75.7696103415582,79.6546125310239,201.101350139248));
#27858=CARTESIAN_POINT('Ctrl Pts',(75.6336972630993,80.0493201135081,201.074308430542));
#27859=CARTESIAN_POINT('Ctrl Pts',(75.6052336851466,80.2625778233924,201.060286307551));
#27860=CARTESIAN_POINT('Ctrl Pts',(75.6333440080259,80.6844893975392,201.029908999931));
#27861=CARTESIAN_POINT('Ctrl Pts',(75.6882924470039,80.8889797296278,201.014473731096));
#27862=CARTESIAN_POINT('Ctrl Pts',(75.8708941126286,81.2589254386447,200.985115966184));
#27863=CARTESIAN_POINT('Ctrl Pts',(75.9943880638178,81.4220094854326,200.972215147236));
#27864=CARTESIAN_POINT('Ctrl Pts',(76.3028196954746,81.6998287002969,200.944936846831));
#27865=CARTESIAN_POINT('Ctrl Pts',(76.4873000683498,81.8090966564369,200.929787631469));
#27866=CARTESIAN_POINT('Ctrl Pts',(76.8833265687373,81.9475986645516,200.899236095611));
#27867=CARTESIAN_POINT('Ctrl Pts',(77.0904587978782,81.9773666558241,200.884131691749));
#27868=CARTESIAN_POINT('Ctrl Pts',(77.5021859648924,81.9563251671592,200.855752400869));
#27869=CARTESIAN_POINT('Ctrl Pts',(77.7028802441797,81.9066637066071,200.84340722707));
#27870=CARTESIAN_POINT('Ctrl Pts',(78.0820047419905,81.7309075887329,200.814562023466));
#27871=CARTESIAN_POINT('Ctrl Pts',(78.2553693071718,81.6036784189801,200.799012421272));
#27872=CARTESIAN_POINT('Ctrl Pts',(78.536684912461,81.2948279961493,200.768624678923));
#27873=CARTESIAN_POINT('Ctrl Pts',(78.6443066654089,81.1182412310875,200.754057389924));
#27874=CARTESIAN_POINT('Ctrl Pts',(78.7892343581798,80.7281654087846,200.726773434395));
#27875=CARTESIAN_POINT('Ctrl Pts',(78.8228831626828,80.5175960494746,200.713230635708));
#27876=CARTESIAN_POINT('Ctrl Pts',(78.8064479126939,80.0963686544912,200.683102995361));
#27877=CARTESIAN_POINT('Ctrl Pts',(78.7569066916746,79.8899114757666,200.667621554002));
#27878=CARTESIAN_POINT('Ctrl Pts',(78.5839060893216,79.5146866365054,200.638055208749));
#27879=CARTESIAN_POINT('Ctrl Pts',(78.4647172737818,79.3483417121807,200.624799640214));
#27880=CARTESIAN_POINT('Ctrl Pts',(78.1637244074197,79.0624835874737,200.597877057872));
#27881=CARTESIAN_POINT('Ctrl Pts',(77.9822244022444,78.9484014966514,200.582837696619));
#27882=CARTESIAN_POINT('Ctrl Pts',(77.5895403317286,78.7992995627259,200.552302732084));
#27883=CARTESIAN_POINT('Ctrl Pts',(77.3827169839753,78.7640755952016,200.537108085843));
#27884=CARTESIAN_POINT('Ctrl Pts',(77.0609849749371,78.7723096416387,200.514763647388));
#27885=CARTESIAN_POINT('Ctrl Pts',(76.9479785400891,78.7873793510447,200.507164957273));
#27886=CARTESIAN_POINT('Ctrl Pts',(76.8377292359511,78.8141945740679,200.5));
#27887=CARTESIAN_POINT('Origin',(77.215862801455,80.368869783441,212.));
#27888=CARTESIAN_POINT('',(76.8377292359515,78.8141945740678,201.9));
#27889=CARTESIAN_POINT('',(76.8377292359509,78.814194574068,201.812499998088));
#27890=CARTESIAN_POINT('',(76.8377292359511,78.8141945740678,212.));
#27891=CARTESIAN_POINT('Ctrl Pts',(76.8377292359507,78.814194574068,201.112499998088));
#27892=CARTESIAN_POINT('Ctrl Pts',(77.002096180345,78.7742166684835,201.123181989625));
#27893=CARTESIAN_POINT('Ctrl Pts',(77.1719446163093,78.7605016544631,201.134785981505));
#27894=CARTESIAN_POINT('Ctrl Pts',(77.5504206323416,78.7902082684024,201.161878936476));
#27895=CARTESIAN_POINT('Ctrl Pts',(77.7545082243137,78.8476990344998,201.177338653418));
#27896=CARTESIAN_POINT('Ctrl Pts',(78.1307490414463,79.0392072412851,201.207592396316));
#27897=CARTESIAN_POINT('Ctrl Pts',(78.2987375993833,79.1720620104365,201.22136567213));
#27898=CARTESIAN_POINT('Ctrl Pts',(78.5683643434518,79.4898654486178,201.248528773316));
#27899=CARTESIAN_POINT('Ctrl Pts',(78.6695876376196,79.669904966601,201.263029113832));
#27900=CARTESIAN_POINT('Ctrl Pts',(78.8012283126906,80.0658395556713,201.293350026175));
#27901=CARTESIAN_POINT('Ctrl Pts',(78.827431612851,80.2789948332638,201.308903860888));
#27902=CARTESIAN_POINT('Ctrl Pts',(78.7955064913181,80.6958435296877,201.337887888365));
#27903=CARTESIAN_POINT('Ctrl Pts',(78.7405579756507,80.8956412160388,201.350273062725));
#27904=CARTESIAN_POINT('Ctrl Pts',(78.5573221803279,81.2651798560001,201.378543447957));
#27905=CARTESIAN_POINT('Ctrl Pts',(78.4301908339087,81.4310691246104,201.393601108851));
#27906=CARTESIAN_POINT('Ctrl Pts',(78.1159056736257,81.7086411578001,201.424152898562));
#27907=CARTESIAN_POINT('Ctrl Pts',(77.9303695077314,81.8161378845038,201.439350943838));
#27908=CARTESIAN_POINT('Ctrl Pts',(77.5371465566135,81.9493450651334,201.466797419545));
#27909=CARTESIAN_POINT('Ctrl Pts',(77.334463519329,81.9773124642208,201.479558530659));
#27910=CARTESIAN_POINT('Ctrl Pts',(76.9227011821081,81.955669202413,201.508815389526));
#27911=CARTESIAN_POINT('Ctrl Pts',(76.7177123438531,81.9037039845092,201.524224888581));
#27912=CARTESIAN_POINT('Ctrl Pts',(76.3352528979562,81.7217753955709,201.554717383265));
#27913=CARTESIAN_POINT('Ctrl Pts',(76.1624405071601,81.5920017264536,201.568993031485));
#27914=CARTESIAN_POINT('Ctrl Pts',(75.8845606754058,81.2795566083094,201.595918712456));
#27915=CARTESIAN_POINT('Ctrl Pts',(75.7793351114691,81.1023953983769,201.610284091439));
#27916=CARTESIAN_POINT('Ctrl Pts',(75.638479124803,80.7107054391281,201.640463071394));
#27917=CARTESIAN_POINT('Ctrl Pts',(75.6070973802606,80.4987956067845,201.656017903278));
#27918=CARTESIAN_POINT('Ctrl Pts',(75.6285334890446,80.0807938260092,201.685264381511));
#27919=CARTESIAN_POINT('Ctrl Pts',(75.678868774513,79.8787221716487,201.697780400931));
#27920=CARTESIAN_POINT('Ctrl Pts',(75.8536545843852,79.5045335824848,201.725839235094));
#27921=CARTESIAN_POINT('Ctrl Pts',(75.9765160923403,79.3360679972547,201.740801410109));
#27922=CARTESIAN_POINT('Ctrl Pts',(76.2836526802474,79.0512728270737,201.771339847148));
#27923=CARTESIAN_POINT('Ctrl Pts',(76.4665570818323,78.9393052211639,201.786624192886));
#27924=CARTESIAN_POINT('Ctrl Pts',(76.7223422222199,78.8457039354087,201.804827717795));
#27925=CARTESIAN_POINT('Ctrl Pts',(76.7796681677926,78.8283163910155,201.808726685632));
#27926=CARTESIAN_POINT('Ctrl Pts',(76.8377292359506,78.814194574068,201.812499998088));
#27927=CARTESIAN_POINT('Ctrl Pts',(76.8377292359518,78.8141945740677,201.9));
#27928=CARTESIAN_POINT('Ctrl Pts',(76.6938364518796,78.8491926824594,201.890648597215));
#27929=CARTESIAN_POINT('Ctrl Pts',(76.5552610660449,78.9040450255853,201.880577997498));
#27930=CARTESIAN_POINT('Ctrl Pts',(76.2422647744921,79.081730899832,201.855123399538));
#27931=CARTESIAN_POINT('Ctrl Pts',(76.0810339803901,79.2213617176755,201.83958934672));
#27932=CARTESIAN_POINT('Ctrl Pts',(75.8268666155398,79.5490530352132,201.809684842051));
#27933=CARTESIAN_POINT('Ctrl Pts',(75.7340437538269,79.7320686383392,201.795653719495));
#27934=CARTESIAN_POINT('Ctrl Pts',(75.6194005766882,80.1314477387972,201.769332883082));
#27935=CARTESIAN_POINT('Ctrl Pts',(75.6020347944844,80.3450485525558,201.754498292373));
#27936=CARTESIAN_POINT('Ctrl Pts',(75.6511887998393,80.7630110843104,201.724038140283));
#27937=CARTESIAN_POINT('Ctrl Pts',(75.7158822734928,80.9635317136401,201.708716196424));
#27938=CARTESIAN_POINT('Ctrl Pts',(75.9159605933464,81.3236228721634,201.679755468037));
#27939=CARTESIAN_POINT('Ctrl Pts',(76.0475536142187,81.4807778326205,201.667290032282));
#27940=CARTESIAN_POINT('Ctrl Pts',(76.3713046110635,81.7446297174043,201.639226109827));
#27941=CARTESIAN_POINT('Ctrl Pts',(76.5630703759829,81.8452914457543,201.623743539663));
#27942=CARTESIAN_POINT('Ctrl Pts',(76.9669225350538,81.9627811359546,201.593075188823));
#27943=CARTESIAN_POINT('Ctrl Pts',(77.1742465913147,81.9815766866632,201.57818231474));
#27944=CARTESIAN_POINT('Ctrl Pts',(77.5855274997963,81.9393036158957,201.550269532907));
#27945=CARTESIAN_POINT('Ctrl Pts',(77.7854828963734,81.8783259652217,201.537623765747));
#27946=CARTESIAN_POINT('Ctrl Pts',(78.1552306389973,81.6812882661153,201.508201599785));
#27947=CARTESIAN_POINT('Ctrl Pts',(78.3204990159484,81.5455685634545,201.492651517212));
#27948=CARTESIAN_POINT('Ctrl Pts',(78.5835421545281,81.2238498476462,201.462579599162));
#27949=CARTESIAN_POINT('Ctrl Pts',(78.6812562225632,81.0428178170226,201.448311049676));
#27950=CARTESIAN_POINT('Ctrl Pts',(78.8059193648389,80.6458649932158,201.421749644208));
#27951=CARTESIAN_POINT('Ctrl Pts',(78.8286320400919,80.4327224343105,201.40731631648));
#27952=CARTESIAN_POINT('Ctrl Pts',(78.7897393059797,80.0129571686907,201.376905267632));
#27953=CARTESIAN_POINT('Ctrl Pts',(78.7297737453715,79.810440723342,201.361523392513));
#27954=CARTESIAN_POINT('Ctrl Pts',(78.5382070845839,79.4455108789494,201.332366516426));
#27955=CARTESIAN_POINT('Ctrl Pts',(78.4106033162836,79.2854683330141,201.319724000473));
#27956=CARTESIAN_POINT('Ctrl Pts',(78.0951581589779,79.0153745405877,201.292113311217));
#27957=CARTESIAN_POINT('Ctrl Pts',(77.9079624449768,78.9107650324366,201.276869595192));
#27958=CARTESIAN_POINT('Ctrl Pts',(77.5090217545997,78.7824226778875,201.246322427869));
#27959=CARTESIAN_POINT('Ctrl Pts',(77.3017272868094,78.7578419437744,201.231313018556));
#27960=CARTESIAN_POINT('Ctrl Pts',(77.0083879813496,78.7799767627696,201.211240352658));
#27961=CARTESIAN_POINT('Ctrl Pts',(76.9222038524457,78.7936483611116,201.205489894223));
#27962=CARTESIAN_POINT('Ctrl Pts',(76.8377292359512,78.8141945740679,201.2));
#27963=CARTESIAN_POINT('Origin',(77.215862801455,80.368869783441,212.));
#27964=CARTESIAN_POINT('',(76.8377292359514,78.8141945740678,202.6));
#27965=CARTESIAN_POINT('',(76.8377292359511,78.8141945740679,202.512499998088));
#27966=CARTESIAN_POINT('',(76.8377292359511,78.8141945740678,212.));
#27967=CARTESIAN_POINT('Ctrl Pts',(76.8377292359506,78.814194574068,201.812499998088));
#27968=CARTESIAN_POINT('Ctrl Pts',(76.9762100022262,78.7805127956555,201.821499680955));
#27969=CARTESIAN_POINT('Ctrl Pts',(77.1187852308018,78.7654218067803,201.831167015972));
#27970=CARTESIAN_POINT('Ctrl Pts',(77.4706856299835,78.7755288147092,201.855998513953));
#27971=CARTESIAN_POINT('Ctrl Pts',(77.6763755253127,78.8223938236945,201.871352506997));
#27972=CARTESIAN_POINT('Ctrl Pts',(78.0611875659895,78.9939077323625,201.901796106966));
#27973=CARTESIAN_POINT('Ctrl Pts',(78.2358867540984,79.1180567371074,201.9164562534));
#27974=CARTESIAN_POINT('Ctrl Pts',(78.5207761799292,79.4208792557371,201.942820956645));
#27975=CARTESIAN_POINT('Ctrl Pts',(78.6306947572285,79.5944745243928,201.957014557878));
#27976=CARTESIAN_POINT('Ctrl Pts',(78.7824296010498,79.9808002601524,201.987000948317));
#27977=CARTESIAN_POINT('Ctrl Pts',(78.8199584472721,80.1910568647587,202.002544578073));
#27978=CARTESIAN_POINT('Ctrl Pts',(78.8111368859214,80.6102990582761,202.032096322967));
#27979=CARTESIAN_POINT('Ctrl Pts',(78.7663473376232,80.8151555974517,202.04486045999));
#27980=CARTESIAN_POINT('Ctrl Pts',(78.6016170787386,81.1947886023995,202.072663062479));
#27981=CARTESIAN_POINT('Ctrl Pts',(78.4838674210283,81.3661604151088,202.08750195263));
#27982=CARTESIAN_POINT('Ctrl Pts',(78.184136943868,81.6604923331254,202.118129942819));
#27983=CARTESIAN_POINT('Ctrl Pts',(78.0027702393406,81.7783566227766,202.133630081357));
#27984=CARTESIAN_POINT('Ctrl Pts',(77.6143641095551,81.9317426641497,202.161838500422));
#27985=CARTESIAN_POINT('Ctrl Pts',(77.4127123815164,81.969692995123,202.174239265294));
#27986=CARTESIAN_POINT('Ctrl Pts',(77.0008164813083,81.967998794392,202.203096481991));
#27987=CARTESIAN_POINT('Ctrl Pts',(76.7945328665446,81.9264079908878,202.218383890842));
#27988=CARTESIAN_POINT('Ctrl Pts',(76.4061079448048,81.7650485970622,202.24887211865));
#27989=CARTESIAN_POINT('Ctrl Pts',(76.228246120193,81.6454598752063,202.263769792534));
#27990=CARTESIAN_POINT('Ctrl Pts',(75.936023256796,81.3503159801701,202.290269065912));
#27991=CARTESIAN_POINT('Ctrl Pts',(75.8218523556062,81.1800726257038,202.304047890935));
#27992=CARTESIAN_POINT('Ctrl Pts',(75.6603051897079,80.7986774888497,202.333854035404));
#27993=CARTESIAN_POINT('Ctrl Pts',(75.6172481277875,80.5900740663342,202.349375801221));
#27994=CARTESIAN_POINT('Ctrl Pts',(75.6145538929958,80.1698427195119,202.379196076377));
#27995=CARTESIAN_POINT('Ctrl Pts',(75.6542734625885,79.9624016441777,202.392269966595));
#27996=CARTESIAN_POINT('Ctrl Pts',(75.8099217931421,79.5779335637995,202.419837008763));
#27997=CARTESIAN_POINT('Ctrl Pts',(75.9230336172966,79.4040863928646,202.43455592085));
#27998=CARTESIAN_POINT('Ctrl Pts',(76.2143656873324,79.1029285681267,202.465084638613));
#27999=CARTESIAN_POINT('Ctrl Pts',(76.3921036130363,78.9806865815961,202.480613800882));
#28000=CARTESIAN_POINT('Ctrl Pts',(76.6694358785856,78.8625050380408,202.501191377896));
#28001=CARTESIAN_POINT('Ctrl Pts',(76.7527509576043,78.8348632894291,202.506977371544));
#28002=CARTESIAN_POINT('Ctrl Pts',(76.8377292359511,78.8141945740679,202.512499998088));
#28003=CARTESIAN_POINT('Ctrl Pts',(76.8377292359516,78.8141945740678,202.6));
#28004=CARTESIAN_POINT('Ctrl Pts',(76.6646070678815,78.856301955909,202.588749017992));
#28005=CARTESIAN_POINT('Ctrl Pts',(76.4995220554568,78.927069548299,202.57647890982));
#28006=CARTESIAN_POINT('Ctrl Pts',(76.1727024693801,79.1376303595131,202.54864000143));
#28007=CARTESIAN_POINT('Ctrl Pts',(76.0202253226858,79.2850865375819,202.533173635364));
#28008=CARTESIAN_POINT('Ctrl Pts',(75.785085469934,79.6245399372925,202.503680475096));
#28009=CARTESIAN_POINT('Ctrl Pts',(75.7023808492954,79.8116672127639,202.490559709967));
#28010=CARTESIAN_POINT('Ctrl Pts',(75.60907673497,80.2161288047186,202.463511044933));
#28011=CARTESIAN_POINT('Ctrl Pts',(75.6030216878962,80.4304323543675,202.448431750691));
#28012=CARTESIAN_POINT('Ctrl Pts',(75.6740690524535,80.8442431514089,202.41788847292));
#28013=CARTESIAN_POINT('Ctrl Pts',(75.7487034949919,81.0401163284464,202.40272449686));
#28014=CARTESIAN_POINT('Ctrl Pts',(75.9669404037729,81.3896371253457,202.374199769453));
#28015=CARTESIAN_POINT('Ctrl Pts',(76.107357250502,81.5406148905507,202.361878505874));
#28016=CARTESIAN_POINT('Ctrl Pts',(76.444720054825,81.7869127503183,202.33322198109));
#28017=CARTESIAN_POINT('Ctrl Pts',(76.6404150839586,81.8769616733207,202.317682039826));
#28018=CARTESIAN_POINT('Ctrl Pts',(77.0476648644173,81.9731814942715,202.287212006857));
#28019=CARTESIAN_POINT('Ctrl Pts',(77.2546353041046,81.9815200715456,202.272558262148));
#28020=CARTESIAN_POINT('Ctrl Pts',(77.6652092200424,81.9187758298425,202.2451146446));
#28021=CARTESIAN_POINT('Ctrl Pts',(77.8645728091164,81.8464785613806,202.231848865544));
#28022=CARTESIAN_POINT('Ctrl Pts',(78.2245532592939,81.6285998555793,202.201892517827));
#28023=CARTESIAN_POINT('Ctrl Pts',(78.3814638780194,81.4850000600263,202.186386486057));
#28024=CARTESIAN_POINT('Ctrl Pts',(78.6261457339997,81.1513913913891,202.156684335572));
#28025=CARTESIAN_POINT('Ctrl Pts',(78.7139194375733,80.9663568862993,202.143148093666));
#28026=CARTESIAN_POINT('Ctrl Pts',(78.8179992237349,80.5644096613865,202.116463267638));
#28027=CARTESIAN_POINT('Ctrl Pts',(78.829766885834,80.3503835666105,202.101502074866));
#28028=CARTESIAN_POINT('Ctrl Pts',(78.7697317797069,79.9343326915472,202.070989855529));
#28029=CARTESIAN_POINT('Ctrl Pts',(78.7000767279325,79.7360532648683,202.05574120217));
#28030=CARTESIAN_POINT('Ctrl Pts',(78.4909851176621,79.3811667102691,202.026993902738));
#28031=CARTESIAN_POINT('Ctrl Pts',(78.3550679719725,79.2270733216115,202.014640712796));
#28032=CARTESIAN_POINT('Ctrl Pts',(78.0245761176084,78.9718244017,201.986281472537));
#28033=CARTESIAN_POINT('Ctrl Pts',(77.8308069317692,78.8763664334322,201.970765398229));
#28034=CARTESIAN_POINT('Ctrl Pts',(77.4251468706189,78.7693327543938,201.940184904414));
#28035=CARTESIAN_POINT('Ctrl Pts',(77.2179313168644,78.755690162093,201.925405266856));
#28036=CARTESIAN_POINT('Ctrl Pts',(76.9544226574544,78.7892401951527,201.907654035774));
#28037=CARTESIAN_POINT('Ctrl Pts',(76.8956524436015,78.8001062880373,201.903764353083));
#28038=CARTESIAN_POINT('Ctrl Pts',(76.8377292359518,78.8141945740677,201.9));
#28039=CARTESIAN_POINT('Origin',(77.215862801455,80.368869783441,212.));
#28040=CARTESIAN_POINT('',(76.8377292359511,78.8141945740679,203.3));
#28041=CARTESIAN_POINT('',(76.8377292359512,78.8141945740679,203.212499998088));
#28042=CARTESIAN_POINT('',(76.8377292359511,78.8141945740678,212.));
#28043=CARTESIAN_POINT('Ctrl Pts',(76.8377292359511,78.8141945740679,202.512499998088));
#28044=CARTESIAN_POINT('Ctrl Pts',(76.9500920619865,78.7868652928247,202.51980231037));
#28045=CARTESIAN_POINT('Ctrl Pts',(77.0653056844449,78.7717391726939,202.527554292286));
#28046=CARTESIAN_POINT('Ctrl Pts',(77.3893336275295,78.7647665223466,202.550085249776));
#28047=CARTESIAN_POINT('Ctrl Pts',(77.5960944244831,78.8008631407702,202.56529340978));
#28048=CARTESIAN_POINT('Ctrl Pts',(77.9882175675707,78.95165226197,202.595823713416));
#28049=CARTESIAN_POINT('Ctrl Pts',(78.1692291048146,79.0664961932466,202.610844513016));
#28050=CARTESIAN_POINT('Ctrl Pts',(78.4690258570057,79.3536327069185,202.637709606131));
#28051=CARTESIAN_POINT('Ctrl Pts',(78.5875269392153,79.5205057199764,202.651029892044));
#28052=CARTESIAN_POINT('Ctrl Pts',(78.7589742726706,79.8965755449381,202.680629338512));
#28053=CARTESIAN_POINT('Ctrl Pts',(78.8076379840997,80.1033365357275,202.69611718347));
#28054=CARTESIAN_POINT('Ctrl Pts',(78.8221977655505,80.5244400183927,202.726203725202));
#28055=CARTESIAN_POINT('Ctrl Pts',(78.7877185822718,80.7345799163406,202.739676345269));
#28056=CARTESIAN_POINT('Ctrl Pts',(78.641334871577,81.1239004584044,202.766999066895));
#28057=CARTESIAN_POINT('Ctrl Pts',(78.5329669010044,81.3001267103364,202.781587561648));
#28058=CARTESIAN_POINT('Ctrl Pts',(78.2502851872322,81.6079556529771,202.811995925023));
#28059=CARTESIAN_POINT('Ctrl Pts',(78.0763213489491,81.7345190774253,202.827543614474));
#28060=CARTESIAN_POINT('Ctrl Pts',(77.6965039804361,81.9086498271757,202.856343525423));
#28061=CARTESIAN_POINT('Ctrl Pts',(77.4957458395885,81.9574553264438,202.868679877669));
#28062=CARTESIAN_POINT('Ctrl Pts',(77.0839964270015,81.9768602172663,202.89709427811));
#28063=CARTESIAN_POINT('Ctrl Pts',(76.876902972486,81.9462428206874,202.912213382904));
#28064=CARTESIAN_POINT('Ctrl Pts',(76.4813781696558,81.8060847737485,202.942763763888));
#28065=CARTESIAN_POINT('Ctrl Pts',(76.2973534315962,81.6960615643215,202.957896580053));
#28066=CARTESIAN_POINT('Ctrl Pts',(75.9900755620327,81.4169853029186,202.985119917269));
#28067=CARTESIAN_POINT('Ctrl Pts',(75.8672527319711,81.2533980005801,202.998070339886));
#28068=CARTESIAN_POINT('Ctrl Pts',(75.6861337459197,80.8826307577042,203.027460760865));
#28069=CARTESIAN_POINT('Ctrl Pts',(75.6320182500649,80.6778267302832,203.042903901538));
#28070=CARTESIAN_POINT('Ctrl Pts',(75.6057201100339,80.2560113946526,203.073243161843));
#28071=CARTESIAN_POINT('Ctrl Pts',(75.6349904960173,80.0431724977292,203.087186166083));
#28072=CARTESIAN_POINT('Ctrl Pts',(75.772297337779,79.6491760351658,203.11426558087));
#28073=CARTESIAN_POINT('Ctrl Pts',(75.8760123302209,79.4707613901058,203.12871885026));
#28074=CARTESIAN_POINT('Ctrl Pts',(76.1501523617184,79.1566841957607,203.158991299902));
#28075=CARTESIAN_POINT('Ctrl Pts',(76.3203551504402,79.0260304256433,203.174546568817));
#28076=CARTESIAN_POINT('Ctrl Pts',(76.6156282801234,78.8811637812547,203.197413972362));
#28077=CARTESIAN_POINT('Ctrl Pts',(76.7251381748456,78.8415793674466,203.20518285311));
#28078=CARTESIAN_POINT('Ctrl Pts',(76.8377292359512,78.8141945740678,203.212499998088));
#28079=CARTESIAN_POINT('Ctrl Pts',(76.8377292359511,78.8141945740679,203.3));
#28080=CARTESIAN_POINT('Ctrl Pts',(76.6372977216527,78.8629442310278,203.286974219498));
#28081=CARTESIAN_POINT('Ctrl Pts',(76.4480122774094,78.9500342613071,203.272605893883));
#28082=CARTESIAN_POINT('Ctrl Pts',(76.1108217964156,79.1930409508577,203.242586366163));
#28083=CARTESIAN_POINT('Ctrl Pts',(75.9668196527448,79.3473072665555,203.227224106349));
#28084=CARTESIAN_POINT('Ctrl Pts',(75.7494649935569,79.6973827808235,203.198134164226));
#28085=CARTESIAN_POINT('Ctrl Pts',(75.6762084806871,79.8885959629813,203.185560243896));
#28086=CARTESIAN_POINT('Ctrl Pts',(75.6034036952677,80.2975370860574,203.157840941478));
#28087=CARTESIAN_POINT('Ctrl Pts',(75.6081911415612,80.511934678872,203.142568139288));
#28088=CARTESIAN_POINT('Ctrl Pts',(75.6998893912881,80.9206962237656,203.112026737038));
#28089=CARTESIAN_POINT('Ctrl Pts',(75.7837462118058,81.1116738560253,203.097050689625));
#28090=CARTESIAN_POINT('Ctrl Pts',(76.0192541893987,81.4508407679873,203.068961919911));
#28091=CARTESIAN_POINT('Ctrl Pts',(76.1684804602313,81.595870075341,203.056468577965));
#28092=CARTESIAN_POINT('Ctrl Pts',(76.5188873796324,81.824638891677,203.027258663057));
#28093=CARTESIAN_POINT('Ctrl Pts',(76.7178923993662,81.9041376018337,203.011703401217));
#28094=CARTESIAN_POINT('Ctrl Pts',(77.1274173827322,81.9794214382293,202.981503382356));
#28095=CARTESIAN_POINT('Ctrl Pts',(77.3335325747862,81.9775639318118,202.967118520072));
#28096=CARTESIAN_POINT('Ctrl Pts',(77.7431344316525,81.8945236225489,202.940159024976));
#28097=CARTESIAN_POINT('Ctrl Pts',(77.9419643006599,81.8105649155683,202.925958811281));
#28098=CARTESIAN_POINT('Ctrl Pts',(78.2914932282357,81.5717502819813,202.895499590603));
#28099=CARTESIAN_POINT('Ctrl Pts',(78.4396099246003,81.420701942175,202.880082342266));
#28100=CARTESIAN_POINT('Ctrl Pts',(78.665531412132,81.0756999302961,202.850796012158));
#28101=CARTESIAN_POINT('Ctrl Pts',(78.7433412207922,80.8864863936483,202.837996197978));
#28102=CARTESIAN_POINT('Ctrl Pts',(78.8260886097391,80.4796673400736,202.810598583886));
#28103=CARTESIAN_POINT('Ctrl Pts',(78.8265534067992,80.2652446547458,202.795414513933));
#28104=CARTESIAN_POINT('Ctrl Pts',(78.7448180217156,79.8539070798602,202.76486228372));
#28105=CARTESIAN_POINT('Ctrl Pts',(78.6653915531734,79.6605044068468,202.749790766244));
#28106=CARTESIAN_POINT('Ctrl Pts',(78.438240109404,79.3162917588312,202.721488505881));
#28107=CARTESIAN_POINT('Ctrl Pts',(78.2933285442398,79.1683714342946,202.709117001913));
#28108=CARTESIAN_POINT('Ctrl Pts',(77.9492420811693,78.9310170139922,202.680173343095));
#28109=CARTESIAN_POINT('Ctrl Pts',(77.7517825479673,78.8463604418928,202.664620482353));
#28110=CARTESIAN_POINT('Ctrl Pts',(77.3432353358874,78.7608667615476,202.634279564757));
#28111=CARTESIAN_POINT('Ctrl Pts',(77.1366405681677,78.7577638908535,202.619759448272));
#28112=CARTESIAN_POINT('Ctrl Pts',(76.9023534571558,78.7995343618604,202.604221532181));
#28113=CARTESIAN_POINT('Ctrl Pts',(76.8699047618658,78.8063687296325,202.602091045111));
#28114=CARTESIAN_POINT('Ctrl Pts',(76.8377292359516,78.8141945740678,202.6));
#28115=CARTESIAN_POINT('Origin',(77.215862801455,80.368869783441,212.));
#28116=CARTESIAN_POINT('',(76.837729235951,78.8141945740679,204.));
#28117=CARTESIAN_POINT('',(76.8377292359514,78.8141945740678,203.912499998088));
#28118=CARTESIAN_POINT('',(76.8377292359511,78.8141945740678,212.));
#28119=CARTESIAN_POINT('Ctrl Pts',(76.8377292359512,78.8141945740678,203.212499998088));
#28120=CARTESIAN_POINT('Ctrl Pts',(76.9241273372014,78.7931805243927,203.218114897055));
#28121=CARTESIAN_POINT('Ctrl Pts',(77.012306563947,78.7793593757555,203.224001896763));
#28122=CARTESIAN_POINT('Ctrl Pts',(77.3077870837124,78.7581666254124,203.244243708424));
#28123=CARTESIAN_POINT('Ctrl Pts',(77.5150650290347,78.7835412677283,203.259268237987));
#28124=CARTESIAN_POINT('Ctrl Pts',(77.913576391502,78.9134437113486,203.289817347387));
#28125=CARTESIAN_POINT('Ctrl Pts',(78.1003640252084,79.018771336565,203.305047230497));
#28126=CARTESIAN_POINT('Ctrl Pts',(78.4147392583877,79.2900531834865,203.332607408692));
#28127=CARTESIAN_POINT('Ctrl Pts',(78.5417125300506,79.4505578745941,203.345284507738));
#28128=CARTESIAN_POINT('Ctrl Pts',(78.7319167218548,79.8162553533708,203.374472292603));
#28129=CARTESIAN_POINT('Ctrl Pts',(78.7911220914528,80.0190802911365,203.389862924639));
#28130=CARTESIAN_POINT('Ctrl Pts',(78.8283685512414,80.4390815528904,203.4202623244));
#28131=CARTESIAN_POINT('Ctrl Pts',(78.8048153931099,80.6521430613691,203.434623965844));
#28132=CARTESIAN_POINT('Ctrl Pts',(78.6785510432537,81.0486930086231,203.461249538411));
#28133=CARTESIAN_POINT('Ctrl Pts',(78.58006767538,81.2294021349393,203.475542404649));
#28134=CARTESIAN_POINT('Ctrl Pts',(78.3155969671828,81.5501669294063,203.50564158689));
#28135=CARTESIAN_POINT('Ctrl Pts',(78.1496908439536,81.6852500983994,203.521193256682));
#28136=CARTESIAN_POINT('Ctrl Pts',(77.7792024180381,81.8806537051101,203.550572212483));
#28137=CARTESIAN_POINT('Ctrl Pts',(77.5791959821053,81.9407545056932,203.563182834373));
#28138=CARTESIAN_POINT('Ctrl Pts',(77.1678707790729,81.9814097036313,203.591131884754));
#28139=CARTESIAN_POINT('Ctrl Pts',(76.9605411325661,81.9617818432542,203.60604221372));
#28140=CARTESIAN_POINT('Ctrl Pts',(76.5570052405901,81.8426078743946,203.636722964176));
#28141=CARTESIAN_POINT('Ctrl Pts',(76.3655752667733,81.7411103402857,203.652199172683));
#28142=CARTESIAN_POINT('Ctrl Pts',(76.042919470818,81.4758765817549,203.680214788941));
#28143=CARTESIAN_POINT('Ctrl Pts',(75.9120212040928,81.3182231903672,203.692705925547));
#28144=CARTESIAN_POINT('Ctrl Pts',(75.7134116942629,80.9572917520173,203.721700877182));
#28145=CARTESIAN_POINT('Ctrl Pts',(75.6495313326676,80.75641830372,203.737033806571));
#28146=CARTESIAN_POINT('Ctrl Pts',(75.6021520058948,80.3381721085283,203.76748347411));
#28147=CARTESIAN_POINT('Ctrl Pts',(75.6204264800724,80.1246547157139,203.78229649554));
#28148=CARTESIAN_POINT('Ctrl Pts',(75.7392370785646,79.7172975776863,203.809110768139));
#28149=CARTESIAN_POINT('Ctrl Pts',(75.8385447395526,79.5273909602021,203.823891447406));
#28150=CARTESIAN_POINT('Ctrl Pts',(76.1035016204051,79.1999979744398,203.854349997429));
#28151=CARTESIAN_POINT('Ctrl Pts',(76.2653990345763,79.0649378230296,203.869689078905));
#28152=CARTESIAN_POINT('Ctrl Pts',(76.5714943646726,78.8976877949465,203.894254263654));
#28153=CARTESIAN_POINT('Ctrl Pts',(76.7022797579508,78.8471390718981,203.90369731466));
#28154=CARTESIAN_POINT('Ctrl Pts',(76.8377292359517,78.8141945740677,203.912499998088));
#28155=CARTESIAN_POINT('Ctrl Pts',(76.837729235951,78.8141945740679,204.));
#28156=CARTESIAN_POINT('Ctrl Pts',(76.8164855339289,78.8193615418961,203.998619399746));
#28157=CARTESIAN_POINT('Ctrl Pts',(76.7953336269056,78.8249673612387,203.997221545057));
#28158=CARTESIAN_POINT('Ctrl Pts',(76.5702076437519,78.8896092732629,203.982093149827));
#28159=CARTESIAN_POINT('Ctrl Pts',(76.379877358006,78.988231115077,203.967089096228));
#28160=CARTESIAN_POINT('Ctrl Pts',(76.052182681302,79.2512379244776,203.93656340598));
#28161=CARTESIAN_POINT('Ctrl Pts',(75.9168985765468,79.4118106224138,203.92134343455));
#28162=CARTESIAN_POINT('Ctrl Pts',(75.7173468648551,79.7721845900864,203.892673943122));
#28163=CARTESIAN_POINT('Ctrl Pts',(75.6535940004212,79.9677531423396,203.880341579362));
#28164=CARTESIAN_POINT('Ctrl Pts',(75.6017095244076,80.3821222569537,203.851877185503));
#28165=CARTESIAN_POINT('Ctrl Pts',(75.617910585001,80.5973130085841,203.836351500336));
#28166=CARTESIAN_POINT('Ctrl Pts',(75.7316246771356,81.0007568706779,203.805807470381));
#28167=CARTESIAN_POINT('Ctrl Pts',(75.8249951750216,81.1860397767841,203.79107095462));
#28168=CARTESIAN_POINT('Ctrl Pts',(76.0788889363189,81.5138488439366,203.763470064755));
#28169=CARTESIAN_POINT('Ctrl Pts',(76.2379921095794,81.6524110555826,203.750445306723));
#28170=CARTESIAN_POINT('Ctrl Pts',(76.6023298567526,81.86155586569,203.720662903977));
#28171=CARTESIAN_POINT('Ctrl Pts',(76.8043330498887,81.929373209693,203.705137331507));
#28172=CARTESIAN_POINT('Ctrl Pts',(77.2153498303632,81.9817368008845,203.675302826279));
#28173=CARTESIAN_POINT('Ctrl Pts',(77.4199800269579,81.9687392875352,203.661453567262));
#28174=CARTESIAN_POINT('Ctrl Pts',(77.8221215248086,81.8647030127121,203.635005444164));
#28175=CARTESIAN_POINT('Ctrl Pts',(78.0149588024898,81.7711753785389,203.620125656083));
#28176=CARTESIAN_POINT('Ctrl Pts',(78.3499058242012,81.5166596610425,203.589644980771));
#28177=CARTESIAN_POINT('Ctrl Pts',(78.4896859687075,81.359255298631,203.574347400866));
#28178=CARTESIAN_POINT('Ctrl Pts',(78.6983654995234,81.0041209070582,203.54546029511));
#28179=CARTESIAN_POINT('Ctrl Pts',(78.7670003086117,80.8108199384722,203.533042856392));
#28180=CARTESIAN_POINT('Ctrl Pts',(78.8298836226726,80.397973906022,203.504875913675));
#28181=CARTESIAN_POINT('Ctrl Pts',(78.8192659813997,80.1818536772977,203.489380591157));
#28182=CARTESIAN_POINT('Ctrl Pts',(78.71562951968,79.7746029993714,203.458740508447));
#28183=CARTESIAN_POINT('Ctrl Pts',(78.6267107702664,79.5865698158039,203.443885847968));
#28184=CARTESIAN_POINT('Ctrl Pts',(78.3815021773898,79.2533512277332,203.416051356147));
#28185=CARTESIAN_POINT('Ctrl Pts',(78.2271316518134,79.1117122007809,203.403323256942));
#28186=CARTESIAN_POINT('Ctrl Pts',(77.8693760757632,78.8931687495223,203.373808755235));
#28187=CARTESIAN_POINT('Ctrl Pts',(77.6687173886042,78.8197782963812,203.35826300697));
#28188=CARTESIAN_POINT('Ctrl Pts',(77.258361291222,78.7565235724923,203.32825144718));
#28189=CARTESIAN_POINT('Ctrl Pts',(77.0529632663945,78.7641962158736,203.314035988574));
#28190=CARTESIAN_POINT('Ctrl Pts',(76.8488878959581,78.8115122881281,203.300725837822));
#28191=CARTESIAN_POINT('Ctrl Pts',(76.843304322095,78.8128385820325,203.300362317516));
#28192=CARTESIAN_POINT('Ctrl Pts',(76.8377292359511,78.8141945740679,203.3));
#28193=CARTESIAN_POINT('Origin',(77.215862801455,80.368869783441,212.));
#28194=CARTESIAN_POINT('',(76.8377292359508,78.8141945740679,204.7));
#28195=CARTESIAN_POINT('',(76.8377292359514,78.8141945740678,204.612499998088));
#28196=CARTESIAN_POINT('',(76.8377292359511,78.8141945740678,212.));
#28197=CARTESIAN_POINT('Ctrl Pts',(76.8377292359517,78.8141945740677,203.912499998088));
#28198=CARTESIAN_POINT('Ctrl Pts',(76.8988718220249,78.7993232595085,203.916473574341));
#28199=CARTESIAN_POINT('Ctrl Pts',(76.9609484409753,78.7880445652141,203.920586164267));
#28200=CARTESIAN_POINT('Ctrl Pts',(77.2345219185842,78.7549405019645,203.939050825753));
#28201=CARTESIAN_POINT('Ctrl Pts',(77.4483288436784,78.7716722576286,203.954355028478));
#28202=CARTESIAN_POINT('Ctrl Pts',(77.851172785091,78.8859699802009,203.984887388585));
#28203=CARTESIAN_POINT('Ctrl Pts',(78.0370246036382,78.9802253934054,203.999824789487));
#28204=CARTESIAN_POINT('Ctrl Pts',(78.3628087403947,79.2343114574565,204.027830765998));
#28205=CARTESIAN_POINT('Ctrl Pts',(78.49957164793,79.3917273975043,204.040390105629));
#28206=CARTESIAN_POINT('Ctrl Pts',(78.7083973684543,79.7546288016049,204.069700683849));
#28207=CARTESIAN_POINT('Ctrl Pts',(78.7765593331449,79.9575757023486,204.085254302958));
#28208=CARTESIAN_POINT('Ctrl Pts',(78.8288169372792,80.3702798779705,204.115395378047));
#28209=CARTESIAN_POINT('Ctrl Pts',(78.8155049889549,80.5757823535477,204.129726051018));
#28210=CARTESIAN_POINT('Ctrl Pts',(78.7097250467114,80.9806973275376,204.15659184709));
#28211=CARTESIAN_POINT('Ctrl Pts',(78.6143813798786,81.1752118164232,204.171004160665));
#28212=CARTESIAN_POINT('Ctrl Pts',(78.355720693294,81.511032958448,204.201554986642));
#28213=CARTESIAN_POINT('Ctrl Pts',(78.1966810946415,81.6502032825951,204.216950284698));
#28214=CARTESIAN_POINT('Ctrl Pts',(77.8396015994553,81.856189009366,204.246154823755));
#28215=CARTESIAN_POINT('Ctrl Pts',(77.6462404194208,81.923192277403,204.258851443234));
#28216=CARTESIAN_POINT('Ctrl Pts',(77.2353161315612,81.9827870629292,204.286384147099));
#28217=CARTESIAN_POINT('Ctrl Pts',(77.0211989834806,81.9711101397455,204.301606425426));
#28218=CARTESIAN_POINT('Ctrl Pts',(76.615335803055,81.8662585490563,204.332156396177));
#28219=CARTESIAN_POINT('Ctrl Pts',(76.4269128279573,81.7761329740433,204.347189045765));
#28220=CARTESIAN_POINT('Ctrl Pts',(76.0958707106108,81.5298631867101,204.375402703916));
#28221=CARTESIAN_POINT('Ctrl Pts',(75.9561209801514,81.376511614043,204.387816171576));
#28222=CARTESIAN_POINT('Ctrl Pts',(75.7386702935091,81.019310546269,204.416871505808));
#28223=CARTESIAN_POINT('Ctrl Pts',(75.6654390627978,80.8175766914384,204.432426536183));
#28224=CARTESIAN_POINT('Ctrl Pts',(75.6032591828435,80.4052628385412,204.462710943586));
#28225=CARTESIAN_POINT('Ctrl Pts',(75.6118021416659,80.1990274982907,204.477175723138));
#28226=CARTESIAN_POINT('Ctrl Pts',(75.7079797728761,79.7931454698215,204.504275509328));
#28227=CARTESIAN_POINT('Ctrl Pts',(75.7977057640665,79.5981176371529,204.518176447608));
#28228=CARTESIAN_POINT('Ctrl Pts',(76.0466229463546,79.256702584626,204.548495027017));
#28229=CARTESIAN_POINT('Ctrl Pts',(76.2024148198878,79.1130975564851,204.563942316811));
#28230=CARTESIAN_POINT('Ctrl Pts',(76.5230643351593,78.9171242773603,204.59072132588));
#28231=CARTESIAN_POINT('Ctrl Pts',(76.6769744816766,78.8532939100829,204.602052758037));
#28232=CARTESIAN_POINT('Ctrl Pts',(76.8377292359517,78.8141945740677,204.612499998088));
#28233=CARTESIAN_POINT('Ctrl Pts',(76.8377292359504,78.814194574068,204.7));
#28234=CARTESIAN_POINT('Ctrl Pts',(76.7895023846101,78.8259244782567,204.696865800361));
#28235=CARTESIAN_POINT('Ctrl Pts',(76.7417728761323,78.839910017265,204.693644261852));
#28236=CARTESIAN_POINT('Ctrl Pts',(76.4938954972622,78.9253081860543,204.676270834625));
#28237=CARTESIAN_POINT('Ctrl Pts',(76.3089114608851,79.0337642943317,204.661053605709));
#28238=CARTESIAN_POINT('Ctrl Pts',(75.9961373947811,79.3128929183864,204.630503141403));
#28239=CARTESIAN_POINT('Ctrl Pts',(75.869912812526,79.4793409245744,204.615465173399));
#28240=CARTESIAN_POINT('Ctrl Pts',(75.6884760444571,79.8498753363947,204.587239536817));
#28241=CARTESIAN_POINT('Ctrl Pts',(75.634506484563,80.0501519397626,204.574832463734));
#28242=CARTESIAN_POINT('Ctrl Pts',(75.6048059548743,80.4672542826168,204.545792129521));
#28243=CARTESIAN_POINT('Ctrl Pts',(75.6321123575831,80.6801553782358,204.530237294496));
#28244=CARTESIAN_POINT('Ctrl Pts',(75.765719886486,81.0752064958853,204.499945082958));
#28245=CARTESIAN_POINT('Ctrl Pts',(75.8677994169808,81.2546423771457,204.485472755538));
#28246=CARTESIAN_POINT('Ctrl Pts',(76.1391774391111,81.5713152242223,204.458359578796));
#28247=CARTESIAN_POINT('Ctrl Pts',(76.3081802069298,81.703521786783,204.444486029876));
#28248=CARTESIAN_POINT('Ctrl Pts',(76.6857425560261,81.8930165113386,204.41418109223));
#28249=CARTESIAN_POINT('Ctrl Pts',(76.8900327571334,81.9493406730169,204.398731114972));
#28250=CARTESIAN_POINT('Ctrl Pts',(77.3016575938514,81.9793913559084,204.369311511891));
#28251=CARTESIAN_POINT('Ctrl Pts',(77.5048308707005,81.9555633877178,204.356314921111));
#28252=CARTESIAN_POINT('Ctrl Pts',(77.9006129346417,81.8304487340569,204.329140925675));
#28253=CARTESIAN_POINT('Ctrl Pts',(78.0882869780496,81.7267830290852,204.314023013219));
#28254=CARTESIAN_POINT('Ctrl Pts',(78.408484830022,81.455462088244,204.283474112372));
#28255=CARTESIAN_POINT('Ctrl Pts',(78.5391868263776,81.2918354512038,204.26834204869));
#28256=CARTESIAN_POINT('Ctrl Pts',(78.7295346840857,80.9262629150247,204.23989624657));
#28257=CARTESIAN_POINT('Ctrl Pts',(78.7883371621984,80.7283325701793,204.227566227471));
#28258=CARTESIAN_POINT('Ctrl Pts',(78.8290107934515,80.3125269232905,204.198806861185));
#28259=CARTESIAN_POINT('Ctrl Pts',(78.8071692961944,80.0984247812819,204.183261105522));
#28260=CARTESIAN_POINT('Ctrl Pts',(78.6833257917591,79.6991052315307,204.152834730954));
#28261=CARTESIAN_POINT('Ctrl Pts',(78.5855074054855,79.5167285662415,204.138227476604));
#28262=CARTESIAN_POINT('Ctrl Pts',(78.3227723413209,79.1945090391943,204.110870252639));
#28263=CARTESIAN_POINT('Ctrl Pts',(78.1587258780098,79.0591300213629,204.09745853139));
#28264=CARTESIAN_POINT('Ctrl Pts',(77.7876934999827,78.8597972340702,204.067408833216));
#28265=CARTESIAN_POINT('Ctrl Pts',(77.5844613521762,78.7977480600917,204.051915521329));
#28266=CARTESIAN_POINT('Ctrl Pts',(77.1948987284957,78.7587945493212,204.023857202725));
#28267=CARTESIAN_POINT('Ctrl Pts',(77.0132492514773,78.7715039793455,204.011406814961));
#28268=CARTESIAN_POINT('Ctrl Pts',(76.837729235951,78.8141945740679,204.));
#28269=CARTESIAN_POINT('Origin',(77.215862801455,80.368869783441,212.));
#28270=CARTESIAN_POINT('',(76.8377292359511,78.8141945740679,205.4));
#28271=CARTESIAN_POINT('',(76.8377292359511,78.8141945740679,205.312499998088));
#28272=CARTESIAN_POINT('',(76.8377292359511,78.8141945740678,212.));
#28273=CARTESIAN_POINT('Ctrl Pts',(76.8377292359517,78.8141945740677,204.612499998088));
#28274=CARTESIAN_POINT('Ctrl Pts',(76.87347087857,78.8055013662011,204.614822800434));
#28275=CARTESIAN_POINT('Ctrl Pts',(76.9095453758351,78.798032605701,204.617193997504));
#28276=CARTESIAN_POINT('Ctrl Pts',(77.1552066426569,78.7559788113551,204.633522013413));
#28277=CARTESIAN_POINT('Ctrl Pts',(77.3695205837571,78.7621829690208,204.648645861751));
#28278=CARTESIAN_POINT('Ctrl Pts',(77.7783972624879,78.8567279410647,204.67919540006));
#28279=CARTESIAN_POINT('Ctrl Pts',(77.9694989853232,78.9423100573504,204.694322347149));
#28280=CARTESIAN_POINT('Ctrl Pts',(78.3061629355851,79.1801080401349,204.722755708176));
#28281=CARTESIAN_POINT('Ctrl Pts',(78.4491193968819,79.3291646858567,204.735088043748));
#28282=CARTESIAN_POINT('Ctrl Pts',(78.6757029845035,79.6801941721309,204.763863498823));
#28283=CARTESIAN_POINT('Ctrl Pts',(78.7543279674699,79.8804964119921,204.779410046368));
#28284=CARTESIAN_POINT('Ctrl Pts',(78.8271145261591,80.2921341074044,204.809829328457));
#28285=CARTESIAN_POINT('Ctrl Pts',(78.8236929481159,80.4990300614199,204.82442916817));
#28286=CARTESIAN_POINT('Ctrl Pts',(78.7377174705474,80.9058713827151,204.851772731434));
#28287=CARTESIAN_POINT('Ctrl Pts',(78.6538446117614,81.1014397604285,204.86520838787));
#28288=CARTESIAN_POINT('Ctrl Pts',(78.4152265811471,81.4485934937248,204.895272703575));
#28289=CARTESIAN_POINT('Ctrl Pts',(78.2629901939392,81.5967945814601,204.910763877175));
#28290=CARTESIAN_POINT('Ctrl Pts',(77.9161651020494,81.8217182132772,204.940381086406));
#28291=CARTESIAN_POINT('Ctrl Pts',(77.7265052478057,81.8986978372163,204.953737074714));
#28292=CARTESIAN_POINT('Ctrl Pts',(77.3193282330171,81.9795770677055,204.980571196726));
#28293=CARTESIAN_POINT('Ctrl Pts',(77.1049626836357,81.979067594133,204.995581906058));
#28294=CARTESIAN_POINT('Ctrl Pts',(76.6932320133264,81.8953353051922,205.026109475268));
#28295=CARTESIAN_POINT('Ctrl Pts',(76.4994587495614,81.8145610697187,205.041324794478));
#28296=CARTESIAN_POINT('Ctrl Pts',(76.157008732524,81.5855974798968,205.069981917019));
#28297=CARTESIAN_POINT('Ctrl Pts',(76.0107423572109,81.4409137873655,205.082311936756));
#28298=CARTESIAN_POINT('Ctrl Pts',(75.7748581957499,81.0963025631212,205.110792924539));
#28299=CARTESIAN_POINT('Ctrl Pts',(75.6907226947701,80.8976152834975,205.126320011226));
#28300=CARTESIAN_POINT('Ctrl Pts',(75.6070466851493,80.4869502960989,205.156858029989));
#28301=CARTESIAN_POINT('Ctrl Pts',(75.6051851602486,80.2795082605422,205.171587602031));
#28302=CARTESIAN_POINT('Ctrl Pts',(75.6807397717952,79.8717584247721,205.199175113662));
#28303=CARTESIAN_POINT('Ctrl Pts',(75.7587530067581,79.6756333159173,205.212219109163));
#28304=CARTESIAN_POINT('Ctrl Pts',(75.9869140471254,79.3228268384665,205.242016509498));
#28305=CARTESIAN_POINT('Ctrl Pts',(76.1354151060354,79.1700590426472,205.257540603753));
#28306=CARTESIAN_POINT('Ctrl Pts',(76.4697255012955,78.9401624955558,205.286748139996));
#28307=CARTESIAN_POINT('Ctrl Pts',(76.648829935328,78.8601393255087,205.300223680986));
#28308=CARTESIAN_POINT('Ctrl Pts',(76.8377292359511,78.8141945740679,205.312499998088));
#28309=CARTESIAN_POINT('Ctrl Pts',(76.837729235951,78.8141945740679,205.4));
#28310=CARTESIAN_POINT('Ctrl Pts',(76.7551212011898,78.8342867904583,205.394631412469));
#28311=CARTESIAN_POINT('Ctrl Pts',(76.6740740682798,78.8609712158328,205.389013236702));
#28312=CARTESIAN_POINT('Ctrl Pts',(76.4047721719173,78.9742784392342,205.369104620904));
#28313=CARTESIAN_POINT('Ctrl Pts',(76.2315578549372,79.0906407584965,205.354110083167));
#28314=CARTESIAN_POINT('Ctrl Pts',(75.9350654447631,79.3867132329826,205.323565240702));
#28315=CARTESIAN_POINT('Ctrl Pts',(75.8161553456459,79.5651720045722,205.308308321444));
#28316=CARTESIAN_POINT('Ctrl Pts',(75.6585440861613,79.9494216629153,205.280648746899));
#28317=CARTESIAN_POINT('Ctrl Pts',(75.6179490665698,80.1500757283593,205.268038083199));
#28318=CARTESIAN_POINT('Ctrl Pts',(75.6138721890207,80.5621666080175,205.238911253169));
#28319=CARTESIAN_POINT('Ctrl Pts',(75.6528250702192,80.7696710992104,205.223538073735));
#28320=CARTESIAN_POINT('Ctrl Pts',(75.8095424391573,81.1609318663869,205.193116168863));
#28321=CARTESIAN_POINT('Ctrl Pts',(75.9269208027371,81.340274475958,205.178611880733));
#28322=CARTESIAN_POINT('Ctrl Pts',(76.2187671975469,81.6366838658313,205.152113006099));
#28323=CARTESIAN_POINT('Ctrl Pts',(76.3881892768247,81.7532332382239,205.137868216388));
#28324=CARTESIAN_POINT('Ctrl Pts',(76.7687972806784,81.9196559783247,205.107823171834));
#28325=CARTESIAN_POINT('Ctrl Pts',(76.9776681826639,81.9651407600593,205.092274884239));
#28326=CARTESIAN_POINT('Ctrl Pts',(77.3966940428623,81.9720875330056,205.062811061138));
#28327=CARTESIAN_POINT('Ctrl Pts',(77.6026659915845,81.9351962846408,205.050129378388));
#28328=CARTESIAN_POINT('Ctrl Pts',(77.988098075007,81.7852653846243,205.022251782484));
#28329=CARTESIAN_POINT('Ctrl Pts',(78.1639919457963,81.6740684619583,205.007375993244));
#28330=CARTESIAN_POINT('Ctrl Pts',(78.4640202909783,81.3909710588773,204.977297944441));
#28331=CARTESIAN_POINT('Ctrl Pts',(78.5853362915726,81.2216066863523,204.962372029918));
#28332=CARTESIAN_POINT('Ctrl Pts',(78.7570757738794,80.8457585555339,204.934390309712));
#28333=CARTESIAN_POINT('Ctrl Pts',(78.8057378661131,80.6428520706424,204.921809701669));
#28334=CARTESIAN_POINT('Ctrl Pts',(78.8233675643026,80.2244589851985,204.892469904537));
#28335=CARTESIAN_POINT('Ctrl Pts',(78.7901213237259,80.0130303360736,204.876917034798));
#28336=CARTESIAN_POINT('Ctrl Pts',(78.6459586495334,79.622929673399,204.846793675241));
#28337=CARTESIAN_POINT('Ctrl Pts',(78.5393029184471,79.446832765854,204.832479057667));
#28338=CARTESIAN_POINT('Ctrl Pts',(78.2600541470652,79.1381441568787,204.805795938984));
#28339=CARTESIAN_POINT('Ctrl Pts',(78.0877588221643,79.0105972118158,204.791497598391));
#28340=CARTESIAN_POINT('Ctrl Pts',(77.7059670624353,78.8314620415953,204.761109094792));
#28341=CARTESIAN_POINT('Ctrl Pts',(77.5008174194325,78.7805899862057,204.745710755011));
#28342=CARTESIAN_POINT('Ctrl Pts',(77.1387798153871,78.7634125216628,204.720024948583));
#28343=CARTESIAN_POINT('Ctrl Pts',(76.9859553886663,78.778142488533,204.709633022714));
#28344=CARTESIAN_POINT('Ctrl Pts',(76.8377292359504,78.814194574068,204.7));
#28345=CARTESIAN_POINT('Origin',(77.215862801455,80.368869783441,212.));
#28346=CARTESIAN_POINT('',(76.8377292359511,78.8141945740678,206.1));
#28347=CARTESIAN_POINT('',(76.8377292359511,78.8141945740678,206.012499998088));
#28348=CARTESIAN_POINT('',(76.8377292359511,78.8141945740678,212.));
#28349=CARTESIAN_POINT('Ctrl Pts',(76.8377292359512,78.8141945740679,205.312499998088));
#28350=CARTESIAN_POINT('Ctrl Pts',(76.8460262768778,78.8121765386288,205.313039211866));
#28351=CARTESIAN_POINT('Ctrl Pts',(76.8543419151689,78.8102243289544,205.313581076532));
#28352=CARTESIAN_POINT('Ctrl Pts',(77.0697299280818,78.761476620757,205.327653480417));
#28353=CARTESIAN_POINT('Ctrl Pts',(77.2839912443304,78.7563019461671,205.342540361718));
#28354=CARTESIAN_POINT('Ctrl Pts',(77.6982836699973,78.8291512923048,205.373024072114));
#28355=CARTESIAN_POINT('Ctrl Pts',(77.8946055301384,78.905044242438,205.388317655467));
#28356=CARTESIAN_POINT('Ctrl Pts',(78.2427681657401,79.1251520129856,205.417192960697));
#28357=CARTESIAN_POINT('Ctrl Pts',(78.3923340039078,79.2655685193145,205.429603623653));
#28358=CARTESIAN_POINT('Ctrl Pts',(78.6373109624049,79.6037671547505,205.457786965554));
#28359=CARTESIAN_POINT('Ctrl Pts',(78.7268457821231,79.8007200571218,205.473284214301));
#28360=CARTESIAN_POINT('Ctrl Pts',(78.8212444038845,80.2101508078975,205.503919565077));
#28361=CARTESIAN_POINT('Ctrl Pts',(78.8283330455804,80.4179993675096,205.518768016861));
#28362=CARTESIAN_POINT('Ctrl Pts',(78.7630008966621,80.8265711687446,205.546589925751));
#28363=CARTESIAN_POINT('Ctrl Pts',(78.6906234423817,81.0232560577664,205.559332073145));
#28364=CARTESIAN_POINT('Ctrl Pts',(78.4726526838346,81.3814108215029,205.588861295697));
#28365=CARTESIAN_POINT('Ctrl Pts',(78.3279091400948,81.5385286778803,205.604406232331));
#28366=CARTESIAN_POINT('Ctrl Pts',(77.9921441869454,81.7826739453617,205.634407900906));
#28367=CARTESIAN_POINT('Ctrl Pts',(77.8060708467818,81.8699216507472,205.648614750934));
#28368=CARTESIAN_POINT('Ctrl Pts',(77.4029701473195,81.9719846302046,205.675014110391));
#28369=CARTESIAN_POINT('Ctrl Pts',(77.1889124798798,81.9826756615117,205.689633534107));
#28370=CARTESIAN_POINT('Ctrl Pts',(76.7722099218598,81.9202722643828,205.720071734931));
#28371=CARTESIAN_POINT('Ctrl Pts',(76.5735641031912,81.8491197064306,205.735430751895));
#28372=CARTESIAN_POINT('Ctrl Pts',(76.2199957127401,81.6375193900391,205.764509909028));
#28373=CARTESIAN_POINT('Ctrl Pts',(76.0672719147115,81.5010992773044,205.777073575518));
#28374=CARTESIAN_POINT('Ctrl Pts',(75.8152137785069,81.170926829644,205.804810280769));
#28375=CARTESIAN_POINT('Ctrl Pts',(75.7212557212402,80.978153041104,205.820087658874));
#28376=CARTESIAN_POINT('Ctrl Pts',(75.6155250598987,80.5728204198378,205.850627933799));
#28377=CARTESIAN_POINT('Ctrl Pts',(75.6025781577021,80.3646728092727,205.865598527017));
#28378=CARTESIAN_POINT('Ctrl Pts',(75.6565391648345,79.955266773706,205.893675497214));
#28379=CARTESIAN_POINT('Ctrl Pts',(75.7227718583759,79.7579332428505,205.906177616559));
#28380=CARTESIAN_POINT('Ctrl Pts',(75.9294921770812,79.3940484602969,205.935401965953));
#28381=CARTESIAN_POINT('Ctrl Pts',(76.0699577027409,79.23224710885,205.95095708058));
#28382=CARTESIAN_POINT('Ctrl Pts',(76.399458871065,78.977764839473,205.9811488438));
#28383=CARTESIAN_POINT('Ctrl Pts',(76.5835011456803,78.8850062283669,205.99552604142));
#28384=CARTESIAN_POINT('Ctrl Pts',(76.7992031104156,78.8239456967837,206.009977069679));
#28385=CARTESIAN_POINT('Ctrl Pts',(76.8184288597615,78.8188888793608,206.011245692024));
#28386=CARTESIAN_POINT('Ctrl Pts',(76.837729235951,78.8141945740679,206.012499998088));
#28387=CARTESIAN_POINT('Ctrl Pts',(76.8377292359512,78.8141945740678,206.1));
#28388=CARTESIAN_POINT('Ctrl Pts',(76.7295564051995,78.84050474994,206.092969990001));
#28389=CARTESIAN_POINT('Ctrl Pts',(76.6242071338796,78.8780811547185,206.085521653149));
#28390=CARTESIAN_POINT('Ctrl Pts',(76.3360805833358,79.0164076254402,206.063360472326));
#28391=CARTESIAN_POINT('Ctrl Pts',(76.168093156805,79.1419510224239,206.048179351679));
#28392=CARTESIAN_POINT('Ctrl Pts',(75.886508064799,79.4535233937972,206.0176403473));
#28393=CARTESIAN_POINT('Ctrl Pts',(75.7769098452468,79.6377726232886,206.002583013583));
#28394=CARTESIAN_POINT('Ctrl Pts',(75.639207908886,80.0293590514828,205.975604104429));
#28395=CARTESIAN_POINT('Ctrl Pts',(75.6088938918627,80.231713904417,205.9624099746));
#28396=CARTESIAN_POINT('Ctrl Pts',(75.6258182785655,80.6444400980455,205.932876224462));
#28397=CARTESIAN_POINT('Ctrl Pts',(75.6757309294006,80.8507143613043,205.917401342142));
#28398=CARTESIAN_POINT('Ctrl Pts',(75.8530109775707,81.2333860441182,205.887233633762));
#28399=CARTESIAN_POINT('Ctrl Pts',(75.9790801299804,81.4057287529166,205.873620103953));
#28400=CARTESIAN_POINT('Ctrl Pts',(76.2860429984549,81.6869793327039,205.846374231918));
#28401=CARTESIAN_POINT('Ctrl Pts',(76.4622559443836,81.795058439425,205.831827904456));
#28402=CARTESIAN_POINT('Ctrl Pts',(76.8532605300127,81.9417045723369,205.801460810072));
#28403=CARTESIAN_POINT('Ctrl Pts',(77.0654675101779,81.9759456732983,205.785909593641));
#28404=CARTESIAN_POINT('Ctrl Pts',(77.4830873312372,81.9596700127071,205.757020256091));
#28405=CARTESIAN_POINT('Ctrl Pts',(77.6845014352316,81.9123823242378,205.744664500929));
#28406=CARTESIAN_POINT('Ctrl Pts',(78.0606130127198,81.7434070248921,205.716319616828));
#28407=CARTESIAN_POINT('Ctrl Pts',(78.2313468732561,81.6225539237121,205.701229796181));
#28408=CARTESIAN_POINT('Ctrl Pts',(78.5206962074919,81.3188536149637,205.670677640206));
#28409=CARTESIAN_POINT('Ctrl Pts',(78.6351165714267,81.1375178583068,205.655512666239));
#28410=CARTESIAN_POINT('Ctrl Pts',(78.7830619342441,80.749652677949,205.628180855822));
#28411=CARTESIAN_POINT('Ctrl Pts',(78.8186672663754,80.5482023002402,205.615326470681));
#28412=CARTESIAN_POINT('Ctrl Pts',(78.8126137889458,80.1357667896468,205.58600065032));
#28413=CARTESIAN_POINT('Ctrl Pts',(78.7683677270193,79.9287852247619,205.570573305253));
#28414=CARTESIAN_POINT('Ctrl Pts',(78.6010919413994,79.5402018279054,205.540159145476));
#28415=CARTESIAN_POINT('Ctrl Pts',(78.4783753241339,79.3631142207569,205.526058225016));
#28416=CARTESIAN_POINT('Ctrl Pts',(78.1772529375327,79.0736830296676,205.49905332579));
#28417=CARTESIAN_POINT('Ctrl Pts',(78.0041426461427,78.9616202196116,205.484642434675));
#28418=CARTESIAN_POINT('Ctrl Pts',(77.6178428989278,78.8057077498253,205.45441458712));
#28419=CARTESIAN_POINT('Ctrl Pts',(77.407112893485,78.7662143562072,205.438859041677));
#28420=CARTESIAN_POINT('Ctrl Pts',(77.0741725852005,78.7705959032636,205.415651318138));
#28421=CARTESIAN_POINT('Ctrl Pts',(76.9544243197534,78.7858115858727,205.407583860016));
#28422=CARTESIAN_POINT('Ctrl Pts',(76.837729235951,78.8141945740679,205.4));
#28423=CARTESIAN_POINT('Origin',(77.215862801455,80.368869783441,212.));
#28424=CARTESIAN_POINT('',(76.8377292359514,78.8141945740678,206.8));
#28425=CARTESIAN_POINT('',(76.8377292359507,78.8141945740679,206.712499998088));
#28426=CARTESIAN_POINT('',(76.8377292359511,78.8141945740678,212.));
#28427=CARTESIAN_POINT('Ctrl Pts',(76.837729235951,78.8141945740679,206.012499998088));
#28428=CARTESIAN_POINT('Ctrl Pts',(77.0257911158799,78.7684535030299,206.024721892321));
#28429=CARTESIAN_POINT('Ctrl Pts',(77.2207820174295,78.7571595604737,206.038134868243));
#28430=CARTESIAN_POINT('Ctrl Pts',(77.6211916289537,78.8069485066445,206.067174350675));
#28431=CARTESIAN_POINT('Ctrl Pts',(77.822008813833,78.8733824400182,206.082588569851));
#28432=CARTESIAN_POINT('Ctrl Pts',(78.1808309533484,79.0765901706023,206.111863297245));
#28433=CARTESIAN_POINT('Ctrl Pts',(78.3366632510614,79.2091600612225,206.124647668695));
#28434=CARTESIAN_POINT('Ctrl Pts',(78.5965453122727,79.5329154385169,206.152064544514));
#28435=CARTESIAN_POINT('Ctrl Pts',(78.6951616979899,79.7233173028714,206.16725414456));
#28436=CARTESIAN_POINT('Ctrl Pts',(78.8108803488985,80.1263876126478,206.197806251788));
#28437=CARTESIAN_POINT('Ctrl Pts',(78.8288516435248,80.3346609153489,206.212872334023));
#28438=CARTESIAN_POINT('Ctrl Pts',(78.7845858054451,80.744711603189,206.241162051983));
#28439=CARTESIAN_POINT('Ctrl Pts',(78.7234945932347,80.9426271118811,206.253538742612));
#28440=CARTESIAN_POINT('Ctrl Pts',(78.5262915101812,81.3112226257922,206.282498311826));
#28441=CARTESIAN_POINT('Ctrl Pts',(78.3895467147799,81.4768849140947,206.298051581849));
#28442=CARTESIAN_POINT('Ctrl Pts',(78.0655682483538,81.7399592826122,206.328384671391));
#28443=CARTESIAN_POINT('Ctrl Pts',(77.8833641244146,81.8373277503449,206.342897024088));
#28444=CARTESIAN_POINT('Ctrl Pts',(77.4852406403898,81.9602007489264,206.370081645795));
#28445=CARTESIAN_POINT('Ctrl Pts',(77.2723350705081,81.981867077468,206.383812602008));
#28446=CARTESIAN_POINT('Ctrl Pts',(76.8522474805038,81.9410988556117,206.414044114645));
#28447=CARTESIAN_POINT('Ctrl Pts',(76.6492066580898,81.8798372037296,206.429507893021));
#28448=CARTESIAN_POINT('Ctrl Pts',(76.2847596732123,81.68575826866,206.458989064702));
#28449=CARTESIAN_POINT('Ctrl Pts',(76.1255499030091,81.5572800398929,206.472088823458));
#28450=CARTESIAN_POINT('Ctrl Pts',(75.85739009848,81.2404453326028,206.499158009755));
#28451=CARTESIAN_POINT('Ctrl Pts',(75.7538709443149,81.0527025114772,206.514243701397));
#28452=CARTESIAN_POINT('Ctrl Pts',(75.6275459159743,80.6523209837157,206.54478808149));
#28453=CARTESIAN_POINT('Ctrl Pts',(75.6041976977911,80.4440461585913,206.559946930229));
#28454=CARTESIAN_POINT('Ctrl Pts',(75.6381324494241,80.0333725344831,206.58845881589));
#28455=CARTESIAN_POINT('Ctrl Pts',(75.693835156032,79.8348083827527,206.600780800812));
#28456=CARTESIAN_POINT('Ctrl Pts',(75.8809780090442,79.4613591540993,206.629454150093));
#28457=CARTESIAN_POINT('Ctrl Pts',(76.0136924153775,79.2917189964761,206.644995130815));
#28458=CARTESIAN_POINT('Ctrl Pts',(76.3316166364797,79.0197207198143,206.675458218143));
#28459=CARTESIAN_POINT('Ctrl Pts',(76.5117607144455,78.9175350303539,206.690104463321));
#28460=CARTESIAN_POINT('Ctrl Pts',(76.7496405829934,78.8376206949813,206.706674488704));
#28461=CARTESIAN_POINT('Ctrl Pts',(76.7934786972824,78.824957345521,206.70962421378));
#28462=CARTESIAN_POINT('Ctrl Pts',(76.8377292359504,78.814194574068,206.712499998088));
#28463=CARTESIAN_POINT('Ctrl Pts',(76.8377292359517,78.8141945740677,206.8));
#28464=CARTESIAN_POINT('Ctrl Pts',(76.7031628343352,78.8469242869579,206.791254706544));
#28465=CARTESIAN_POINT('Ctrl Pts',(76.573192662753,78.8970312216183,206.781876896184));
#28466=CARTESIAN_POINT('Ctrl Pts',(76.2676427912773,79.0633108488901,206.757389339445));
#28467=CARTESIAN_POINT('Ctrl Pts',(76.1055401402883,79.1980677513917,206.74205470168));
#28468=CARTESIAN_POINT('Ctrl Pts',(75.8401590437235,79.5248060945437,206.711606738352));
#28469=CARTESIAN_POINT('Ctrl Pts',(75.7404483387497,79.7144923942664,206.69679714349));
#28470=CARTESIAN_POINT('Ctrl Pts',(75.6233815825307,80.1132492705014,206.670545557463));
#28471=CARTESIAN_POINT('Ctrl Pts',(75.6037754590442,80.3176208162215,206.656411580955));
#28472=CARTESIAN_POINT('Ctrl Pts',(75.643046219008,80.7306773491343,206.626469338703));
#28473=CARTESIAN_POINT('Ctrl Pts',(75.7045291494201,80.9350293292451,206.610931265655));
#28474=CARTESIAN_POINT('Ctrl Pts',(75.9019114114379,81.3052993341646,206.58129581519));
#28475=CARTESIAN_POINT('Ctrl Pts',(76.0347618582989,81.468120535608,206.568444632706));
#28476=CARTESIAN_POINT('Ctrl Pts',(76.3536451345256,81.7323115455285,206.540714377177));
#28477=CARTESIAN_POINT('Ctrl Pts',(76.5360356092322,81.8318100281579,206.525911692908));
#28478=CARTESIAN_POINT('Ctrl Pts',(76.9361502253573,81.9586904897149,206.495312351129));
#28479=CARTESIAN_POINT('Ctrl Pts',(77.1510285772583,81.9818164417919,206.479802083691));
#28480=CARTESIAN_POINT('Ctrl Pts',(77.5668155004734,81.9431233309061,206.45150059773));
#28481=CARTESIAN_POINT('Ctrl Pts',(77.7640021649421,81.88577224502,206.439131629642));
#28482=CARTESIAN_POINT('Ctrl Pts',(78.130613908673,81.698012588912,206.410342008544));
#28483=CARTESIAN_POINT('Ctrl Pts',(78.2956834699523,81.5677700607989,206.395078184758));
#28484=CARTESIAN_POINT('Ctrl Pts',(78.5691662141335,81.2484118562036,206.364574506118));
#28485=CARTESIAN_POINT('Ctrl Pts',(78.6737920676496,81.0613408752536,206.349637353839));
#28486=CARTESIAN_POINT('Ctrl Pts',(78.8010612081228,80.6660762385,206.323023500772));
#28487=CARTESIAN_POINT('Ctrl Pts',(78.8259728468762,80.4627345162427,206.309396880066));
#28488=CARTESIAN_POINT('Ctrl Pts',(78.7978271852326,80.049796452476,206.279654746401));
#28489=CARTESIAN_POINT('Ctrl Pts',(78.7420885864796,79.8444095707088,206.264142339503));
#28490=CARTESIAN_POINT('Ctrl Pts',(78.5546369896886,79.467926160763,206.234237794231));
#28491=CARTESIAN_POINT('Ctrl Pts',(78.4251473336631,79.3004044864736,206.221047935949));
#28492=CARTESIAN_POINT('Ctrl Pts',(78.1121843959568,79.0276791522115,206.193556989518));
#28493=CARTESIAN_POINT('Ctrl Pts',(77.9328334352432,78.9238435470682,206.178878077657));
#28494=CARTESIAN_POINT('Ctrl Pts',(77.5371555125614,78.7870041470317,206.148385019757));
#28495=CARTESIAN_POINT('Ctrl Pts',(77.3235437267372,78.7582924327972,206.132848863259));
#28496=CARTESIAN_POINT('Ctrl Pts',(77.0183726466444,78.7784185326988,206.111907084985));
#28497=CARTESIAN_POINT('Ctrl Pts',(76.9271049840608,78.792456290664,206.10580841232));
#28498=CARTESIAN_POINT('Ctrl Pts',(76.8377292359512,78.8141945740679,206.1));
#28499=CARTESIAN_POINT('Origin',(77.215862801455,80.368869783441,212.));
#28500=CARTESIAN_POINT('',(76.8377292359514,78.8141945740678,207.5));
#28501=CARTESIAN_POINT('',(76.8377292359509,78.8141945740679,207.412499998088));
#28502=CARTESIAN_POINT('',(76.8377292359511,78.8141945740678,212.));
#28503=CARTESIAN_POINT('Ctrl Pts',(76.8377292359504,78.814194574068,206.712499998088));
#28504=CARTESIAN_POINT('Ctrl Pts',(76.997035119303,78.775447637528,206.722853077924));
#28505=CARTESIAN_POINT('Ctrl Pts',(77.161571312679,78.7613499102684,206.734077498517));
#28506=CARTESIAN_POINT('Ctrl Pts',(77.5358324712544,78.7871044077927,206.760794493322));
#28507=CARTESIAN_POINT('Ctrl Pts',(77.7410463522403,78.8429139599381,206.776298554896));
#28508=CARTESIAN_POINT('Ctrl Pts',(78.1112826620142,79.0274325164619,206.805988832192));
#28509=CARTESIAN_POINT('Ctrl Pts',(78.2740289188509,79.1517242309619,206.819498922382));
#28510=CARTESIAN_POINT('Ctrl Pts',(78.5506079792258,79.4613825138365,206.846204737318));
#28511=CARTESIAN_POINT('Ctrl Pts',(78.6590777580625,79.646263514295,206.861172978244));
#28512=CARTESIAN_POINT('Ctrl Pts',(78.7962154838579,80.0435947151159,206.891687570791));
#28513=CARTESIAN_POINT('Ctrl Pts',(78.8250902676227,80.2517283691258,206.906931654772));
#28514=CARTESIAN_POINT('Ctrl Pts',(78.8017416654103,80.6629722531716,206.935666371369));
#28515=CARTESIAN_POINT('Ctrl Pts',(78.7514710624391,80.8622346739487,206.948015477938));
#28516=CARTESIAN_POINT('Ctrl Pts',(78.5745460292897,81.2404883153497,206.976391813275));
#28517=CARTESIAN_POINT('Ctrl Pts',(78.4460225886296,81.4140566814621,206.991909535085));
#28518=CARTESIAN_POINT('Ctrl Pts',(78.134466906013,81.6949440521815,207.022484290718));
#28519=CARTESIAN_POINT('Ctrl Pts',(77.9565350789733,81.8019592720384,207.037257020441));
#28520=CARTESIAN_POINT('Ctrl Pts',(77.5671906874959,81.9436937733108,207.064928277103));
#28521=CARTESIAN_POINT('Ctrl Pts',(77.3591707612842,81.9760362641169,207.077855801554));
#28522=CARTESIAN_POINT('Ctrl Pts',(76.9397003487069,81.9589452951304,207.10755870483));
#28523=CARTESIAN_POINT('Ctrl Pts',(76.7324607878316,81.9086490494024,207.123091481919));
#28524=CARTESIAN_POINT('Ctrl Pts',(76.356505160668,81.7337516094761,207.152984720812));
#28525=CARTESIAN_POINT('Ctrl Pts',(76.1901980973244,81.6135807730318,207.166985795827));
#28526=CARTESIAN_POINT('Ctrl Pts',(75.9053941660867,81.3110660341237,207.193327219246));
#28527=CARTESIAN_POINT('Ctrl Pts',(75.7921319860464,81.1291329059222,207.208169185998));
#28528=CARTESIAN_POINT('Ctrl Pts',(75.6444236432481,80.7350919151538,207.238632823335));
#28529=CARTESIAN_POINT('Ctrl Pts',(75.6101008392802,80.5272387588863,207.25395091757));
#28530=CARTESIAN_POINT('Ctrl Pts',(75.6230304341367,80.1155061082904,207.282899810908));
#28531=CARTESIAN_POINT('Ctrl Pts',(75.668038150444,79.915511146734,207.295356861781));
#28532=CARTESIAN_POINT('Ctrl Pts',(75.8349977199822,79.5326927281716,207.323437427555));
#28533=CARTESIAN_POINT('Ctrl Pts',(75.9593452818444,79.3554057433861,207.33892213344));
#28534=CARTESIAN_POINT('Ctrl Pts',(76.2644868922184,79.0660278791462,207.369586086494));
#28535=CARTESIAN_POINT('Ctrl Pts',(76.4401486419303,78.9543692729348,207.3844728786));
#28536=CARTESIAN_POINT('Ctrl Pts',(76.6993146523219,78.8528307943672,207.403254352416));
#28537=CARTESIAN_POINT('Ctrl Pts',(76.7679808517075,78.8311590210875,207.407967142331));
#28538=CARTESIAN_POINT('Ctrl Pts',(76.8377292359507,78.814194574068,207.412499998088));
#28539=CARTESIAN_POINT('Ctrl Pts',(76.8377292359517,78.8141945740677,207.5));
#28540=CARTESIAN_POINT('Ctrl Pts',(76.6777981233889,78.8530935810524,207.48960628734));
#28541=CARTESIAN_POINT('Ctrl Pts',(76.5246335080535,78.9164726848852,207.47833689724));
#28542=CARTESIAN_POINT('Ctrl Pts',(76.2044243933626,79.111483892041,207.451629555803));
#28543=CARTESIAN_POINT('Ctrl Pts',(76.0484270350896,79.2548152912046,207.436185205297));
#28544=CARTESIAN_POINT('Ctrl Pts',(75.7989033333978,79.5958868983958,207.405851928815));
#28545=CARTESIAN_POINT('Ctrl Pts',(75.7088299834789,79.7908829252769,207.391921163592));
#28546=CARTESIAN_POINT('Ctrl Pts',(75.6120532891954,80.1967064537015,207.364835845637));
#28547=CARTESIAN_POINT('Ctrl Pts',(75.6032112991938,80.4028991933799,207.350379237481));
#28548=CARTESIAN_POINT('Ctrl Pts',(75.6647703143932,80.8152443372814,207.320103312222));
#28549=CARTESIAN_POINT('Ctrl Pts',(75.737685014966,81.0170576733383,207.304548105169));
#28550=CARTESIAN_POINT('Ctrl Pts',(75.9545984511083,81.3746174799975,207.275476612147));
#28551=CARTESIAN_POINT('Ctrl Pts',(76.0941610081724,81.5282219652729,207.263055990249));
#28552=CARTESIAN_POINT('Ctrl Pts',(76.4248741664475,81.7749838042379,207.234855263202));
#28553=CARTESIAN_POINT('Ctrl Pts',(76.6131380772798,81.8653711679294,207.219828377068));
#28554=CARTESIAN_POINT('Ctrl Pts',(77.0188179295303,81.9708193125118,207.189279004408));
#28555=CARTESIAN_POINT('Ctrl Pts',(77.2329191960042,81.9828143537899,207.174051315461));
#28556=CARTESIAN_POINT('Ctrl Pts',(77.6439443479865,81.9238277299733,207.146499085306));
#28557=CARTESIAN_POINT('Ctrl Pts',(77.8374137083549,81.8571059993959,207.13381639049));
#28558=CARTESIAN_POINT('Ctrl Pts',(78.1947768040688,81.6516537639493,207.104623754626));
#28559=CARTESIAN_POINT('Ctrl Pts',(78.3540002206048,81.5127417182456,207.089231765731));
#28560=CARTESIAN_POINT('Ctrl Pts',(78.6118112428972,81.1790752348933,207.058834239073));
#28561=CARTESIAN_POINT('Ctrl Pts',(78.7068414276177,80.9869296971543,207.044483726747));
#28562=CARTESIAN_POINT('Ctrl Pts',(78.8142904703869,80.5848573721532,207.01784809846));
#28563=CARTESIAN_POINT('Ctrl Pts',(78.828767629234,80.3795513980379,207.003551427495));
#28564=CARTESIAN_POINT('Ctrl Pts',(78.7789410778507,79.9667873192257,206.97344800168));
#28565=CARTESIAN_POINT('Ctrl Pts',(78.7120246101494,79.7635618210616,206.957896106856));
#28566=CARTESIAN_POINT('Ctrl Pts',(78.5053254270433,79.399274287447,206.92852396573));
#28567=CARTESIAN_POINT('Ctrl Pts',(78.3692935007023,79.2408549348209,206.91591869202));
#28568=CARTESIAN_POINT('Ctrl Pts',(78.0447982122093,78.9848685281713,206.887963942756));
#28569=CARTESIAN_POINT('Ctrl Pts',(77.859585667051,78.8896185850703,206.873050885631));
#28570=CARTESIAN_POINT('Ctrl Pts',(77.455439567366,78.7724342951044,206.84236822745));
#28571=CARTESIAN_POINT('Ctrl Pts',(77.239477261348,78.7547193693666,206.826893045004));
#28572=CARTESIAN_POINT('Ctrl Pts',(76.9627741045119,78.7877137527686,206.808207135088));
#28573=CARTESIAN_POINT('Ctrl Pts',(76.899771582067,78.7991044167105,206.804032050474));
#28574=CARTESIAN_POINT('Ctrl Pts',(76.8377292359517,78.8141945740677,206.8));
#28575=CARTESIAN_POINT('Origin',(77.215862801455,80.368869783441,212.));
#28576=CARTESIAN_POINT('',(76.8377292359511,78.8141945740678,208.2));
#28577=CARTESIAN_POINT('',(76.8377292359511,78.8141945740679,208.112499998088));
#28578=CARTESIAN_POINT('',(76.8377292359511,78.8141945740678,212.));
#28579=CARTESIAN_POINT('Ctrl Pts',(76.8377292359507,78.814194574068,207.412499998088));
#28580=CARTESIAN_POINT('Ctrl Pts',(76.9684916976914,78.7823900687964,207.420998078495));
#28581=CARTESIAN_POINT('Ctrl Pts',(77.1029799634108,78.7671439496196,207.430096346542));
#28582=CARTESIAN_POINT('Ctrl Pts',(77.4498635404948,78.7719712833825,207.454468549654));
#28583=CARTESIAN_POINT('Ctrl Pts',(77.658907610699,78.8169227172997,207.470018020224));
#28584=CARTESIAN_POINT('Ctrl Pts',(78.0400365892561,78.9824124890444,207.500080392696));
#28585=CARTESIAN_POINT('Ctrl Pts',(78.2097935453799,79.0985650149274,207.514340479469));
#28586=CARTESIAN_POINT('Ctrl Pts',(78.5024133351802,79.394297461228,207.540879594097));
#28587=CARTESIAN_POINT('Ctrl Pts',(78.6202345840811,79.5733568839449,207.555338093668));
#28588=CARTESIAN_POINT('Ctrl Pts',(78.777931269987,79.9642816395426,207.585753067982));
#28589=CARTESIAN_POINT('Ctrl Pts',(78.817392852367,80.1717416404156,207.601131861497));
#28590=CARTESIAN_POINT('Ctrl Pts',(78.8142889134598,80.5838686624257,207.630278018563));
#28591=CARTESIAN_POINT('Ctrl Pts',(78.7741757834228,80.7845972519932,207.642908972068));
#28592=CARTESIAN_POINT('Ctrl Pts',(78.6174978654381,81.169200555034,207.670537125653));
#28593=CARTESIAN_POINT('Ctrl Pts',(78.4990185776205,81.3479424802035,207.685785579469));
#28594=CARTESIAN_POINT('Ctrl Pts',(78.2032078888692,81.6447597587104,207.716331966708));
#28595=CARTESIAN_POINT('Ctrl Pts',(78.0302282929965,81.7615583376688,207.731336090101));
#28596=CARTESIAN_POINT('Ctrl Pts',(77.6501511969106,81.922511869429,207.759486234002));
#28597=CARTESIAN_POINT('Ctrl Pts',(77.4468528725997,81.9654469115731,207.771937330493));
#28598=CARTESIAN_POINT('Ctrl Pts',(77.0285798523411,81.9720006089835,207.801071691852));
#28599=CARTESIAN_POINT('Ctrl Pts',(76.8177006931565,81.9330156752873,207.816627250096));
#28600=CARTESIAN_POINT('Ctrl Pts',(76.4309339806257,81.7779981310026,207.846869426193));
#28601=CARTESIAN_POINT('Ctrl Pts',(76.2575180542302,81.6663189293149,207.861293839571));
#28602=CARTESIAN_POINT('Ctrl Pts',(75.9558238922242,81.3776835173705,207.888322434105));
#28603=CARTESIAN_POINT('Ctrl Pts',(75.8327778251431,81.2010625880721,207.902372454566));
#28604=CARTESIAN_POINT('Ctrl Pts',(75.6645181565862,80.8130528558924,207.932762924489));
#28605=CARTESIAN_POINT('Ctrl Pts',(75.6197177765441,80.606133740526,207.948195397308));
#28606=CARTESIAN_POINT('Ctrl Pts',(75.6126023097434,80.1936661904108,207.977541788595));
#28607=CARTESIAN_POINT('Ctrl Pts',(75.6476879821394,79.9921297253142,207.990425839145));
#28608=CARTESIAN_POINT('Ctrl Pts',(75.7946267510987,79.6038939155045,208.017723220263));
#28609=CARTESIAN_POINT('Ctrl Pts',(75.9085760800567,79.4222656484567,208.032878078399));
#28610=CARTESIAN_POINT('Ctrl Pts',(76.1971711430594,79.1177820053721,208.06342989267));
#28611=CARTESIAN_POINT('Ctrl Pts',(76.3676404318543,78.9964647868572,208.078529127192));
#28612=CARTESIAN_POINT('Ctrl Pts',(76.6472679322046,78.8699976331339,208.099644936608));
#28613=CARTESIAN_POINT('Ctrl Pts',(76.7414060787578,78.8376226307131,208.106240082789));
#28614=CARTESIAN_POINT('Ctrl Pts',(76.8377292359511,78.8141945740679,208.112499998088));
#28615=CARTESIAN_POINT('Ctrl Pts',(76.8377292359511,78.8141945740679,208.2));
#28616=CARTESIAN_POINT('Ctrl Pts',(76.6496783488809,78.8599329713841,208.187778820179));
#28617=CARTESIAN_POINT('Ctrl Pts',(76.4713255474108,78.9394459630036,208.174368609384));
#28618=CARTESIAN_POINT('Ctrl Pts',(76.137386981879,79.1682907824281,208.145233638291));
#28619=CARTESIAN_POINT('Ctrl Pts',(75.9886585518949,79.3207877535425,208.12971118779));
#28620=CARTESIAN_POINT('Ctrl Pts',(75.759870735986,79.6732601904406,208.099897548496));
#28621=CARTESIAN_POINT('Ctrl Pts',(75.6815085293303,79.869351520945,208.08683239959));
#28622=CARTESIAN_POINT('Ctrl Pts',(75.6053274043631,80.2770487558979,208.05925941127));
#28623=CARTESIAN_POINT('Ctrl Pts',(75.6068699396097,80.4844616896433,208.044537398159));
#28624=CARTESIAN_POINT('Ctrl Pts',(75.6898899419757,80.8951932736331,208.014005965699));
#28625=CARTESIAN_POINT('Ctrl Pts',(75.7736942510371,81.0939820127701,207.998477397809));
#28626=CARTESIAN_POINT('Ctrl Pts',(76.0090201561273,81.438982522867,207.969978448938));
#28627=CARTESIAN_POINT('Ctrl Pts',(76.1550860915338,81.5839284341693,207.957650674205));
#28628=CARTESIAN_POINT('Ctrl Pts',(76.4971871757524,81.813428594404,207.929006967727));
#28629=CARTESIAN_POINT('Ctrl Pts',(76.6908018298294,81.8944966741833,207.913796722969));
#28630=CARTESIAN_POINT('Ctrl Pts',(77.1023676486615,81.9788871083084,207.883267196219));
#28631=CARTESIAN_POINT('Ctrl Pts',(77.3167345151289,81.9797418516438,207.868249316131));
#28632=CARTESIAN_POINT('Ctrl Pts',(77.7240333610203,81.899519390134,207.841393204133));
#28633=CARTESIAN_POINT('Ctrl Pts',(77.9138050455682,81.8228515260244,207.828062625307));
#28634=CARTESIAN_POINT('Ctrl Pts',(78.260956467854,81.5985201212301,207.798458022898));
#28635=CARTESIAN_POINT('Ctrl Pts',(78.4134136759075,81.4505971161129,207.78296920396));
#28636=CARTESIAN_POINT('Ctrl Pts',(78.6526610489904,81.1037890896475,207.752889101302));
#28637=CARTESIAN_POINT('Ctrl Pts',(78.7368891754549,80.9082538630004,207.739427260937));
#28638=CARTESIAN_POINT('Ctrl Pts',(78.8234897447539,80.5014693206156,207.712098492507));
#28639=CARTESIAN_POINT('Ctrl Pts',(78.8272266223828,80.2946102882477,207.69750670218));
#28640=CARTESIAN_POINT('Ctrl Pts',(78.7550916221485,79.8829233435445,207.667095158804));
#28641=CARTESIAN_POINT('Ctrl Pts',(78.6767972232593,79.6825291409411,207.651547792439));
#28642=CARTESIAN_POINT('Ctrl Pts',(78.4507725554193,79.3311185265315,207.622754965691));
#28643=CARTESIAN_POINT('Ctrl Pts',(78.30801310448,79.1817987667151,207.610419838608));
#28644=CARTESIAN_POINT('Ctrl Pts',(77.9716950288724,78.9434768952379,207.581999939645));
#28645=CARTESIAN_POINT('Ctrl Pts',(77.7807557196506,78.8576117586452,207.566878555098));
#28646=CARTESIAN_POINT('Ctrl Pts',(77.3720576160872,78.7624273203424,207.536328402515));
#28647=CARTESIAN_POINT('Ctrl Pts',(77.1577516537931,78.755884884644,207.521198177244));
#28648=CARTESIAN_POINT('Ctrl Pts',(76.9111913140107,78.7976925211682,207.504802201921));
#28649=CARTESIAN_POINT('Ctrl Pts',(76.8742863805139,78.8053030169537,207.502375800744));
#28650=CARTESIAN_POINT('Ctrl Pts',(76.8377292359517,78.8141945740677,207.5));
#28651=CARTESIAN_POINT('Origin',(77.215862801455,80.368869783441,212.));
#28652=CARTESIAN_POINT('',(76.8377292359511,78.8141945740679,208.9));
#28653=CARTESIAN_POINT('',(76.8377292359513,78.8141945740678,208.812499998088));
#28654=CARTESIAN_POINT('',(76.8377292359511,78.8141945740678,212.));
#28655=CARTESIAN_POINT('Ctrl Pts',(76.8377292359511,78.8141945740679,208.112499998088));
#28656=CARTESIAN_POINT('Ctrl Pts',(76.9396630831313,78.7894018656955,208.11912454475));
#28657=CARTESIAN_POINT('Ctrl Pts',(77.0439972318632,78.7746397691921,208.126122696795));
#28658=CARTESIAN_POINT('Ctrl Pts',(77.3620334959564,78.7613966957854,208.148105831678));
#28659=CARTESIAN_POINT('Ctrl Pts',(77.574385754742,78.7950926560753,208.163656037733));
#28660=CARTESIAN_POINT('Ctrl Pts',(77.9658637169711,78.9407742712014,208.194036482534));
#28661=CARTESIAN_POINT('Ctrl Pts',(78.1423918359513,79.0484372526846,208.208596333037));
#28662=CARTESIAN_POINT('Ctrl Pts',(78.4499527939014,79.3288435688161,208.235866747699));
#28663=CARTESIAN_POINT('Ctrl Pts',(78.5763638298165,79.5007032173591,208.249434493321));
#28664=CARTESIAN_POINT('Ctrl Pts',(78.754662616906,79.8827631611168,208.279576414897));
#28665=CARTESIAN_POINT('Ctrl Pts',(78.805155940984,80.088956282147,208.29505555474));
#28666=CARTESIAN_POINT('Ctrl Pts',(78.8231964431696,80.5017076070801,208.324610319086));
#28667=CARTESIAN_POINT('Ctrl Pts',(78.7934223240728,80.7041582210938,208.337843799841));
#28668=CARTESIAN_POINT('Ctrl Pts',(78.6567644858968,81.0961177626275,208.364786426685));
#28669=CARTESIAN_POINT('Ctrl Pts',(78.5476612347784,81.2806560417358,208.379832208013));
#28670=CARTESIAN_POINT('Ctrl Pts',(78.2668783640649,81.5930182716591,208.410368670172));
#28671=CARTESIAN_POINT('Ctrl Pts',(78.0991775394105,81.7190355748876,208.425558535636));
#28672=CARTESIAN_POINT('Ctrl Pts',(77.7282312102709,81.8983015302319,208.454149120467));
#28673=CARTESIAN_POINT('Ctrl Pts',(77.5291678402495,81.9511212129701,208.466471027369));
#28674=CARTESIAN_POINT('Ctrl Pts',(77.112500469628,81.9797377129393,208.495040709726));
#28675=CARTESIAN_POINT('Ctrl Pts',(76.898754559665,81.9515872121988,208.51057474579));
#28676=CARTESIAN_POINT('Ctrl Pts',(76.5026180724941,81.8157460596159,208.541079426116));
#28677=CARTESIAN_POINT('Ctrl Pts',(76.3229558484872,81.7123439487735,208.555771231337));
#28678=CARTESIAN_POINT('Ctrl Pts',(76.0093919016011,81.4404794011624,208.583286585955));
#28679=CARTESIAN_POINT('Ctrl Pts',(75.8795605854027,81.27343750618,208.596438422272));
#28680=CARTESIAN_POINT('Ctrl Pts',(75.6910960792052,80.8975801057865,208.626316069202));
#28681=CARTESIAN_POINT('Ctrl Pts',(75.6347740023039,80.692291073723,208.641831598217));
#28682=CARTESIAN_POINT('Ctrl Pts',(75.6055013609186,80.2793368025846,208.671594301038));
#28683=CARTESIAN_POINT('Ctrl Pts',(75.6298734058512,80.0758930474358,208.68526881607));
#28684=CARTESIAN_POINT('Ctrl Pts',(75.7561026578783,79.6802677912866,208.711845979796));
#28685=CARTESIAN_POINT('Ctrl Pts',(75.860229790237,79.492923688012,208.726770579827));
#28686=CARTESIAN_POINT('Ctrl Pts',(76.1328946305887,79.1728025539968,208.757269533244));
#28687=CARTESIAN_POINT('Ctrl Pts',(76.2976668473919,79.0420961464191,208.772541030412));
#28688=CARTESIAN_POINT('Ctrl Pts',(76.5957546958503,78.8884667952882,208.795998086802));
#28689=CARTESIAN_POINT('Ctrl Pts',(76.7148672649924,78.8440774942195,208.804515360187));
#28690=CARTESIAN_POINT('Ctrl Pts',(76.8377292359514,78.8141945740678,208.812499998088));
#28691=CARTESIAN_POINT('Ctrl Pts',(76.837729235951,78.8141945740679,208.9));
#28692=CARTESIAN_POINT('Ctrl Pts',(76.8191600495721,78.8187110368066,208.898793213));
#28693=CARTESIAN_POINT('Ctrl Pts',(76.8006598466345,78.8235630882186,208.897573167653));
#28694=CARTESIAN_POINT('Ctrl Pts',(76.5856257667561,78.8841065309996,208.883183400459));
#28695=CARTESIAN_POINT('Ctrl Pts',(76.4014766339768,78.9765868869151,208.868814576868));
#28696=CARTESIAN_POINT('Ctrl Pts',(76.0716504374976,79.2305489188511,208.838631864517));
#28697=CARTESIAN_POINT('Ctrl Pts',(75.9309645086107,79.3921155504159,208.823076943288));
#28698=CARTESIAN_POINT('Ctrl Pts',(75.7236729500161,79.7557136693539,208.793836898622));
#28699=CARTESIAN_POINT('Ctrl Pts',(75.657130075,79.953013318426,208.781324975927));
#28700=CARTESIAN_POINT('Ctrl Pts',(75.6025894183993,80.362378866944,208.753260863177));
#28701=CARTESIAN_POINT('Ctrl Pts',(75.6152367173269,80.5705151760514,208.738296233638));
#28702=CARTESIAN_POINT('Ctrl Pts',(75.7203694459341,80.9759750235647,208.70775724856));
#28703=CARTESIAN_POINT('Ctrl Pts',(75.8140473721468,81.1688867810982,208.692474922603));
#28704=CARTESIAN_POINT('Ctrl Pts',(76.065636006685,81.4994404471978,208.66471929837));
#28705=CARTESIAN_POINT('Ctrl Pts',(76.2181757101933,81.6360911709214,208.652166546734));
#28706=CARTESIAN_POINT('Ctrl Pts',(76.5714307894876,81.8481880514375,208.623099133227));
#28707=CARTESIAN_POINT('Ctrl Pts',(76.7699443474843,81.9196185486146,208.607743673018));
#28708=CARTESIAN_POINT('Ctrl Pts',(77.1865225688845,81.9826337295144,208.577301630105));
#28709=CARTESIAN_POINT('Ctrl Pts',(77.4005921695774,81.9722594527818,208.562653369994));
#28710=CARTESIAN_POINT('Ctrl Pts',(77.8038082113088,81.8708052628951,208.536278579317));
#28711=CARTESIAN_POINT('Ctrl Pts',(77.9899853334896,81.783852779215,208.522081119817));
#28712=CARTESIAN_POINT('Ctrl Pts',(78.3260756228065,81.5402632488109,208.492090273253));
#28713=CARTESIAN_POINT('Ctrl Pts',(78.471043211573,81.3833983407653,208.476546255731));
#28714=CARTESIAN_POINT('Ctrl Pts',(78.689613075432,81.0255537745091,208.447001053133));
#28715=CARTESIAN_POINT('Ctrl Pts',(78.7623199526234,80.8289024317685,208.434243365705));
#28716=CARTESIAN_POINT('Ctrl Pts',(78.8282550590881,80.4203772188331,208.406435148202));
#28717=CARTESIAN_POINT('Ctrl Pts',(78.8214758388479,80.2125490428189,208.39159347277));
#28718=CARTESIAN_POINT('Ctrl Pts',(78.7277105333233,79.8030377521981,208.360963329375));
#28719=CARTESIAN_POINT('Ctrl Pts',(78.6384938779096,79.6059784248178,208.345464023115));
#28720=CARTESIAN_POINT('Ctrl Pts',(78.3940524213567,79.2673983913106,208.317262886865));
#28721=CARTESIAN_POINT('Ctrl Pts',(78.2446827883486,79.1267307472499,208.304859305263));
#28722=CARTESIAN_POINT('Ctrl Pts',(77.8968581088172,78.9060952802595,208.275996829927));
#28723=CARTESIAN_POINT('Ctrl Pts',(77.70068443458,78.8299098716014,208.260707620031));
#28724=CARTESIAN_POINT('Ctrl Pts',(77.2865362487069,78.7564111077173,208.230220688716));
#28725=CARTESIAN_POINT('Ctrl Pts',(77.0722643830667,78.7612479163064,208.215326142416));
#28726=CARTESIAN_POINT('Ctrl Pts',(76.8559773625412,78.8098410641186,208.201187661587));
#28727=CARTESIAN_POINT('Ctrl Pts',(76.846842092359,78.8119781131218,208.200592232552));
#28728=CARTESIAN_POINT('Ctrl Pts',(76.8377292359511,78.8141945740679,208.2));
#28729=CARTESIAN_POINT('Origin',(77.215862801455,80.368869783441,212.));
#28730=CARTESIAN_POINT('',(76.8377292359507,78.8141945740679,209.6));
#28731=CARTESIAN_POINT('',(76.8377292359515,78.8141945740678,209.512499998088));
#28732=CARTESIAN_POINT('',(76.8377292359511,78.8141945740678,212.));
#28733=CARTESIAN_POINT('Ctrl Pts',(76.8377292359514,78.8141945740678,208.812499998088));
#28734=CARTESIAN_POINT('Ctrl Pts',(76.9117861001804,78.7961822034118,208.817312856293));
#28735=CARTESIAN_POINT('Ctrl Pts',(76.9871810149374,78.7834478133498,208.822327552005));
#28736=CARTESIAN_POINT('Ctrl Pts',(77.2764642233986,78.7557509783693,208.842002361462));
#28737=CARTESIAN_POINT('Ctrl Pts',(77.4914599607559,78.7783229727028,208.857509485931));
#28738=CARTESIAN_POINT('Ctrl Pts',(77.891999254429,78.904212966651,208.888118238391));
#28739=CARTESIAN_POINT('Ctrl Pts',(78.0746841308784,79.0032786127344,208.902932649615));
#28740=CARTESIAN_POINT('Ctrl Pts',(78.3941473199926,79.2666270286464,208.930686210092));
#28741=CARTESIAN_POINT('Ctrl Pts',(78.5273265651122,79.4289909173781,208.943508557155));
#28742=CARTESIAN_POINT('Ctrl Pts',(78.7256759252887,79.7986468145787,208.973117163087));
#28743=CARTESIAN_POINT('Ctrl Pts',(78.7877209789437,80.0028889353391,208.988657139353));
#28744=CARTESIAN_POINT('Ctrl Pts',(78.8280647507798,80.4157520639106,209.018604169536));
#28745=CARTESIAN_POINT('Ctrl Pts',(78.8090546736185,80.6202277288121,209.032763898));
#28746=CARTESIAN_POINT('Ctrl Pts',(78.6929807637921,81.0193264871479,209.059040216555));
#28747=CARTESIAN_POINT('Ctrl Pts',(78.5938153353027,81.2093094331402,209.07380566194));
#28748=CARTESIAN_POINT('Ctrl Pts',(78.3290952503072,81.5369145567883,209.104262403781));
#28749=CARTESIAN_POINT('Ctrl Pts',(78.1672858277899,81.672104377895,209.119603373155));
#28750=CARTESIAN_POINT('Ctrl Pts',(77.8058893717694,81.8699115993271,209.148623816298));
#28751=CARTESIAN_POINT('Ctrl Pts',(77.6108449824573,81.9325932893769,209.161135508644));
#28752=CARTESIAN_POINT('Ctrl Pts',(77.1984050893787,81.982812432269,209.188966483185));
#28753=CARTESIAN_POINT('Ctrl Pts',(76.9845865057771,81.9662399063241,209.204268237249));
#28754=CARTESIAN_POINT('Ctrl Pts',(76.5816439968789,81.8522386682799,209.234801416215));
#28755=CARTESIAN_POINT('Ctrl Pts',(76.395709763203,81.7581123737807,209.249741936985));
#28756=CARTESIAN_POINT('Ctrl Pts',(76.0697589604614,81.504272494516,209.277754528787));
#28757=CARTESIAN_POINT('Ctrl Pts',(75.9329015039603,81.3469861040627,209.290308219051));
#28758=CARTESIAN_POINT('Ctrl Pts',(75.7238011499693,80.9842642711913,209.319610807118));
#28759=CARTESIAN_POINT('Ctrl Pts',(75.6554782008993,80.7813539375629,209.335164609594));
#28760=CARTESIAN_POINT('Ctrl Pts',(75.602906180264,80.3686585369461,209.365310481194));
#28761=CARTESIAN_POINT('Ctrl Pts',(75.6160673347275,80.1631311343417,209.379645518849));
#28762=CARTESIAN_POINT('Ctrl Pts',(75.721542016164,79.758184447611,209.406518822256));
#28763=CARTESIAN_POINT('Ctrl Pts',(75.8167054451588,79.5636534840546,209.420913789842));
#28764=CARTESIAN_POINT('Ctrl Pts',(76.0750556983137,79.2276515583953,209.451457345137));
#28765=CARTESIAN_POINT('Ctrl Pts',(76.2339935886625,79.0883386734642,209.466854456699));
#28766=CARTESIAN_POINT('Ctrl Pts',(76.5475346151698,78.9071303852898,209.492515136969));
#28767=CARTESIAN_POINT('Ctrl Pts',(76.6897902221338,78.8501768206713,209.502885636153));
#28768=CARTESIAN_POINT('Ctrl Pts',(76.8377292359518,78.8141945740677,209.512499998088));
#28769=CARTESIAN_POINT('Ctrl Pts',(76.8377292359504,78.814194574068,209.6));
#28770=CARTESIAN_POINT('Ctrl Pts',(76.7942908559166,78.8247598094451,209.597176996813));
#28771=CARTESIAN_POINT('Ctrl Pts',(76.7512492262698,78.8371566672181,209.594282698051));
#28772=CARTESIAN_POINT('Ctrl Pts',(76.5140714446782,78.9164207692148,209.577782441394));
#28773=CARTESIAN_POINT('Ctrl Pts',(76.3337928147036,79.0183018514361,209.563144436412));
#28774=CARTESIAN_POINT('Ctrl Pts',(76.0154770429867,79.2897375258994,209.532689024434));
#28775=CARTESIAN_POINT('Ctrl Pts',(75.8825033975968,79.4591278980739,209.517146947354));
#28776=CARTESIAN_POINT('Ctrl Pts',(75.6947207488768,79.8322719764637,209.488455217788));
#28777=CARTESIAN_POINT('Ctrl Pts',(75.6386764922219,80.0307940860058,209.476132128372));
#28778=CARTESIAN_POINT('Ctrl Pts',(75.604082006991,80.4414297232222,209.447634303082));
#28779=CARTESIAN_POINT('Ctrl Pts',(75.6270862834564,80.6497085558458,209.432481097433));
#28780=CARTESIAN_POINT('Ctrl Pts',(75.752735412568,81.0502703273327,209.401935594412));
#28781=CARTESIAN_POINT('Ctrl Pts',(75.855943501156,81.2381869490555,209.386842949294));
#28782=CARTESIAN_POINT('Ctrl Pts',(76.1235765041631,81.5554660965533,209.359751352111));
#28783=CARTESIAN_POINT('Ctrl Pts',(76.2825684687308,81.6842053783251,209.346674233288));
#28784=CARTESIAN_POINT('Ctrl Pts',(76.6466554791337,81.8788731444417,209.317206178883));
#28785=CARTESIAN_POINT('Ctrl Pts',(76.8495572389379,81.9404695091472,209.301745269278));
#28786=CARTESIAN_POINT('Ctrl Pts',(77.269654312385,81.981974038721,209.271497997527));
#28787=CARTESIAN_POINT('Ctrl Pts',(77.4827137482154,81.9606415523302,209.257737116563));
#28788=CARTESIAN_POINT('Ctrl Pts',(77.8811026128087,81.8383493555527,209.230567741071));
#28789=CARTESIAN_POINT('Ctrl Pts',(78.0634291017205,81.7412780091156,209.216063894433));
#28790=CARTESIAN_POINT('Ctrl Pts',(78.3877714364682,81.4787559021546,209.185739419629));
#28791=CARTESIAN_POINT('Ctrl Pts',(78.5247600209496,81.3133408784821,209.170185741196));
#28792=CARTESIAN_POINT('Ctrl Pts',(78.7225796795045,80.9450468700421,209.141208832876));
#28793=CARTESIAN_POINT('Ctrl Pts',(78.7840025383195,80.7471701291659,209.128826191886));
#28794=CARTESIAN_POINT('Ctrl Pts',(78.8288986903484,80.3371594828524,209.100550172892));
#28795=CARTESIAN_POINT('Ctrl Pts',(78.8112547470093,80.1288907067295,209.085490052499));
#28796=CARTESIAN_POINT('Ctrl Pts',(78.6961845719065,79.7256656223808,209.054938154282));
#28797=CARTESIAN_POINT('Ctrl Pts',(78.5978694193352,79.5351058904301,209.03974256019));
#28798=CARTESIAN_POINT('Ctrl Pts',(78.3384943630141,79.2109310072873,209.012304698965));
#28799=CARTESIAN_POINT('Ctrl Pts',(78.1828658951182,79.0781111608098,208.999536877318));
#28800=CARTESIAN_POINT('Ctrl Pts',(77.8243860671525,78.8743527481466,208.97027481335));
#28801=CARTESIAN_POINT('Ctrl Pts',(77.623707638452,78.8076080485544,208.954863932446));
#28802=CARTESIAN_POINT('Ctrl Pts',(77.2225449303185,78.7570603845167,208.925756197003));
#28803=CARTESIAN_POINT('Ctrl Pts',(77.0266459230265,78.7682455938331,208.912277447025));
#28804=CARTESIAN_POINT('Ctrl Pts',(76.837729235951,78.8141945740679,208.9));
#28805=CARTESIAN_POINT('Origin',(77.215862801455,80.368869783441,212.));
#28806=CARTESIAN_POINT('',(76.8377292359509,78.8141945740679,210.3));
#28807=CARTESIAN_POINT('',(76.8377292359512,78.8141945740678,210.212499998088));
#28808=CARTESIAN_POINT('',(76.8377292359511,78.8141945740678,212.));
#28809=CARTESIAN_POINT('Ctrl Pts',(76.8377292359518,78.8141945740677,209.512499998088));
#28810=CARTESIAN_POINT('Ctrl Pts',(76.8862442835823,78.802394573765,209.515652927225));
#28811=CARTESIAN_POINT('Ctrl Pts',(76.935360342617,78.7928534801644,209.518894223502));
#28812=CARTESIAN_POINT('Ctrl Pts',(77.1950863244861,78.754969094926,209.536291899824));
#28813=CARTESIAN_POINT('Ctrl Pts',(77.4092120307742,78.7664703996703,209.551511176548));
#28814=CARTESIAN_POINT('Ctrl Pts',(77.8151760340083,78.8709925406764,209.582061448137));
#28815=CARTESIAN_POINT('Ctrl Pts',(78.0036866632141,78.9609734855733,209.597097266181));
#28816=CARTESIAN_POINT('Ctrl Pts',(78.334910275856,79.2069716197041,209.625318055162));
#28817=CARTESIAN_POINT('Ctrl Pts',(78.4747632965217,79.3601837318022,209.637727689104));
#28818=CARTESIAN_POINT('Ctrl Pts',(78.6925102643476,79.7171867555457,209.666774097412));
#28819=CARTESIAN_POINT('Ctrl Pts',(78.7659160943085,79.9188765542249,209.682329015168));
#28820=CARTESIAN_POINT('Ctrl Pts',(78.8284385204956,80.3311727507581,209.712618074578));
#28821=CARTESIAN_POINT('Ctrl Pts',(78.8200605799987,80.5374314086927,209.727087349915));
#28822=CARTESIAN_POINT('Ctrl Pts',(78.7242133712058,80.9433456001172,209.75419510894));
#28823=CARTESIAN_POINT('Ctrl Pts',(78.6346787952959,81.1383909680076,209.768079714338));
#28824=CARTESIAN_POINT('Ctrl Pts',(78.3860960677452,81.479995141551,209.798390175903));
#28825=CARTESIAN_POINT('Ctrl Pts',(78.2304176921289,81.623750918391,209.813839069646));
#28826=CARTESIAN_POINT('Ctrl Pts',(77.8784595048441,81.8392798590798,209.843253993662));
#28827=CARTESIAN_POINT('Ctrl Pts',(77.6869965317385,81.9113133854704,209.856243064268));
#28828=CARTESIAN_POINT('Ctrl Pts',(77.2779212303413,81.9817072837881,209.883424985593));
#28829=CARTESIAN_POINT('Ctrl Pts',(77.0636031282149,81.9756895263487,209.898545303591));
#28830=CARTESIAN_POINT('Ctrl Pts',(76.6546284829339,81.8814970527803,209.929094470332));
#28831=CARTESIAN_POINT('Ctrl Pts',(76.4634374439547,81.7960710115093,209.944224467541));
#28832=CARTESIAN_POINT('Ctrl Pts',(76.1265830158737,81.5585617417386,209.972665238197));
#28833=CARTESIAN_POINT('Ctrl Pts',(75.9835180214879,81.4096499123308,209.984996163619));
#28834=CARTESIAN_POINT('Ctrl Pts',(75.7566267729065,81.0588304429404,210.013762040584));
#28835=CARTESIAN_POINT('Ctrl Pts',(75.677819786164,80.8585790697991,210.029308120574));
#28836=CARTESIAN_POINT('Ctrl Pts',(75.6046744280676,80.4469689261906,210.059731633652));
#28837=CARTESIAN_POINT('Ctrl Pts',(75.6079223383217,80.2400528448175,210.074335892166));
#28838=CARTESIAN_POINT('Ctrl Pts',(75.6935536740291,79.8331803748162,210.101687592826));
#28839=CARTESIAN_POINT('Ctrl Pts',(75.7772311264332,79.6375937389282,210.115108963578));
#28840=CARTESIAN_POINT('Ctrl Pts',(76.0155027725043,79.2902500026941,210.145164576635));
#28841=CARTESIAN_POINT('Ctrl Pts',(76.1676174268031,79.141896015853,210.160657028122));
#28842=CARTESIAN_POINT('Ctrl Pts',(76.4956184297709,78.9287615566256,210.188687829182));
#28843=CARTESIAN_POINT('Ctrl Pts',(76.6625281596926,78.8568075952612,210.201113910571));
#28844=CARTESIAN_POINT('Ctrl Pts',(76.8377292359513,78.8141945740678,210.212499998088));
#28845=CARTESIAN_POINT('Ctrl Pts',(76.8377292359507,78.814194574068,210.3));
#28846=CARTESIAN_POINT('Ctrl Pts',(76.7687480941578,78.8309724096837,210.295517006321));
#28847=CARTESIAN_POINT('Ctrl Pts',(76.7008236983214,78.8523550273851,210.290857899815));
#28848=CARTESIAN_POINT('Ctrl Pts',(76.4422757112119,78.9532092563482,210.272143473695));
#28849=CARTESIAN_POINT('Ctrl Pts',(76.2664718582602,79.0645855604091,210.257263400465));
#28850=CARTESIAN_POINT('Ctrl Pts',(75.9609319759317,79.3534488295603,210.22660435113));
#28851=CARTESIAN_POINT('Ctrl Pts',(75.8363263466194,79.5305113967565,210.211117333421));
#28852=CARTESIAN_POINT('Ctrl Pts',(75.6687566621022,79.9130536754183,210.183018492143));
#28853=CARTESIAN_POINT('Ctrl Pts',(75.6234275719121,80.1130022581412,210.17057036958));
#28854=CARTESIAN_POINT('Ctrl Pts',(75.609857319051,80.5247069416304,210.141634497977));
#28855=CARTESIAN_POINT('Ctrl Pts',(75.6438450221561,80.7325813993198,210.126320669189));
#28856=CARTESIAN_POINT('Ctrl Pts',(75.790905719824,81.1268328673936,210.095853279948));
#28857=CARTESIAN_POINT('Ctrl Pts',(75.9038756447547,81.3089509307157,210.081003246673));
#28858=CARTESIAN_POINT('Ctrl Pts',(76.1881755710675,81.6119071707128,210.054639227763));
#28859=CARTESIAN_POINT('Ctrl Pts',(76.3542612929968,81.7323315479678,210.040670851305));
#28860=CARTESIAN_POINT('Ctrl Pts',(76.7298647110601,81.9078268056968,210.010790002062));
#28861=CARTESIAN_POINT('Ctrl Pts',(76.9369831120127,81.9584662165145,209.995258667715));
#28862=CARTESIAN_POINT('Ctrl Pts',(77.3564813822758,81.9762860006598,209.965538873194));
#28863=CARTESIAN_POINT('Ctrl Pts',(77.5646496144558,81.9442707452982,209.952591351819));
#28864=CARTESIAN_POINT('Ctrl Pts',(77.9542715115944,81.8031223657582,209.92493496972));
#28865=CARTESIAN_POINT('Ctrl Pts',(78.1323448530387,81.6964065582324,209.910169851419));
#28866=CARTESIAN_POINT('Ctrl Pts',(78.4443042338802,81.4160685686061,209.879601464765));
#28867=CARTESIAN_POINT('Ctrl Pts',(78.5730919626864,81.2427419612856,209.864081976157));
#28868=CARTESIAN_POINT('Ctrl Pts',(78.7506546572598,80.864784412002,209.83568691703));
#28869=CARTESIAN_POINT('Ctrl Pts',(78.8012631036944,80.665567090636,209.823341973441));
#28870=CARTESIAN_POINT('Ctrl Pts',(78.8252751596618,80.2543567708347,209.794621067973));
#28871=CARTESIAN_POINT('Ctrl Pts',(78.7967470803763,80.0462100137167,209.77938203026));
#28872=CARTESIAN_POINT('Ctrl Pts',(78.6602850281205,79.6486789352933,209.748864919813));
#28873=CARTESIAN_POINT('Ctrl Pts',(78.5521231839478,79.4636145846229,209.733888994856));
#28874=CARTESIAN_POINT('Ctrl Pts',(78.2760699131448,79.1535040912048,209.707160201061));
#28875=CARTESIAN_POINT('Ctrl Pts',(78.1135476494756,79.0289500624745,209.693678439137));
#28876=CARTESIAN_POINT('Ctrl Pts',(77.7436748553578,78.8438260633372,209.664001186349));
#28877=CARTESIAN_POINT('Ctrl Pts',(77.5385938536597,78.787670353911,209.648499326236));
#28878=CARTESIAN_POINT('Ctrl Pts',(77.1634696062218,78.7611896362101,209.62170704795));
#28879=CARTESIAN_POINT('Ctrl Pts',(76.9979584166627,78.7752230699009,209.610413083717));
#28880=CARTESIAN_POINT('Ctrl Pts',(76.8377292359503,78.814194574068,209.6));
#28881=CARTESIAN_POINT('Origin',(77.215862801455,80.368869783441,212.));
#28882=CARTESIAN_POINT('',(76.8377292359511,78.8141945740678,211.));
#28883=CARTESIAN_POINT('',(76.8377292359511,78.8141945740679,210.912499998088));
#28884=CARTESIAN_POINT('',(76.8377292359511,78.8141945740678,212.));
#28885=CARTESIAN_POINT('',(75.7705853637063,79.6824492651474,211.6));
#28886=CARTESIAN_POINT('Ctrl Pts',(75.7705853637062,79.6824492651474,211.6));
#28887=CARTESIAN_POINT('Ctrl Pts',(75.7127116257352,79.8043040254562,211.590812272922));
#28888=CARTESIAN_POINT('Ctrl Pts',(75.6705039153542,79.9329159682097,211.582518428267));
#28889=CARTESIAN_POINT('Ctrl Pts',(75.6185721019073,80.2016904192254,211.564370389863));
#28890=CARTESIAN_POINT('Ctrl Pts',(75.6100956975266,80.3408694116708,211.554655478317));
#28891=CARTESIAN_POINT('Ctrl Pts',(75.6342384712736,80.6896390858489,211.529528724962));
#28892=CARTESIAN_POINT('Ctrl Pts',(75.6902046363061,80.8949879995436,211.514015086573));
#28893=CARTESIAN_POINT('Ctrl Pts',(75.8780514037409,81.2712273915844,211.484121020397));
#28894=CARTESIAN_POINT('Ctrl Pts',(76.0076743264714,81.4385618794624,211.470946087786));
#28895=CARTESIAN_POINT('Ctrl Pts',(76.3208716620126,81.7109516499105,211.443445618933));
#28896=CARTESIAN_POINT('Ctrl Pts',(76.5003440872578,81.8146183718967,211.428761669952));
#28897=CARTESIAN_POINT('Ctrl Pts',(76.8962010668449,81.9510687922483,211.398264057233));
#28898=CARTESIAN_POINT('Ctrl Pts',(77.1098653081239,81.9795617872084,211.382728714258));
#28899=CARTESIAN_POINT('Ctrl Pts',(77.5265895643817,81.9516354056831,211.354140902766));
#28900=CARTESIAN_POINT('Ctrl Pts',(77.7257830195731,81.8991254680589,211.34181973093));
#28901=CARTESIAN_POINT('Ctrl Pts',(78.0970222399127,81.7204382190393,211.313242835828));
#28902=CARTESIAN_POINT('Ctrl Pts',(78.2648981435312,81.5947100816425,211.298058295601));
#28903=CARTESIAN_POINT('Ctrl Pts',(78.5461709019992,81.2828296812592,211.267520255385));
#28904=CARTESIAN_POINT('Ctrl Pts',(78.6555763416884,81.0984676551874,211.252467410117));
#28905=CARTESIAN_POINT('Ctrl Pts',(78.792871469451,80.7067357179128,211.225502630768));
#28906=CARTESIAN_POINT('Ctrl Pts',(78.8229751441819,80.5043436329824,211.212293272722));
#28907=CARTESIAN_POINT('Ctrl Pts',(78.8056160690616,80.0916075495711,211.182751331048));
#28908=CARTESIAN_POINT('Ctrl Pts',(78.7554772361788,79.8853646939831,211.16727477628));
#28909=CARTESIAN_POINT('Ctrl Pts',(78.5778002403132,79.5029311632517,211.137117100773));
#28910=CARTESIAN_POINT('Ctrl Pts',(78.4515978885323,79.3307766817871,211.123521497342));
#28911=CARTESIAN_POINT('Ctrl Pts',(78.1444020505696,79.0498548169265,211.096266062422));
#28912=CARTESIAN_POINT('Ctrl Pts',(77.9680662780484,78.9419376196915,211.081714459557));
#28913=CARTESIAN_POINT('Ctrl Pts',(77.5768771091062,78.7956668446035,211.051342144373));
#28914=CARTESIAN_POINT('Ctrl Pts',(77.3646134045188,78.7616379285038,211.035791308777));
#28915=CARTESIAN_POINT('Ctrl Pts',(77.0457190880988,78.7743972129179,211.013738213079));
#28916=CARTESIAN_POINT('Ctrl Pts',(76.9405061401058,78.7891968144167,211.006679335826));
#28917=CARTESIAN_POINT('Ctrl Pts',(76.8377292359511,78.8141945740678,211.));
#28918=CARTESIAN_POINT('',(76.6545412773313,78.870564692161,211.6));
#28919=CARTESIAN_POINT('Origin',(77.215862801455,80.368869783441,211.6));
#28920=CARTESIAN_POINT('Ctrl Pts',(76.8377292359511,78.8141945740678,210.912499998088));
#28921=CARTESIAN_POINT('Ctrl Pts',(77.038449004072,78.7653748070007,210.925544511827));
#28922=CARTESIAN_POINT('Ctrl Pts',(77.2468954172806,78.7558454971608,210.939935217219));
#28923=CARTESIAN_POINT('Ctrl Pts',(77.6582733012602,78.8171103436994,210.969977480965));
#28924=CARTESIAN_POINT('Ctrl Pts',(77.8569914622933,78.888110439331,210.985338434372));
#28925=CARTESIAN_POINT('Ctrl Pts',(78.210731531279,79.0994384791586,211.014424022625));
#28926=CARTESIAN_POINT('Ctrl Pts',(78.3635562622254,79.2357322791863,211.02699377697));
#28927=CARTESIAN_POINT('Ctrl Pts',(78.6158715202084,79.565695767531,211.054720108117));
#28928=CARTESIAN_POINT('Ctrl Pts',(78.7099829658183,79.7583937882494,211.069994761277));
#28929=CARTESIAN_POINT('Ctrl Pts',(78.8160411588355,80.1636563271765,211.100535715031));
#28930=CARTESIAN_POINT('Ctrl Pts',(78.8291522320142,80.3718099484641,211.115509563216));
#28931=CARTESIAN_POINT('Ctrl Pts',(78.7755087713307,80.7812380709433,211.143593570462));
#28932=CARTESIAN_POINT('Ctrl Pts',(78.7094458670987,80.9785902039949,211.156090429798));
#28933=CARTESIAN_POINT('Ctrl Pts',(78.503038382884,81.3426317847808,211.18530617422));
#28934=CARTESIAN_POINT('Ctrl Pts',(78.3626937012489,81.5045615368933,211.200861380132));
#28935=CARTESIAN_POINT('Ctrl Pts',(78.0333708446082,81.7593284959067,211.231058072714));
#28936=CARTESIAN_POINT('Ctrl Pts',(77.8493872576715,81.8522394178766,211.245439843767));
#28937=CARTESIAN_POINT('Ctrl Pts',(77.4473115727342,81.9663943425186,211.272393964221));
#28938=CARTESIAN_POINT('Ctrl Pts',(77.2320777590094,81.9830148099074,211.286606083563));
#28939=CARTESIAN_POINT('Ctrl Pts',(76.8119112771593,81.9311502697992,211.317070609277));
#28940=CARTESIAN_POINT('Ctrl Pts',(76.6110183595505,81.8648865131105,211.332486638964));
#28941=CARTESIAN_POINT('Ctrl Pts',(76.2520089838787,81.6619802240671,211.361768288196));
#28942=CARTESIAN_POINT('Ctrl Pts',(76.0960651164363,81.5295470033163,211.374561840147));
#28943=CARTESIAN_POINT('Ctrl Pts',(75.8359058962999,81.2060211670675,211.401967228916));
#28944=CARTESIAN_POINT('Ctrl Pts',(75.7371248802881,81.0157058464226,211.417153534263));
#28945=CARTESIAN_POINT('Ctrl Pts',(75.6210516696081,80.6127206269661,211.447705722754));
#28946=CARTESIAN_POINT('Ctrl Pts',(75.6029013253923,80.4044450639927,211.462775050631));
#28947=CARTESIAN_POINT('Ctrl Pts',(75.6468224760359,79.9943725896507,211.491072252065));
#28948=CARTESIAN_POINT('Ctrl Pts',(75.7077324777136,79.7964358226992,211.503445817942));
#28949=CARTESIAN_POINT('Ctrl Pts',(75.8956950985807,79.4443531646425,211.531086608675));
#28950=CARTESIAN_POINT('Ctrl Pts',(76.0172905095577,79.2913820444512,211.545201868697));
#28951=CARTESIAN_POINT('Ctrl Pts',(76.3080221565354,79.0374102574885,211.573323127396));
#28952=CARTESIAN_POINT('Ctrl Pts',(76.4744428920774,78.9380363310756,211.587103998264));
#28953=CARTESIAN_POINT('Ctrl Pts',(76.6545412773326,78.8705646921605,211.6));
#28954=CARTESIAN_POINT('Origin',(77.2158628014545,80.368869783439,198.006249999044));
#28955=CARTESIAN_POINT('',(77.5939963669566,81.9235449928104,211.6));
#28956=CARTESIAN_POINT('',(77.5939963669582,81.9235449928142,211.962499998088));
#28957=CARTESIAN_POINT('',(77.5939963669579,81.9235449928101,198.006249999044));
#28958=CARTESIAN_POINT('Origin',(77.215862801455,80.368869783441,211.6));
#28959=CARTESIAN_POINT('',(76.8377292359511,78.8141945740679,211.7));
#28960=CARTESIAN_POINT('Origin',(77.2158628014592,80.3688697834461,211.641666666667));
#28961=CARTESIAN_POINT('',(76.8377292359511,78.8141945740678,212.312499998088));
#28962=CARTESIAN_POINT('',(76.8377292359511,78.8141945740678,212.006249999044));
#28963=CARTESIAN_POINT('Ctrl Pts',(77.5939963669588,81.9235449928141,211.962499998088));
#28964=CARTESIAN_POINT('Ctrl Pts',(76.6964042163248,82.1418605086474,212.020833331422));
#28965=CARTESIAN_POINT('Ctrl Pts',(76.0585413582559,81.4736806618775,212.079166664755));
#28966=CARTESIAN_POINT('Ctrl Pts',(75.420678500187,80.8055008151075,212.137499998088));
#28967=CARTESIAN_POINT('Ctrl Pts',(75.680407792752,79.9190054525043,212.195833331422));
#28968=CARTESIAN_POINT('Ctrl Pts',(75.9401370853171,79.0325100899011,212.254166664755));
#28969=CARTESIAN_POINT('Ctrl Pts',(76.8377292359511,78.8141945740678,212.312499998088));
#28970=CARTESIAN_POINT('Origin',(77.2158628014549,80.3688697834408,198.006249999044));
#28971=CARTESIAN_POINT('',(77.5044528940591,81.5553919638894,211.568749999044));
#28972=CARTESIAN_POINT('',(77.5044528940591,81.5553919638894,211.743749999044));
#28973=CARTESIAN_POINT('',(77.504452894059,81.555391963889,198.006249999044));
#28974=CARTESIAN_POINT('',(76.9272727088508,79.1823476029925,212.093749999044));
#28975=CARTESIAN_POINT('Ctrl Pts',(77.5044528940591,81.5553919638894,211.743749999044));
#28976=CARTESIAN_POINT('Ctrl Pts',(76.8194139937778,81.7220095315399,211.802083332377));
#28977=CARTESIAN_POINT('Ctrl Pts',(76.332599497335,81.2120572251409,211.860416665711));
#28978=CARTESIAN_POINT('Ctrl Pts',(75.8457850008923,80.7021049187419,211.918749999044));
#28979=CARTESIAN_POINT('Ctrl Pts',(76.0440094047309,80.0255350446925,211.977083332377));
#28980=CARTESIAN_POINT('Ctrl Pts',(76.2422338085695,79.348965170643,212.035416665711));
#28981=CARTESIAN_POINT('Ctrl Pts',(76.9272727088508,79.1823476029925,212.093749999044));
#28982=CARTESIAN_POINT('',(76.9272727088508,79.1823476029925,211.918749999044));
#28983=CARTESIAN_POINT('',(76.9272727088508,79.1823476029925,212.006249999044));
#28984=CARTESIAN_POINT('Ctrl Pts',(77.5044528940591,81.5553919638894,211.568749999044));
#28985=CARTESIAN_POINT('Ctrl Pts',(76.8194139937778,81.7220095315399,211.627083332377));
#28986=CARTESIAN_POINT('Ctrl Pts',(76.332599497335,81.2120572251409,211.685416665711));
#28987=CARTESIAN_POINT('Ctrl Pts',(75.8457850008923,80.7021049187419,211.743749999044));
#28988=CARTESIAN_POINT('Ctrl Pts',(76.0440094047309,80.0255350446925,211.802083332377));
#28989=CARTESIAN_POINT('Ctrl Pts',(76.2422338085695,79.348965170643,211.860416665711));
#28990=CARTESIAN_POINT('Ctrl Pts',(76.9272727088508,79.1823476029925,211.918749999044));
#28991=CARTESIAN_POINT('Origin',(77.2158628014549,80.3688697834408,198.006249999044));
#28992=CARTESIAN_POINT('',(77.5044528940591,81.5553919638894,210.868749999044));
#28993=CARTESIAN_POINT('',(77.5044528940591,81.5553919638894,211.043749999044));
#28994=CARTESIAN_POINT('',(77.504452894059,81.555391963889,198.006249999044));
#28995=CARTESIAN_POINT('Ctrl Pts',(77.5044528940591,81.5553919638894,211.043749999044));
#28996=CARTESIAN_POINT('Ctrl Pts',(76.8194139937778,81.7220095315399,211.102083332377));
#28997=CARTESIAN_POINT('Ctrl Pts',(76.332599497335,81.2120572251409,211.160416665711));
#28998=CARTESIAN_POINT('Ctrl Pts',(75.8457850008923,80.7021049187419,211.218749999044));
#28999=CARTESIAN_POINT('Ctrl Pts',(76.0440094047309,80.0255350446925,211.277083332377));
#29000=CARTESIAN_POINT('Ctrl Pts',(76.2422338085695,79.348965170643,211.335416665711));
#29001=CARTESIAN_POINT('Ctrl Pts',(76.9272727088508,79.1823476029925,211.393749999044));
#29002=CARTESIAN_POINT('Ctrl Pts',(77.6123116091322,79.0157300353421,211.452083332377));
#29003=CARTESIAN_POINT('Ctrl Pts',(78.0991261055749,79.525682341741,211.510416665711));
#29004=CARTESIAN_POINT('Ctrl Pts',(78.5859406020177,80.03563464814,211.568749999044));
#29005=CARTESIAN_POINT('Ctrl Pts',(78.3877161981791,80.7122045221895,211.627083332377));
#29006=CARTESIAN_POINT('Ctrl Pts',(78.1894917943405,81.3887743962389,211.685416665711));
#29007=CARTESIAN_POINT('Ctrl Pts',(77.5044528940591,81.5553919638894,211.743749999044));
#29008=CARTESIAN_POINT('Ctrl Pts',(77.5044528940591,81.5553919638894,210.868749999044));
#29009=CARTESIAN_POINT('Ctrl Pts',(76.8194139937778,81.7220095315399,210.927083332377));
#29010=CARTESIAN_POINT('Ctrl Pts',(76.332599497335,81.2120572251409,210.985416665711));
#29011=CARTESIAN_POINT('Ctrl Pts',(75.8457850008923,80.7021049187419,211.043749999044));
#29012=CARTESIAN_POINT('Ctrl Pts',(76.0440094047309,80.0255350446925,211.102083332377));
#29013=CARTESIAN_POINT('Ctrl Pts',(76.2422338085695,79.348965170643,211.160416665711));
#29014=CARTESIAN_POINT('Ctrl Pts',(76.9272727088508,79.1823476029925,211.218749999044));
#29015=CARTESIAN_POINT('Ctrl Pts',(77.6123116091322,79.0157300353421,211.277083332377));
#29016=CARTESIAN_POINT('Ctrl Pts',(78.0991261055749,79.5256823417411,211.335416665711));
#29017=CARTESIAN_POINT('Ctrl Pts',(78.5859406020177,80.03563464814,211.393749999044));
#29018=CARTESIAN_POINT('Ctrl Pts',(78.3877161981791,80.7122045221895,211.452083332377));
#29019=CARTESIAN_POINT('Ctrl Pts',(78.1894917943405,81.3887743962389,211.510416665711));
#29020=CARTESIAN_POINT('Ctrl Pts',(77.5044528940591,81.5553919638894,211.568749999044));
#29021=CARTESIAN_POINT('Origin',(77.2158628014549,80.3688697834408,198.006249999044));
#29022=CARTESIAN_POINT('',(77.5044528940591,81.5553919638894,210.168749999044));
#29023=CARTESIAN_POINT('',(77.5044528940591,81.5553919638894,210.343749999044));
#29024=CARTESIAN_POINT('',(77.504452894059,81.555391963889,198.006249999044));
#29025=CARTESIAN_POINT('Ctrl Pts',(77.5044528940591,81.5553919638894,210.343749999044));
#29026=CARTESIAN_POINT('Ctrl Pts',(76.8194139937778,81.7220095315399,210.402083332377));
#29027=CARTESIAN_POINT('Ctrl Pts',(76.332599497335,81.2120572251409,210.460416665711));
#29028=CARTESIAN_POINT('Ctrl Pts',(75.8457850008923,80.7021049187419,210.518749999044));
#29029=CARTESIAN_POINT('Ctrl Pts',(76.0440094047309,80.0255350446925,210.577083332377));
#29030=CARTESIAN_POINT('Ctrl Pts',(76.2422338085695,79.348965170643,210.635416665711));
#29031=CARTESIAN_POINT('Ctrl Pts',(76.9272727088508,79.1823476029926,210.693749999044));
#29032=CARTESIAN_POINT('Ctrl Pts',(77.6123116091322,79.0157300353421,210.752083332377));
#29033=CARTESIAN_POINT('Ctrl Pts',(78.0991261055749,79.5256823417411,210.810416665711));
#29034=CARTESIAN_POINT('Ctrl Pts',(78.5859406020177,80.03563464814,210.868749999044));
#29035=CARTESIAN_POINT('Ctrl Pts',(78.3877161981791,80.7122045221895,210.927083332377));
#29036=CARTESIAN_POINT('Ctrl Pts',(78.1894917943405,81.3887743962389,210.985416665711));
#29037=CARTESIAN_POINT('Ctrl Pts',(77.5044528940591,81.5553919638894,211.043749999044));
#29038=CARTESIAN_POINT('Ctrl Pts',(77.5044528940591,81.5553919638894,210.168749999044));
#29039=CARTESIAN_POINT('Ctrl Pts',(76.8194139937778,81.7220095315399,210.227083332377));
#29040=CARTESIAN_POINT('Ctrl Pts',(76.332599497335,81.2120572251409,210.285416665711));
#29041=CARTESIAN_POINT('Ctrl Pts',(75.8457850008923,80.7021049187419,210.343749999044));
#29042=CARTESIAN_POINT('Ctrl Pts',(76.0440094047309,80.0255350446925,210.402083332377));
#29043=CARTESIAN_POINT('Ctrl Pts',(76.2422338085695,79.348965170643,210.460416665711));
#29044=CARTESIAN_POINT('Ctrl Pts',(76.9272727088508,79.1823476029926,210.518749999044));
#29045=CARTESIAN_POINT('Ctrl Pts',(77.6123116091322,79.0157300353421,210.577083332377));
#29046=CARTESIAN_POINT('Ctrl Pts',(78.0991261055749,79.5256823417411,210.635416665711));
#29047=CARTESIAN_POINT('Ctrl Pts',(78.5859406020177,80.03563464814,210.693749999044));
#29048=CARTESIAN_POINT('Ctrl Pts',(78.3877161981791,80.7122045221895,210.752083332377));
#29049=CARTESIAN_POINT('Ctrl Pts',(78.1894917943405,81.3887743962389,210.810416665711));
#29050=CARTESIAN_POINT('Ctrl Pts',(77.5044528940591,81.5553919638894,210.868749999044));
#29051=CARTESIAN_POINT('Origin',(77.2158628014549,80.3688697834408,198.006249999044));
#29052=CARTESIAN_POINT('',(77.5044528940591,81.5553919638894,209.468749999044));
#29053=CARTESIAN_POINT('',(77.5044528940591,81.5553919638894,209.643749999044));
#29054=CARTESIAN_POINT('',(77.504452894059,81.555391963889,198.006249999044));
#29055=CARTESIAN_POINT('Ctrl Pts',(77.5044528940591,81.5553919638894,209.643749999044));
#29056=CARTESIAN_POINT('Ctrl Pts',(76.8194139937778,81.7220095315399,209.702083332377));
#29057=CARTESIAN_POINT('Ctrl Pts',(76.332599497335,81.2120572251409,209.760416665711));
#29058=CARTESIAN_POINT('Ctrl Pts',(75.8457850008923,80.7021049187419,209.818749999044));
#29059=CARTESIAN_POINT('Ctrl Pts',(76.0440094047309,80.0255350446925,209.877083332377));
#29060=CARTESIAN_POINT('Ctrl Pts',(76.2422338085695,79.348965170643,209.935416665711));
#29061=CARTESIAN_POINT('Ctrl Pts',(76.9272727088508,79.1823476029926,209.993749999044));
#29062=CARTESIAN_POINT('Ctrl Pts',(77.6123116091322,79.0157300353421,210.052083332377));
#29063=CARTESIAN_POINT('Ctrl Pts',(78.0991261055749,79.5256823417411,210.110416665711));
#29064=CARTESIAN_POINT('Ctrl Pts',(78.5859406020177,80.03563464814,210.168749999044));
#29065=CARTESIAN_POINT('Ctrl Pts',(78.3877161981791,80.7122045221895,210.227083332377));
#29066=CARTESIAN_POINT('Ctrl Pts',(78.1894917943405,81.3887743962389,210.285416665711));
#29067=CARTESIAN_POINT('Ctrl Pts',(77.5044528940591,81.5553919638894,210.343749999044));
#29068=CARTESIAN_POINT('Ctrl Pts',(77.5044528940591,81.5553919638894,209.468749999044));
#29069=CARTESIAN_POINT('Ctrl Pts',(76.8194139937778,81.7220095315399,209.527083332377));
#29070=CARTESIAN_POINT('Ctrl Pts',(76.332599497335,81.2120572251409,209.585416665711));
#29071=CARTESIAN_POINT('Ctrl Pts',(75.8457850008923,80.7021049187419,209.643749999044));
#29072=CARTESIAN_POINT('Ctrl Pts',(76.0440094047309,80.0255350446925,209.702083332377));
#29073=CARTESIAN_POINT('Ctrl Pts',(76.2422338085695,79.348965170643,209.760416665711));
#29074=CARTESIAN_POINT('Ctrl Pts',(76.9272727088508,79.1823476029926,209.818749999044));
#29075=CARTESIAN_POINT('Ctrl Pts',(77.6123116091322,79.0157300353421,209.877083332377));
#29076=CARTESIAN_POINT('Ctrl Pts',(78.0991261055749,79.5256823417411,209.935416665711));
#29077=CARTESIAN_POINT('Ctrl Pts',(78.5859406020177,80.03563464814,209.993749999044));
#29078=CARTESIAN_POINT('Ctrl Pts',(78.3877161981791,80.7122045221895,210.052083332377));
#29079=CARTESIAN_POINT('Ctrl Pts',(78.1894917943405,81.3887743962389,210.110416665711));
#29080=CARTESIAN_POINT('Ctrl Pts',(77.5044528940591,81.5553919638894,210.168749999044));
#29081=CARTESIAN_POINT('Origin',(77.2158628014549,80.3688697834408,198.006249999044));
#29082=CARTESIAN_POINT('',(77.5044528940591,81.5553919638894,208.768749999044));
#29083=CARTESIAN_POINT('',(77.5044528940591,81.5553919638894,208.943749999044));
#29084=CARTESIAN_POINT('',(77.504452894059,81.555391963889,198.006249999044));
#29085=CARTESIAN_POINT('Ctrl Pts',(77.5044528940591,81.5553919638894,208.943749999044));
#29086=CARTESIAN_POINT('Ctrl Pts',(76.8194139937778,81.7220095315399,209.002083332377));
#29087=CARTESIAN_POINT('Ctrl Pts',(76.332599497335,81.2120572251409,209.060416665711));
#29088=CARTESIAN_POINT('Ctrl Pts',(75.8457850008923,80.7021049187419,209.118749999044));
#29089=CARTESIAN_POINT('Ctrl Pts',(76.0440094047309,80.0255350446925,209.177083332377));
#29090=CARTESIAN_POINT('Ctrl Pts',(76.2422338085695,79.348965170643,209.235416665711));
#29091=CARTESIAN_POINT('Ctrl Pts',(76.9272727088508,79.1823476029926,209.293749999044));
#29092=CARTESIAN_POINT('Ctrl Pts',(77.6123116091322,79.0157300353421,209.352083332377));
#29093=CARTESIAN_POINT('Ctrl Pts',(78.0991261055749,79.5256823417411,209.410416665711));
#29094=CARTESIAN_POINT('Ctrl Pts',(78.5859406020177,80.03563464814,209.468749999044));
#29095=CARTESIAN_POINT('Ctrl Pts',(78.3877161981791,80.7122045221895,209.527083332377));
#29096=CARTESIAN_POINT('Ctrl Pts',(78.1894917943405,81.3887743962389,209.585416665711));
#29097=CARTESIAN_POINT('Ctrl Pts',(77.5044528940591,81.5553919638894,209.643749999044));
#29098=CARTESIAN_POINT('Ctrl Pts',(77.5044528940591,81.5553919638894,208.768749999044));
#29099=CARTESIAN_POINT('Ctrl Pts',(76.8194139937778,81.7220095315399,208.827083332377));
#29100=CARTESIAN_POINT('Ctrl Pts',(76.332599497335,81.2120572251409,208.885416665711));
#29101=CARTESIAN_POINT('Ctrl Pts',(75.8457850008923,80.7021049187419,208.943749999044));
#29102=CARTESIAN_POINT('Ctrl Pts',(76.0440094047309,80.0255350446925,209.002083332377));
#29103=CARTESIAN_POINT('Ctrl Pts',(76.2422338085695,79.348965170643,209.060416665711));
#29104=CARTESIAN_POINT('Ctrl Pts',(76.9272727088508,79.1823476029926,209.118749999044));
#29105=CARTESIAN_POINT('Ctrl Pts',(77.6123116091322,79.0157300353421,209.177083332377));
#29106=CARTESIAN_POINT('Ctrl Pts',(78.0991261055749,79.5256823417411,209.235416665711));
#29107=CARTESIAN_POINT('Ctrl Pts',(78.5859406020177,80.03563464814,209.293749999044));
#29108=CARTESIAN_POINT('Ctrl Pts',(78.3877161981791,80.7122045221895,209.352083332377));
#29109=CARTESIAN_POINT('Ctrl Pts',(78.1894917943405,81.3887743962389,209.410416665711));
#29110=CARTESIAN_POINT('Ctrl Pts',(77.5044528940591,81.5553919638894,209.468749999044));
#29111=CARTESIAN_POINT('Origin',(77.2158628014549,80.3688697834408,198.006249999044));
#29112=CARTESIAN_POINT('',(77.5044528940591,81.5553919638894,208.068749999044));
#29113=CARTESIAN_POINT('',(77.5044528940591,81.5553919638894,208.243749999044));
#29114=CARTESIAN_POINT('',(77.504452894059,81.555391963889,198.006249999044));
#29115=CARTESIAN_POINT('Ctrl Pts',(77.5044528940591,81.5553919638894,208.243749999044));
#29116=CARTESIAN_POINT('Ctrl Pts',(76.8194139937778,81.7220095315399,208.302083332377));
#29117=CARTESIAN_POINT('Ctrl Pts',(76.332599497335,81.2120572251409,208.360416665711));
#29118=CARTESIAN_POINT('Ctrl Pts',(75.8457850008923,80.7021049187419,208.418749999044));
#29119=CARTESIAN_POINT('Ctrl Pts',(76.0440094047309,80.0255350446925,208.477083332377));
#29120=CARTESIAN_POINT('Ctrl Pts',(76.2422338085695,79.348965170643,208.535416665711));
#29121=CARTESIAN_POINT('Ctrl Pts',(76.9272727088508,79.1823476029926,208.593749999044));
#29122=CARTESIAN_POINT('Ctrl Pts',(77.6123116091322,79.0157300353421,208.652083332377));
#29123=CARTESIAN_POINT('Ctrl Pts',(78.0991261055749,79.5256823417411,208.710416665711));
#29124=CARTESIAN_POINT('Ctrl Pts',(78.5859406020177,80.03563464814,208.768749999044));
#29125=CARTESIAN_POINT('Ctrl Pts',(78.3877161981791,80.7122045221895,208.827083332377));
#29126=CARTESIAN_POINT('Ctrl Pts',(78.1894917943405,81.3887743962389,208.885416665711));
#29127=CARTESIAN_POINT('Ctrl Pts',(77.5044528940591,81.5553919638894,208.943749999044));
#29128=CARTESIAN_POINT('Ctrl Pts',(77.5044528940591,81.5553919638894,208.068749999044));
#29129=CARTESIAN_POINT('Ctrl Pts',(76.8194139937778,81.7220095315399,208.127083332377));
#29130=CARTESIAN_POINT('Ctrl Pts',(76.332599497335,81.2120572251409,208.185416665711));
#29131=CARTESIAN_POINT('Ctrl Pts',(75.8457850008923,80.7021049187419,208.243749999044));
#29132=CARTESIAN_POINT('Ctrl Pts',(76.0440094047309,80.0255350446925,208.302083332377));
#29133=CARTESIAN_POINT('Ctrl Pts',(76.2422338085695,79.348965170643,208.360416665711));
#29134=CARTESIAN_POINT('Ctrl Pts',(76.9272727088508,79.1823476029926,208.418749999044));
#29135=CARTESIAN_POINT('Ctrl Pts',(77.6123116091322,79.0157300353421,208.477083332377));
#29136=CARTESIAN_POINT('Ctrl Pts',(78.0991261055749,79.5256823417411,208.535416665711));
#29137=CARTESIAN_POINT('Ctrl Pts',(78.5859406020177,80.03563464814,208.593749999044));
#29138=CARTESIAN_POINT('Ctrl Pts',(78.3877161981791,80.7122045221895,208.652083332377));
#29139=CARTESIAN_POINT('Ctrl Pts',(78.1894917943405,81.3887743962389,208.710416665711));
#29140=CARTESIAN_POINT('Ctrl Pts',(77.5044528940591,81.5553919638894,208.768749999044));
#29141=CARTESIAN_POINT('Origin',(77.2158628014549,80.3688697834408,198.006249999044));
#29142=CARTESIAN_POINT('',(77.5044528940591,81.5553919638894,207.368749999044));
#29143=CARTESIAN_POINT('',(77.5044528940591,81.5553919638894,207.543749999044));
#29144=CARTESIAN_POINT('',(77.504452894059,81.555391963889,198.006249999044));
#29145=CARTESIAN_POINT('Ctrl Pts',(77.5044528940591,81.5553919638894,207.543749999044));
#29146=CARTESIAN_POINT('Ctrl Pts',(76.8194139937778,81.7220095315399,207.602083332377));
#29147=CARTESIAN_POINT('Ctrl Pts',(76.332599497335,81.2120572251409,207.660416665711));
#29148=CARTESIAN_POINT('Ctrl Pts',(75.8457850008923,80.7021049187419,207.718749999044));
#29149=CARTESIAN_POINT('Ctrl Pts',(76.0440094047309,80.0255350446925,207.777083332377));
#29150=CARTESIAN_POINT('Ctrl Pts',(76.2422338085695,79.348965170643,207.835416665711));
#29151=CARTESIAN_POINT('Ctrl Pts',(76.9272727088508,79.1823476029926,207.893749999044));
#29152=CARTESIAN_POINT('Ctrl Pts',(77.6123116091322,79.0157300353421,207.952083332377));
#29153=CARTESIAN_POINT('Ctrl Pts',(78.0991261055749,79.5256823417411,208.010416665711));
#29154=CARTESIAN_POINT('Ctrl Pts',(78.5859406020177,80.03563464814,208.068749999044));
#29155=CARTESIAN_POINT('Ctrl Pts',(78.3877161981791,80.7122045221895,208.127083332377));
#29156=CARTESIAN_POINT('Ctrl Pts',(78.1894917943405,81.3887743962389,208.185416665711));
#29157=CARTESIAN_POINT('Ctrl Pts',(77.5044528940591,81.5553919638894,208.243749999044));
#29158=CARTESIAN_POINT('Ctrl Pts',(77.5044528940591,81.5553919638894,207.368749999044));
#29159=CARTESIAN_POINT('Ctrl Pts',(76.8194139937778,81.7220095315399,207.427083332377));
#29160=CARTESIAN_POINT('Ctrl Pts',(76.332599497335,81.2120572251409,207.485416665711));
#29161=CARTESIAN_POINT('Ctrl Pts',(75.8457850008923,80.7021049187419,207.543749999044));
#29162=CARTESIAN_POINT('Ctrl Pts',(76.0440094047309,80.0255350446925,207.602083332377));
#29163=CARTESIAN_POINT('Ctrl Pts',(76.2422338085695,79.348965170643,207.660416665711));
#29164=CARTESIAN_POINT('Ctrl Pts',(76.9272727088508,79.1823476029926,207.718749999044));
#29165=CARTESIAN_POINT('Ctrl Pts',(77.6123116091322,79.0157300353421,207.777083332377));
#29166=CARTESIAN_POINT('Ctrl Pts',(78.0991261055749,79.5256823417411,207.835416665711));
#29167=CARTESIAN_POINT('Ctrl Pts',(78.5859406020177,80.03563464814,207.893749999044));
#29168=CARTESIAN_POINT('Ctrl Pts',(78.3877161981791,80.7122045221895,207.952083332377));
#29169=CARTESIAN_POINT('Ctrl Pts',(78.1894917943405,81.3887743962389,208.010416665711));
#29170=CARTESIAN_POINT('Ctrl Pts',(77.5044528940591,81.5553919638894,208.068749999044));
#29171=CARTESIAN_POINT('Origin',(77.2158628014549,80.3688697834408,198.006249999044));
#29172=CARTESIAN_POINT('',(77.5044528940591,81.5553919638894,206.668749999044));
#29173=CARTESIAN_POINT('',(77.5044528940591,81.5553919638894,206.843749999044));
#29174=CARTESIAN_POINT('',(77.504452894059,81.555391963889,198.006249999044));
#29175=CARTESIAN_POINT('Ctrl Pts',(77.5044528940591,81.5553919638894,206.843749999044));
#29176=CARTESIAN_POINT('Ctrl Pts',(76.8194139937778,81.7220095315399,206.902083332377));
#29177=CARTESIAN_POINT('Ctrl Pts',(76.332599497335,81.2120572251409,206.960416665711));
#29178=CARTESIAN_POINT('Ctrl Pts',(75.8457850008923,80.7021049187419,207.018749999044));
#29179=CARTESIAN_POINT('Ctrl Pts',(76.0440094047309,80.0255350446925,207.077083332377));
#29180=CARTESIAN_POINT('Ctrl Pts',(76.2422338085695,79.348965170643,207.135416665711));
#29181=CARTESIAN_POINT('Ctrl Pts',(76.9272727088508,79.1823476029926,207.193749999044));
#29182=CARTESIAN_POINT('Ctrl Pts',(77.6123116091322,79.0157300353421,207.252083332377));
#29183=CARTESIAN_POINT('Ctrl Pts',(78.099126105575,79.5256823417411,207.310416665711));
#29184=CARTESIAN_POINT('Ctrl Pts',(78.5859406020177,80.03563464814,207.368749999044));
#29185=CARTESIAN_POINT('Ctrl Pts',(78.3877161981791,80.7122045221895,207.427083332377));
#29186=CARTESIAN_POINT('Ctrl Pts',(78.1894917943405,81.3887743962389,207.485416665711));
#29187=CARTESIAN_POINT('Ctrl Pts',(77.5044528940591,81.5553919638894,207.543749999044));
#29188=CARTESIAN_POINT('Ctrl Pts',(77.5044528940591,81.5553919638894,206.668749999044));
#29189=CARTESIAN_POINT('Ctrl Pts',(76.8194139937778,81.7220095315399,206.727083332378));
#29190=CARTESIAN_POINT('Ctrl Pts',(76.332599497335,81.2120572251409,206.785416665711));
#29191=CARTESIAN_POINT('Ctrl Pts',(75.8457850008923,80.7021049187419,206.843749999044));
#29192=CARTESIAN_POINT('Ctrl Pts',(76.0440094047309,80.0255350446925,206.902083332377));
#29193=CARTESIAN_POINT('Ctrl Pts',(76.2422338085695,79.348965170643,206.960416665711));
#29194=CARTESIAN_POINT('Ctrl Pts',(76.9272727088508,79.1823476029926,207.018749999044));
#29195=CARTESIAN_POINT('Ctrl Pts',(77.6123116091322,79.0157300353421,207.077083332377));
#29196=CARTESIAN_POINT('Ctrl Pts',(78.099126105575,79.5256823417411,207.135416665711));
#29197=CARTESIAN_POINT('Ctrl Pts',(78.5859406020177,80.03563464814,207.193749999044));
#29198=CARTESIAN_POINT('Ctrl Pts',(78.3877161981791,80.7122045221895,207.252083332377));
#29199=CARTESIAN_POINT('Ctrl Pts',(78.1894917943405,81.3887743962389,207.310416665711));
#29200=CARTESIAN_POINT('Ctrl Pts',(77.5044528940591,81.5553919638894,207.368749999044));
#29201=CARTESIAN_POINT('Origin',(77.2158628014549,80.3688697834408,198.006249999044));
#29202=CARTESIAN_POINT('',(77.5044528940591,81.5553919638894,205.968749999044));
#29203=CARTESIAN_POINT('',(77.5044528940591,81.5553919638894,206.143749999044));
#29204=CARTESIAN_POINT('',(77.504452894059,81.555391963889,198.006249999044));
#29205=CARTESIAN_POINT('Ctrl Pts',(77.5044528940591,81.5553919638894,206.143749999044));
#29206=CARTESIAN_POINT('Ctrl Pts',(76.8194139937778,81.7220095315399,206.202083332377));
#29207=CARTESIAN_POINT('Ctrl Pts',(76.332599497335,81.2120572251409,206.260416665711));
#29208=CARTESIAN_POINT('Ctrl Pts',(75.8457850008923,80.7021049187419,206.318749999044));
#29209=CARTESIAN_POINT('Ctrl Pts',(76.0440094047309,80.0255350446925,206.377083332377));
#29210=CARTESIAN_POINT('Ctrl Pts',(76.2422338085695,79.348965170643,206.435416665711));
#29211=CARTESIAN_POINT('Ctrl Pts',(76.9272727088508,79.1823476029926,206.493749999044));
#29212=CARTESIAN_POINT('Ctrl Pts',(77.6123116091322,79.0157300353421,206.552083332377));
#29213=CARTESIAN_POINT('Ctrl Pts',(78.099126105575,79.5256823417411,206.610416665711));
#29214=CARTESIAN_POINT('Ctrl Pts',(78.5859406020177,80.03563464814,206.668749999044));
#29215=CARTESIAN_POINT('Ctrl Pts',(78.3877161981791,80.7122045221895,206.727083332377));
#29216=CARTESIAN_POINT('Ctrl Pts',(78.1894917943405,81.3887743962389,206.785416665711));
#29217=CARTESIAN_POINT('Ctrl Pts',(77.5044528940591,81.5553919638894,206.843749999044));
#29218=CARTESIAN_POINT('Ctrl Pts',(77.5044528940591,81.5553919638894,205.968749999044));
#29219=CARTESIAN_POINT('Ctrl Pts',(76.8194139937778,81.7220095315399,206.027083332377));
#29220=CARTESIAN_POINT('Ctrl Pts',(76.332599497335,81.2120572251409,206.085416665711));
#29221=CARTESIAN_POINT('Ctrl Pts',(75.8457850008923,80.7021049187419,206.143749999044));
#29222=CARTESIAN_POINT('Ctrl Pts',(76.0440094047309,80.0255350446925,206.202083332377));
#29223=CARTESIAN_POINT('Ctrl Pts',(76.2422338085695,79.348965170643,206.260416665711));
#29224=CARTESIAN_POINT('Ctrl Pts',(76.9272727088508,79.1823476029926,206.318749999044));
#29225=CARTESIAN_POINT('Ctrl Pts',(77.6123116091322,79.0157300353421,206.377083332377));
#29226=CARTESIAN_POINT('Ctrl Pts',(78.099126105575,79.5256823417411,206.435416665711));
#29227=CARTESIAN_POINT('Ctrl Pts',(78.5859406020177,80.03563464814,206.493749999044));
#29228=CARTESIAN_POINT('Ctrl Pts',(78.3877161981791,80.7122045221895,206.552083332377));
#29229=CARTESIAN_POINT('Ctrl Pts',(78.1894917943405,81.3887743962389,206.610416665711));
#29230=CARTESIAN_POINT('Ctrl Pts',(77.5044528940591,81.5553919638894,206.668749999044));
#29231=CARTESIAN_POINT('Origin',(77.2158628014549,80.3688697834408,198.006249999044));
#29232=CARTESIAN_POINT('',(77.5044528940591,81.5553919638894,205.268749999044));
#29233=CARTESIAN_POINT('',(77.5044528940591,81.5553919638894,205.443749999044));
#29234=CARTESIAN_POINT('',(77.504452894059,81.555391963889,198.006249999044));
#29235=CARTESIAN_POINT('Ctrl Pts',(77.5044528940591,81.5553919638894,205.443749999044));
#29236=CARTESIAN_POINT('Ctrl Pts',(76.8194139937778,81.7220095315399,205.502083332377));
#29237=CARTESIAN_POINT('Ctrl Pts',(76.332599497335,81.2120572251409,205.560416665711));
#29238=CARTESIAN_POINT('Ctrl Pts',(75.8457850008923,80.7021049187419,205.618749999044));
#29239=CARTESIAN_POINT('Ctrl Pts',(76.0440094047309,80.0255350446925,205.677083332377));
#29240=CARTESIAN_POINT('Ctrl Pts',(76.2422338085695,79.348965170643,205.735416665711));
#29241=CARTESIAN_POINT('Ctrl Pts',(76.9272727088508,79.1823476029926,205.793749999044));
#29242=CARTESIAN_POINT('Ctrl Pts',(77.6123116091322,79.0157300353421,205.852083332377));
#29243=CARTESIAN_POINT('Ctrl Pts',(78.099126105575,79.5256823417411,205.910416665711));
#29244=CARTESIAN_POINT('Ctrl Pts',(78.5859406020177,80.03563464814,205.968749999044));
#29245=CARTESIAN_POINT('Ctrl Pts',(78.3877161981791,80.7122045221895,206.027083332377));
#29246=CARTESIAN_POINT('Ctrl Pts',(78.1894917943405,81.3887743962389,206.085416665711));
#29247=CARTESIAN_POINT('Ctrl Pts',(77.5044528940591,81.5553919638894,206.143749999044));
#29248=CARTESIAN_POINT('Ctrl Pts',(77.5044528940591,81.5553919638894,205.268749999044));
#29249=CARTESIAN_POINT('Ctrl Pts',(76.8194139937778,81.7220095315399,205.327083332377));
#29250=CARTESIAN_POINT('Ctrl Pts',(76.332599497335,81.2120572251409,205.385416665711));
#29251=CARTESIAN_POINT('Ctrl Pts',(75.8457850008923,80.7021049187419,205.443749999044));
#29252=CARTESIAN_POINT('Ctrl Pts',(76.0440094047309,80.0255350446925,205.502083332377));
#29253=CARTESIAN_POINT('Ctrl Pts',(76.2422338085695,79.348965170643,205.560416665711));
#29254=CARTESIAN_POINT('Ctrl Pts',(76.9272727088508,79.1823476029926,205.618749999044));
#29255=CARTESIAN_POINT('Ctrl Pts',(77.6123116091322,79.0157300353421,205.677083332377));
#29256=CARTESIAN_POINT('Ctrl Pts',(78.099126105575,79.5256823417411,205.735416665711));
#29257=CARTESIAN_POINT('Ctrl Pts',(78.5859406020177,80.03563464814,205.793749999044));
#29258=CARTESIAN_POINT('Ctrl Pts',(78.3877161981791,80.7122045221895,205.852083332377));
#29259=CARTESIAN_POINT('Ctrl Pts',(78.1894917943405,81.388774396239,205.910416665711));
#29260=CARTESIAN_POINT('Ctrl Pts',(77.5044528940591,81.5553919638894,205.968749999044));
#29261=CARTESIAN_POINT('Origin',(77.2158628014549,80.3688697834408,198.006249999044));
#29262=CARTESIAN_POINT('',(77.5044528940591,81.5553919638894,204.568749999044));
#29263=CARTESIAN_POINT('',(77.5044528940591,81.5553919638894,204.743749999044));
#29264=CARTESIAN_POINT('',(77.504452894059,81.555391963889,198.006249999044));
#29265=CARTESIAN_POINT('Ctrl Pts',(77.5044528940591,81.5553919638894,204.743749999044));
#29266=CARTESIAN_POINT('Ctrl Pts',(76.8194139937778,81.7220095315399,204.802083332378));
#29267=CARTESIAN_POINT('Ctrl Pts',(76.332599497335,81.2120572251409,204.860416665711));
#29268=CARTESIAN_POINT('Ctrl Pts',(75.8457850008923,80.7021049187419,204.918749999044));
#29269=CARTESIAN_POINT('Ctrl Pts',(76.0440094047309,80.0255350446925,204.977083332377));
#29270=CARTESIAN_POINT('Ctrl Pts',(76.2422338085695,79.348965170643,205.035416665711));
#29271=CARTESIAN_POINT('Ctrl Pts',(76.9272727088508,79.1823476029926,205.093749999044));
#29272=CARTESIAN_POINT('Ctrl Pts',(77.6123116091322,79.0157300353421,205.152083332377));
#29273=CARTESIAN_POINT('Ctrl Pts',(78.099126105575,79.5256823417411,205.210416665711));
#29274=CARTESIAN_POINT('Ctrl Pts',(78.5859406020177,80.03563464814,205.268749999044));
#29275=CARTESIAN_POINT('Ctrl Pts',(78.3877161981791,80.7122045221895,205.327083332377));
#29276=CARTESIAN_POINT('Ctrl Pts',(78.1894917943405,81.388774396239,205.385416665711));
#29277=CARTESIAN_POINT('Ctrl Pts',(77.5044528940591,81.5553919638894,205.443749999044));
#29278=CARTESIAN_POINT('Ctrl Pts',(77.5044528940591,81.5553919638894,204.568749999044));
#29279=CARTESIAN_POINT('Ctrl Pts',(76.8194139937778,81.7220095315399,204.627083332377));
#29280=CARTESIAN_POINT('Ctrl Pts',(76.332599497335,81.2120572251409,204.685416665711));
#29281=CARTESIAN_POINT('Ctrl Pts',(75.8457850008923,80.7021049187419,204.743749999044));
#29282=CARTESIAN_POINT('Ctrl Pts',(76.0440094047309,80.0255350446925,204.802083332377));
#29283=CARTESIAN_POINT('Ctrl Pts',(76.2422338085695,79.348965170643,204.860416665711));
#29284=CARTESIAN_POINT('Ctrl Pts',(76.9272727088508,79.1823476029926,204.918749999044));
#29285=CARTESIAN_POINT('Ctrl Pts',(77.6123116091322,79.0157300353421,204.977083332377));
#29286=CARTESIAN_POINT('Ctrl Pts',(78.099126105575,79.5256823417411,205.035416665711));
#29287=CARTESIAN_POINT('Ctrl Pts',(78.5859406020177,80.03563464814,205.093749999044));
#29288=CARTESIAN_POINT('Ctrl Pts',(78.3877161981791,80.7122045221895,205.152083332377));
#29289=CARTESIAN_POINT('Ctrl Pts',(78.1894917943405,81.388774396239,205.210416665711));
#29290=CARTESIAN_POINT('Ctrl Pts',(77.5044528940591,81.5553919638894,205.268749999044));
#29291=CARTESIAN_POINT('Origin',(77.2158628014549,80.3688697834408,198.006249999044));
#29292=CARTESIAN_POINT('',(77.5044528940591,81.5553919638894,203.868749999044));
#29293=CARTESIAN_POINT('',(77.5044528940591,81.5553919638894,204.043749999044));
#29294=CARTESIAN_POINT('',(77.504452894059,81.555391963889,198.006249999044));
#29295=CARTESIAN_POINT('Ctrl Pts',(77.5044528940591,81.5553919638894,204.043749999044));
#29296=CARTESIAN_POINT('Ctrl Pts',(76.8194139937778,81.7220095315399,204.102083332377));
#29297=CARTESIAN_POINT('Ctrl Pts',(76.332599497335,81.2120572251409,204.160416665711));
#29298=CARTESIAN_POINT('Ctrl Pts',(75.8457850008923,80.7021049187419,204.218749999044));
#29299=CARTESIAN_POINT('Ctrl Pts',(76.0440094047309,80.0255350446925,204.277083332377));
#29300=CARTESIAN_POINT('Ctrl Pts',(76.2422338085695,79.348965170643,204.335416665711));
#29301=CARTESIAN_POINT('Ctrl Pts',(76.9272727088508,79.1823476029926,204.393749999044));
#29302=CARTESIAN_POINT('Ctrl Pts',(77.6123116091322,79.0157300353421,204.452083332377));
#29303=CARTESIAN_POINT('Ctrl Pts',(78.099126105575,79.5256823417411,204.510416665711));
#29304=CARTESIAN_POINT('Ctrl Pts',(78.5859406020177,80.03563464814,204.568749999044));
#29305=CARTESIAN_POINT('Ctrl Pts',(78.3877161981791,80.7122045221895,204.627083332377));
#29306=CARTESIAN_POINT('Ctrl Pts',(78.1894917943405,81.388774396239,204.685416665711));
#29307=CARTESIAN_POINT('Ctrl Pts',(77.5044528940591,81.5553919638894,204.743749999044));
#29308=CARTESIAN_POINT('Ctrl Pts',(77.5044528940591,81.5553919638894,203.868749999044));
#29309=CARTESIAN_POINT('Ctrl Pts',(76.8194139937778,81.7220095315399,203.927083332377));
#29310=CARTESIAN_POINT('Ctrl Pts',(76.332599497335,81.2120572251409,203.985416665711));
#29311=CARTESIAN_POINT('Ctrl Pts',(75.8457850008923,80.7021049187419,204.043749999044));
#29312=CARTESIAN_POINT('Ctrl Pts',(76.0440094047309,80.0255350446925,204.102083332377));
#29313=CARTESIAN_POINT('Ctrl Pts',(76.2422338085695,79.348965170643,204.160416665711));
#29314=CARTESIAN_POINT('Ctrl Pts',(76.9272727088508,79.1823476029926,204.218749999044));
#29315=CARTESIAN_POINT('Ctrl Pts',(77.6123116091322,79.0157300353421,204.277083332377));
#29316=CARTESIAN_POINT('Ctrl Pts',(78.099126105575,79.5256823417411,204.335416665711));
#29317=CARTESIAN_POINT('Ctrl Pts',(78.5859406020177,80.03563464814,204.393749999044));
#29318=CARTESIAN_POINT('Ctrl Pts',(78.3877161981791,80.7122045221895,204.452083332377));
#29319=CARTESIAN_POINT('Ctrl Pts',(78.1894917943405,81.388774396239,204.510416665711));
#29320=CARTESIAN_POINT('Ctrl Pts',(77.5044528940591,81.5553919638894,204.568749999044));
#29321=CARTESIAN_POINT('Origin',(77.2158628014549,80.3688697834408,198.006249999044));
#29322=CARTESIAN_POINT('',(77.5044528940591,81.5553919638894,203.168749999044));
#29323=CARTESIAN_POINT('',(77.5044528940591,81.5553919638894,203.343749999044));
#29324=CARTESIAN_POINT('',(77.504452894059,81.555391963889,198.006249999044));
#29325=CARTESIAN_POINT('Ctrl Pts',(77.5044528940591,81.5553919638894,203.343749999044));
#29326=CARTESIAN_POINT('Ctrl Pts',(76.8194139937778,81.7220095315399,203.402083332378));
#29327=CARTESIAN_POINT('Ctrl Pts',(76.332599497335,81.2120572251409,203.460416665711));
#29328=CARTESIAN_POINT('Ctrl Pts',(75.8457850008923,80.7021049187419,203.518749999044));
#29329=CARTESIAN_POINT('Ctrl Pts',(76.0440094047309,80.0255350446925,203.577083332377));
#29330=CARTESIAN_POINT('Ctrl Pts',(76.2422338085695,79.348965170643,203.635416665711));
#29331=CARTESIAN_POINT('Ctrl Pts',(76.9272727088508,79.1823476029926,203.693749999044));
#29332=CARTESIAN_POINT('Ctrl Pts',(77.6123116091322,79.0157300353421,203.752083332377));
#29333=CARTESIAN_POINT('Ctrl Pts',(78.099126105575,79.5256823417411,203.810416665711));
#29334=CARTESIAN_POINT('Ctrl Pts',(78.5859406020177,80.03563464814,203.868749999044));
#29335=CARTESIAN_POINT('Ctrl Pts',(78.3877161981791,80.7122045221895,203.927083332377));
#29336=CARTESIAN_POINT('Ctrl Pts',(78.1894917943405,81.388774396239,203.985416665711));
#29337=CARTESIAN_POINT('Ctrl Pts',(77.5044528940591,81.5553919638894,204.043749999044));
#29338=CARTESIAN_POINT('Ctrl Pts',(77.5044528940591,81.5553919638894,203.168749999044));
#29339=CARTESIAN_POINT('Ctrl Pts',(76.8194139937778,81.7220095315399,203.227083332378));
#29340=CARTESIAN_POINT('Ctrl Pts',(76.332599497335,81.2120572251409,203.285416665711));
#29341=CARTESIAN_POINT('Ctrl Pts',(75.8457850008923,80.7021049187419,203.343749999044));
#29342=CARTESIAN_POINT('Ctrl Pts',(76.0440094047309,80.0255350446925,203.402083332377));
#29343=CARTESIAN_POINT('Ctrl Pts',(76.2422338085695,79.348965170643,203.460416665711));
#29344=CARTESIAN_POINT('Ctrl Pts',(76.9272727088508,79.1823476029926,203.518749999044));
#29345=CARTESIAN_POINT('Ctrl Pts',(77.6123116091322,79.0157300353421,203.577083332377));
#29346=CARTESIAN_POINT('Ctrl Pts',(78.099126105575,79.5256823417411,203.635416665711));
#29347=CARTESIAN_POINT('Ctrl Pts',(78.5859406020177,80.0356346481401,203.693749999044));
#29348=CARTESIAN_POINT('Ctrl Pts',(78.3877161981791,80.7122045221895,203.752083332377));
#29349=CARTESIAN_POINT('Ctrl Pts',(78.1894917943405,81.388774396239,203.810416665711));
#29350=CARTESIAN_POINT('Ctrl Pts',(77.5044528940591,81.5553919638894,203.868749999044));
#29351=CARTESIAN_POINT('Origin',(77.2158628014549,80.3688697834408,198.006249999044));
#29352=CARTESIAN_POINT('',(77.5044528940591,81.5553919638894,202.468749999044));
#29353=CARTESIAN_POINT('',(77.5044528940591,81.5553919638894,202.643749999044));
#29354=CARTESIAN_POINT('',(77.504452894059,81.555391963889,198.006249999044));
#29355=CARTESIAN_POINT('Ctrl Pts',(77.5044528940591,81.5553919638894,202.643749999044));
#29356=CARTESIAN_POINT('Ctrl Pts',(76.8194139937778,81.7220095315399,202.702083332377));
#29357=CARTESIAN_POINT('Ctrl Pts',(76.332599497335,81.2120572251409,202.760416665711));
#29358=CARTESIAN_POINT('Ctrl Pts',(75.8457850008923,80.7021049187419,202.818749999044));
#29359=CARTESIAN_POINT('Ctrl Pts',(76.0440094047309,80.0255350446925,202.877083332377));
#29360=CARTESIAN_POINT('Ctrl Pts',(76.2422338085695,79.348965170643,202.935416665711));
#29361=CARTESIAN_POINT('Ctrl Pts',(76.9272727088508,79.1823476029926,202.993749999044));
#29362=CARTESIAN_POINT('Ctrl Pts',(77.6123116091322,79.0157300353421,203.052083332377));
#29363=CARTESIAN_POINT('Ctrl Pts',(78.099126105575,79.5256823417411,203.110416665711));
#29364=CARTESIAN_POINT('Ctrl Pts',(78.5859406020177,80.0356346481401,203.168749999044));
#29365=CARTESIAN_POINT('Ctrl Pts',(78.3877161981791,80.7122045221895,203.227083332377));
#29366=CARTESIAN_POINT('Ctrl Pts',(78.1894917943405,81.388774396239,203.285416665711));
#29367=CARTESIAN_POINT('Ctrl Pts',(77.5044528940591,81.5553919638894,203.343749999044));
#29368=CARTESIAN_POINT('Ctrl Pts',(77.5044528940591,81.5553919638894,202.468749999044));
#29369=CARTESIAN_POINT('Ctrl Pts',(76.8194139937778,81.7220095315399,202.527083332377));
#29370=CARTESIAN_POINT('Ctrl Pts',(76.332599497335,81.2120572251409,202.585416665711));
#29371=CARTESIAN_POINT('Ctrl Pts',(75.8457850008923,80.702104918742,202.643749999044));
#29372=CARTESIAN_POINT('Ctrl Pts',(76.0440094047309,80.0255350446925,202.702083332377));
#29373=CARTESIAN_POINT('Ctrl Pts',(76.2422338085695,79.348965170643,202.760416665711));
#29374=CARTESIAN_POINT('Ctrl Pts',(76.9272727088508,79.1823476029926,202.818749999044));
#29375=CARTESIAN_POINT('Ctrl Pts',(77.6123116091322,79.0157300353421,202.877083332377));
#29376=CARTESIAN_POINT('Ctrl Pts',(78.099126105575,79.5256823417411,202.935416665711));
#29377=CARTESIAN_POINT('Ctrl Pts',(78.5859406020177,80.0356346481401,202.993749999044));
#29378=CARTESIAN_POINT('Ctrl Pts',(78.3877161981791,80.7122045221895,203.052083332377));
#29379=CARTESIAN_POINT('Ctrl Pts',(78.1894917943405,81.388774396239,203.110416665711));
#29380=CARTESIAN_POINT('Ctrl Pts',(77.5044528940591,81.5553919638894,203.168749999044));
#29381=CARTESIAN_POINT('Origin',(77.2158628014549,80.3688697834408,198.006249999044));
#29382=CARTESIAN_POINT('',(77.5044528940591,81.5553919638894,201.768749999044));
#29383=CARTESIAN_POINT('',(77.5044528940591,81.5553919638894,201.943749999044));
#29384=CARTESIAN_POINT('',(77.504452894059,81.555391963889,198.006249999044));
#29385=CARTESIAN_POINT('Ctrl Pts',(77.5044528940591,81.5553919638894,201.943749999044));
#29386=CARTESIAN_POINT('Ctrl Pts',(76.8194139937778,81.7220095315399,202.002083332377));
#29387=CARTESIAN_POINT('Ctrl Pts',(76.332599497335,81.2120572251409,202.060416665711));
#29388=CARTESIAN_POINT('Ctrl Pts',(75.8457850008923,80.702104918742,202.118749999044));
#29389=CARTESIAN_POINT('Ctrl Pts',(76.0440094047309,80.0255350446925,202.177083332377));
#29390=CARTESIAN_POINT('Ctrl Pts',(76.2422338085695,79.348965170643,202.235416665711));
#29391=CARTESIAN_POINT('Ctrl Pts',(76.9272727088508,79.1823476029926,202.293749999044));
#29392=CARTESIAN_POINT('Ctrl Pts',(77.6123116091322,79.0157300353421,202.352083332377));
#29393=CARTESIAN_POINT('Ctrl Pts',(78.099126105575,79.5256823417411,202.410416665711));
#29394=CARTESIAN_POINT('Ctrl Pts',(78.5859406020177,80.0356346481401,202.468749999044));
#29395=CARTESIAN_POINT('Ctrl Pts',(78.3877161981791,80.7122045221895,202.527083332377));
#29396=CARTESIAN_POINT('Ctrl Pts',(78.1894917943405,81.388774396239,202.585416665711));
#29397=CARTESIAN_POINT('Ctrl Pts',(77.5044528940591,81.5553919638894,202.643749999044));
#29398=CARTESIAN_POINT('Ctrl Pts',(77.5044528940591,81.5553919638894,201.768749999044));
#29399=CARTESIAN_POINT('Ctrl Pts',(76.8194139937778,81.7220095315399,201.827083332377));
#29400=CARTESIAN_POINT('Ctrl Pts',(76.332599497335,81.2120572251409,201.885416665711));
#29401=CARTESIAN_POINT('Ctrl Pts',(75.8457850008923,80.702104918742,201.943749999044));
#29402=CARTESIAN_POINT('Ctrl Pts',(76.0440094047309,80.0255350446925,202.002083332377));
#29403=CARTESIAN_POINT('Ctrl Pts',(76.2422338085695,79.348965170643,202.060416665711));
#29404=CARTESIAN_POINT('Ctrl Pts',(76.9272727088508,79.1823476029926,202.118749999044));
#29405=CARTESIAN_POINT('Ctrl Pts',(77.6123116091322,79.0157300353421,202.177083332377));
#29406=CARTESIAN_POINT('Ctrl Pts',(78.099126105575,79.5256823417411,202.235416665711));
#29407=CARTESIAN_POINT('Ctrl Pts',(78.5859406020177,80.0356346481401,202.293749999044));
#29408=CARTESIAN_POINT('Ctrl Pts',(78.3877161981791,80.7122045221895,202.352083332377));
#29409=CARTESIAN_POINT('Ctrl Pts',(78.1894917943405,81.388774396239,202.410416665711));
#29410=CARTESIAN_POINT('Ctrl Pts',(77.5044528940591,81.5553919638894,202.468749999044));
#29411=CARTESIAN_POINT('Origin',(77.2158628014549,80.3688697834408,198.006249999044));
#29412=CARTESIAN_POINT('',(77.5044528940591,81.5553919638894,201.068749999044));
#29413=CARTESIAN_POINT('',(77.5044528940591,81.5553919638894,201.243749999044));
#29414=CARTESIAN_POINT('',(77.504452894059,81.555391963889,198.006249999044));
#29415=CARTESIAN_POINT('Ctrl Pts',(77.5044528940591,81.5553919638894,201.243749999044));
#29416=CARTESIAN_POINT('Ctrl Pts',(76.8194139937778,81.7220095315399,201.302083332377));
#29417=CARTESIAN_POINT('Ctrl Pts',(76.332599497335,81.2120572251409,201.360416665711));
#29418=CARTESIAN_POINT('Ctrl Pts',(75.8457850008923,80.702104918742,201.418749999044));
#29419=CARTESIAN_POINT('Ctrl Pts',(76.0440094047309,80.0255350446925,201.477083332377));
#29420=CARTESIAN_POINT('Ctrl Pts',(76.2422338085695,79.348965170643,201.535416665711));
#29421=CARTESIAN_POINT('Ctrl Pts',(76.9272727088508,79.1823476029926,201.593749999044));
#29422=CARTESIAN_POINT('Ctrl Pts',(77.6123116091322,79.0157300353421,201.652083332377));
#29423=CARTESIAN_POINT('Ctrl Pts',(78.099126105575,79.5256823417411,201.710416665711));
#29424=CARTESIAN_POINT('Ctrl Pts',(78.5859406020177,80.0356346481401,201.768749999044));
#29425=CARTESIAN_POINT('Ctrl Pts',(78.3877161981791,80.7122045221895,201.827083332377));
#29426=CARTESIAN_POINT('Ctrl Pts',(78.1894917943405,81.388774396239,201.885416665711));
#29427=CARTESIAN_POINT('Ctrl Pts',(77.5044528940591,81.5553919638894,201.943749999044));
#29428=CARTESIAN_POINT('Ctrl Pts',(77.5044528940591,81.5553919638894,201.068749999044));
#29429=CARTESIAN_POINT('Ctrl Pts',(76.8194139937778,81.7220095315399,201.127083332377));
#29430=CARTESIAN_POINT('Ctrl Pts',(76.332599497335,81.2120572251409,201.185416665711));
#29431=CARTESIAN_POINT('Ctrl Pts',(75.8457850008923,80.702104918742,201.243749999044));
#29432=CARTESIAN_POINT('Ctrl Pts',(76.0440094047309,80.0255350446925,201.302083332377));
#29433=CARTESIAN_POINT('Ctrl Pts',(76.2422338085695,79.348965170643,201.360416665711));
#29434=CARTESIAN_POINT('Ctrl Pts',(76.9272727088508,79.1823476029926,201.418749999044));
#29435=CARTESIAN_POINT('Ctrl Pts',(77.6123116091322,79.0157300353421,201.477083332377));
#29436=CARTESIAN_POINT('Ctrl Pts',(78.099126105575,79.5256823417411,201.535416665711));
#29437=CARTESIAN_POINT('Ctrl Pts',(78.5859406020177,80.0356346481401,201.593749999044));
#29438=CARTESIAN_POINT('Ctrl Pts',(78.3877161981791,80.7122045221895,201.652083332377));
#29439=CARTESIAN_POINT('Ctrl Pts',(78.1894917943405,81.388774396239,201.710416665711));
#29440=CARTESIAN_POINT('Ctrl Pts',(77.5044528940591,81.5553919638894,201.768749999044));
#29441=CARTESIAN_POINT('Origin',(77.2158628014549,80.3688697834408,198.006249999044));
#29442=CARTESIAN_POINT('',(77.5044528940591,81.5553919638894,200.368749999044));
#29443=CARTESIAN_POINT('',(77.5044528940591,81.5553919638894,200.543749999044));
#29444=CARTESIAN_POINT('',(77.504452894059,81.555391963889,198.006249999044));
#29445=CARTESIAN_POINT('Ctrl Pts',(77.5044528940591,81.5553919638894,200.543749999044));
#29446=CARTESIAN_POINT('Ctrl Pts',(76.8194139937778,81.7220095315399,200.602083332377));
#29447=CARTESIAN_POINT('Ctrl Pts',(76.332599497335,81.2120572251409,200.660416665711));
#29448=CARTESIAN_POINT('Ctrl Pts',(75.8457850008923,80.702104918742,200.718749999044));
#29449=CARTESIAN_POINT('Ctrl Pts',(76.0440094047309,80.0255350446925,200.777083332377));
#29450=CARTESIAN_POINT('Ctrl Pts',(76.2422338085695,79.348965170643,200.835416665711));
#29451=CARTESIAN_POINT('Ctrl Pts',(76.9272727088508,79.1823476029926,200.893749999044));
#29452=CARTESIAN_POINT('Ctrl Pts',(77.6123116091322,79.0157300353421,200.952083332377));
#29453=CARTESIAN_POINT('Ctrl Pts',(78.099126105575,79.5256823417411,201.010416665711));
#29454=CARTESIAN_POINT('Ctrl Pts',(78.5859406020177,80.0356346481401,201.068749999044));
#29455=CARTESIAN_POINT('Ctrl Pts',(78.3877161981791,80.7122045221895,201.127083332377));
#29456=CARTESIAN_POINT('Ctrl Pts',(78.1894917943405,81.388774396239,201.185416665711));
#29457=CARTESIAN_POINT('Ctrl Pts',(77.5044528940591,81.5553919638894,201.243749999044));
#29458=CARTESIAN_POINT('Ctrl Pts',(77.5044528940591,81.5553919638894,200.368749999044));
#29459=CARTESIAN_POINT('Ctrl Pts',(76.8194139937778,81.7220095315399,200.427083332377));
#29460=CARTESIAN_POINT('Ctrl Pts',(76.332599497335,81.2120572251409,200.485416665711));
#29461=CARTESIAN_POINT('Ctrl Pts',(75.8457850008923,80.702104918742,200.543749999044));
#29462=CARTESIAN_POINT('Ctrl Pts',(76.0440094047309,80.0255350446925,200.602083332377));
#29463=CARTESIAN_POINT('Ctrl Pts',(76.2422338085695,79.348965170643,200.660416665711));
#29464=CARTESIAN_POINT('Ctrl Pts',(76.9272727088508,79.1823476029926,200.718749999044));
#29465=CARTESIAN_POINT('Ctrl Pts',(77.6123116091322,79.0157300353421,200.777083332377));
#29466=CARTESIAN_POINT('Ctrl Pts',(78.099126105575,79.5256823417411,200.835416665711));
#29467=CARTESIAN_POINT('Ctrl Pts',(78.5859406020177,80.0356346481401,200.893749999044));
#29468=CARTESIAN_POINT('Ctrl Pts',(78.3877161981791,80.7122045221895,200.952083332377));
#29469=CARTESIAN_POINT('Ctrl Pts',(78.1894917943405,81.388774396239,201.010416665711));
#29470=CARTESIAN_POINT('Ctrl Pts',(77.5044528940591,81.5553919638894,201.068749999044));
#29471=CARTESIAN_POINT('Origin',(77.2158628014549,80.3688697834408,198.006249999044));
#29472=CARTESIAN_POINT('',(77.5044528940591,81.5553919638894,199.668749999044));
#29473=CARTESIAN_POINT('',(77.5044528940591,81.5553919638894,199.843749999044));
#29474=CARTESIAN_POINT('',(77.504452894059,81.555391963889,198.006249999044));
#29475=CARTESIAN_POINT('Ctrl Pts',(77.5044528940591,81.5553919638894,199.843749999044));
#29476=CARTESIAN_POINT('Ctrl Pts',(76.8194139937778,81.7220095315399,199.902083332377));
#29477=CARTESIAN_POINT('Ctrl Pts',(76.332599497335,81.2120572251409,199.960416665711));
#29478=CARTESIAN_POINT('Ctrl Pts',(75.8457850008923,80.702104918742,200.018749999044));
#29479=CARTESIAN_POINT('Ctrl Pts',(76.0440094047309,80.0255350446925,200.077083332377));
#29480=CARTESIAN_POINT('Ctrl Pts',(76.2422338085695,79.3489651706431,200.135416665711));
#29481=CARTESIAN_POINT('Ctrl Pts',(76.9272727088508,79.1823476029926,200.193749999044));
#29482=CARTESIAN_POINT('Ctrl Pts',(77.6123116091322,79.0157300353421,200.252083332377));
#29483=CARTESIAN_POINT('Ctrl Pts',(78.099126105575,79.5256823417411,200.310416665711));
#29484=CARTESIAN_POINT('Ctrl Pts',(78.5859406020177,80.0356346481401,200.368749999044));
#29485=CARTESIAN_POINT('Ctrl Pts',(78.3877161981791,80.7122045221895,200.427083332377));
#29486=CARTESIAN_POINT('Ctrl Pts',(78.1894917943405,81.388774396239,200.485416665711));
#29487=CARTESIAN_POINT('Ctrl Pts',(77.5044528940591,81.5553919638894,200.543749999044));
#29488=CARTESIAN_POINT('Ctrl Pts',(77.5044528940591,81.5553919638894,199.668749999044));
#29489=CARTESIAN_POINT('Ctrl Pts',(76.8194139937778,81.7220095315399,199.727083332377));
#29490=CARTESIAN_POINT('Ctrl Pts',(76.332599497335,81.2120572251409,199.785416665711));
#29491=CARTESIAN_POINT('Ctrl Pts',(75.8457850008923,80.702104918742,199.843749999044));
#29492=CARTESIAN_POINT('Ctrl Pts',(76.0440094047309,80.0255350446925,199.902083332377));
#29493=CARTESIAN_POINT('Ctrl Pts',(76.2422338085695,79.3489651706431,199.960416665711));
#29494=CARTESIAN_POINT('Ctrl Pts',(76.9272727088508,79.1823476029926,200.018749999044));
#29495=CARTESIAN_POINT('Ctrl Pts',(77.6123116091322,79.0157300353421,200.077083332377));
#29496=CARTESIAN_POINT('Ctrl Pts',(78.099126105575,79.5256823417411,200.135416665711));
#29497=CARTESIAN_POINT('Ctrl Pts',(78.5859406020177,80.0356346481401,200.193749999044));
#29498=CARTESIAN_POINT('Ctrl Pts',(78.3877161981791,80.7122045221895,200.252083332377));
#29499=CARTESIAN_POINT('Ctrl Pts',(78.1894917943405,81.388774396239,200.310416665711));
#29500=CARTESIAN_POINT('Ctrl Pts',(77.5044528940591,81.5553919638894,200.368749999044));
#29501=CARTESIAN_POINT('Origin',(77.2158628014549,80.3688697834408,198.006249999044));
#29502=CARTESIAN_POINT('',(77.5044528940591,81.5553919638894,198.968749999044));
#29503=CARTESIAN_POINT('',(77.5044528940591,81.5553919638894,199.143749999044));
#29504=CARTESIAN_POINT('',(77.504452894059,81.555391963889,198.006249999044));
#29505=CARTESIAN_POINT('Ctrl Pts',(77.5044528940591,81.5553919638894,199.143749999044));
#29506=CARTESIAN_POINT('Ctrl Pts',(76.8194139937778,81.7220095315399,199.202083332377));
#29507=CARTESIAN_POINT('Ctrl Pts',(76.332599497335,81.2120572251409,199.260416665711));
#29508=CARTESIAN_POINT('Ctrl Pts',(75.8457850008923,80.702104918742,199.318749999044));
#29509=CARTESIAN_POINT('Ctrl Pts',(76.0440094047309,80.0255350446925,199.377083332377));
#29510=CARTESIAN_POINT('Ctrl Pts',(76.2422338085695,79.3489651706431,199.435416665711));
#29511=CARTESIAN_POINT('Ctrl Pts',(76.9272727088509,79.1823476029926,199.493749999044));
#29512=CARTESIAN_POINT('Ctrl Pts',(77.6123116091322,79.0157300353421,199.552083332377));
#29513=CARTESIAN_POINT('Ctrl Pts',(78.099126105575,79.5256823417411,199.610416665711));
#29514=CARTESIAN_POINT('Ctrl Pts',(78.5859406020177,80.0356346481401,199.668749999044));
#29515=CARTESIAN_POINT('Ctrl Pts',(78.3877161981791,80.7122045221895,199.727083332377));
#29516=CARTESIAN_POINT('Ctrl Pts',(78.1894917943405,81.388774396239,199.785416665711));
#29517=CARTESIAN_POINT('Ctrl Pts',(77.5044528940591,81.5553919638894,199.843749999044));
#29518=CARTESIAN_POINT('Ctrl Pts',(77.5044528940591,81.5553919638894,198.968749999044));
#29519=CARTESIAN_POINT('Ctrl Pts',(76.8194139937778,81.7220095315399,199.027083332377));
#29520=CARTESIAN_POINT('Ctrl Pts',(76.332599497335,81.2120572251409,199.085416665711));
#29521=CARTESIAN_POINT('Ctrl Pts',(75.8457850008923,80.702104918742,199.143749999044));
#29522=CARTESIAN_POINT('Ctrl Pts',(76.0440094047309,80.0255350446925,199.202083332377));
#29523=CARTESIAN_POINT('Ctrl Pts',(76.2422338085695,79.3489651706431,199.260416665711));
#29524=CARTESIAN_POINT('Ctrl Pts',(76.9272727088509,79.1823476029926,199.318749999044));
#29525=CARTESIAN_POINT('Ctrl Pts',(77.6123116091322,79.0157300353421,199.377083332377));
#29526=CARTESIAN_POINT('Ctrl Pts',(78.099126105575,79.5256823417411,199.435416665711));
#29527=CARTESIAN_POINT('Ctrl Pts',(78.5859406020177,80.0356346481401,199.493749999044));
#29528=CARTESIAN_POINT('Ctrl Pts',(78.3877161981791,80.7122045221895,199.552083332377));
#29529=CARTESIAN_POINT('Ctrl Pts',(78.1894917943405,81.388774396239,199.610416665711));
#29530=CARTESIAN_POINT('Ctrl Pts',(77.5044528940591,81.5553919638894,199.668749999044));
#29531=CARTESIAN_POINT('Origin',(77.2158628014549,80.3688697834408,198.006249999044));
#29532=CARTESIAN_POINT('',(77.5044528940591,81.5553919638894,198.268749999044));
#29533=CARTESIAN_POINT('',(77.5044528940591,81.5553919638894,198.443749999044));
#29534=CARTESIAN_POINT('',(77.504452894059,81.555391963889,198.006249999044));
#29535=CARTESIAN_POINT('',(76.9272727088509,79.1823476029926,197.918749999044));
#29536=CARTESIAN_POINT('Ctrl Pts',(76.9272727088509,79.1823476029926,197.918749999044));
#29537=CARTESIAN_POINT('Ctrl Pts',(77.6123116091322,79.0157300353421,197.977083332377));
#29538=CARTESIAN_POINT('Ctrl Pts',(78.099126105575,79.5256823417411,198.035416665711));
#29539=CARTESIAN_POINT('Ctrl Pts',(78.5859406020177,80.0356346481401,198.093749999044));
#29540=CARTESIAN_POINT('Ctrl Pts',(78.3877161981791,80.7122045221895,198.152083332377));
#29541=CARTESIAN_POINT('Ctrl Pts',(78.1894917943405,81.388774396239,198.210416665711));
#29542=CARTESIAN_POINT('Ctrl Pts',(77.5044528940591,81.5553919638894,198.268749999044));
#29543=CARTESIAN_POINT('',(76.9272727088509,79.1823476029926,198.093749999044));
#29544=CARTESIAN_POINT('',(76.9272727088509,79.1823476029926,198.006249999044));
#29545=CARTESIAN_POINT('Ctrl Pts',(76.9272727088509,79.1823476029926,198.093749999044));
#29546=CARTESIAN_POINT('Ctrl Pts',(77.6123116091322,79.0157300353421,198.152083332378));
#29547=CARTESIAN_POINT('Ctrl Pts',(78.099126105575,79.5256823417411,198.210416665711));
#29548=CARTESIAN_POINT('Ctrl Pts',(78.5859406020177,80.0356346481401,198.268749999044));
#29549=CARTESIAN_POINT('Ctrl Pts',(78.3877161981791,80.7122045221895,198.327083332377));
#29550=CARTESIAN_POINT('Ctrl Pts',(78.1894917943405,81.388774396239,198.385416665711));
#29551=CARTESIAN_POINT('Ctrl Pts',(77.5044528940591,81.5553919638894,198.443749999044));
#29552=CARTESIAN_POINT('Origin',(77.215862801455,80.3688697834411,196.));
#29553=CARTESIAN_POINT('',(79.2246973681942,88.6280818332357,204.25));
#29554=CARTESIAN_POINT('',(79.2246973681943,88.6280818332357,204.062499995903));
#29555=CARTESIAN_POINT('',(79.2246973681942,88.6280818332357,196.));
#29556=CARTESIAN_POINT('',(72.3914232244021,87.3670683207337,202.950490121702));
#29557=CARTESIAN_POINT('Ctrl Pts',(72.3914232244021,87.3670683207337,202.950490121702));
#29558=CARTESIAN_POINT('Ctrl Pts',(71.8866410030934,87.0190800044125,202.967172868051));
#29559=CARTESIAN_POINT('Ctrl Pts',(71.4210052486793,86.6175094622243,202.984436404133));
#29560=CARTESIAN_POINT('Ctrl Pts',(70.5787635197524,85.715337435547,203.01975318524));
#29561=CARTESIAN_POINT('Ctrl Pts',(70.2059380614513,85.2162151353597,203.037707708689));
#29562=CARTESIAN_POINT('Ctrl Pts',(69.3281756281021,83.7251393098489,203.087330386574));
#29563=CARTESIAN_POINT('Ctrl Pts',(68.9580012473484,82.668401936068,203.116727001829));
#29564=CARTESIAN_POINT('Ctrl Pts',(68.6452620704762,80.4782567768875,203.177718055383));
#29565=CARTESIAN_POINT('Ctrl Pts',(68.7034266927971,79.3661137029368,203.209648851176));
#29566=CARTESIAN_POINT('Ctrl Pts',(69.2432554551038,77.2191089181655,203.273183071381));
#29567=CARTESIAN_POINT('Ctrl Pts',(69.7225545707681,76.205486960677,203.302726170008));
#29568=CARTESIAN_POINT('Ctrl Pts',(71.0390106890496,74.4264730124253,203.363616273261));
#29569=CARTESIAN_POINT('Ctrl Pts',(71.8610437967351,73.6762308356727,203.395503603533));
#29570=CARTESIAN_POINT('Ctrl Pts',(73.7538572107139,72.5265957263018,203.459097812285));
#29571=CARTESIAN_POINT('Ctrl Pts',(74.8084645726234,72.1414076437613,203.488789499096));
#29572=CARTESIAN_POINT('Ctrl Pts',(76.9959887135032,71.8005722002156,203.54958160803));
#29573=CARTESIAN_POINT('Ctrl Pts',(78.1073488517799,71.8442444202341,203.581425991173));
#29574=CARTESIAN_POINT('Ctrl Pts',(80.2627901024727,72.3559911613201,203.645076243339));
#29575=CARTESIAN_POINT('Ctrl Pts',(81.2851662350286,72.8236259817403,203.67491753275));
#29576=CARTESIAN_POINT('Ctrl Pts',(83.0813896544156,74.1192123802627,203.73561480348));
#29577=CARTESIAN_POINT('Ctrl Pts',(83.8408482567561,74.9308459382432,203.767416943822));
#29578=CARTESIAN_POINT('Ctrl Pts',(85.0151855726337,76.8102540662147,203.831119441553));
#29579=CARTESIAN_POINT('Ctrl Pts',(85.4142237057403,77.8628781075825,203.861110334641));
#29580=CARTESIAN_POINT('Ctrl Pts',(85.7808027993859,80.0478577829302,203.921716087211));
#29581=CARTESIAN_POINT('Ctrl Pts',(85.7503746510489,81.1583392967423,203.953476855176));
#29582=CARTESIAN_POINT('Ctrl Pts',(85.2644213488685,83.3213286029071,204.01722796243));
#29583=CARTESIAN_POINT('Ctrl Pts',(84.8075074237539,84.3517284345946,204.047367533357));
#29584=CARTESIAN_POINT('Ctrl Pts',(83.531047351044,86.1635553311158,204.107885216322));
#29585=CARTESIAN_POINT('Ctrl Pts',(82.7289789307318,86.9312925102494,204.139605627809));
#29586=CARTESIAN_POINT('Ctrl Pts',(81.0095420444879,88.0334763293615,204.198358840566));
#29587=CARTESIAN_POINT('Ctrl Pts',(80.1380923292335,88.4059227023454,204.224969648026));
#29588=CARTESIAN_POINT('Ctrl Pts',(79.2246973681942,88.6280818332357,204.25));
#29589=CARTESIAN_POINT('',(68.8559951920602,81.9059493368122,202.950490121702));
#29590=CARTESIAN_POINT('Origin',(77.215862801455,80.368869783441,202.950490121702));
#29591=CARTESIAN_POINT('Ctrl Pts',(79.2246973681943,88.6280818332357,204.062499995903));
#29592=CARTESIAN_POINT('Ctrl Pts',(79.423283621529,88.5797809871292,204.057058008559));
#29593=CARTESIAN_POINT('Ctrl Pts',(79.6203365987936,88.5242672453642,204.051529004407));
#29594=CARTESIAN_POINT('Ctrl Pts',(80.8896901414571,88.1165169205814,204.015059875846));
#29595=CARTESIAN_POINT('Ctrl Pts',(81.8845174455793,87.5609913684401,203.982464351867));
#29596=CARTESIAN_POINT('Ctrl Pts',(83.5685697934855,86.1201326713807,203.918773583326));
#29597=CARTESIAN_POINT('Ctrl Pts',(84.2518515672673,85.2605668161688,203.889436476945));
#29598=CARTESIAN_POINT('Ctrl Pts',(85.2760200246701,83.2943364473811,203.828907917564));
#29599=CARTESIAN_POINT('Ctrl Pts',(85.59287874222,82.1991688982689,203.796316107443));
#29600=CARTESIAN_POINT('Ctrl Pts',(85.7768504176493,79.9896690547137,203.732576372513));
#29601=CARTESIAN_POINT('Ctrl Pts',(85.6580421040234,78.8978746755789,203.703125859407));
#29602=CARTESIAN_POINT('Ctrl Pts',(85.002978577606,76.7790656498003,203.642686154301));
#29603=CARTESIAN_POINT('Ctrl Pts',(84.4575669291109,75.7771942401416,203.610098775639));
#29604=CARTESIAN_POINT('Ctrl Pts',(83.0334840710811,74.0768095521821,203.546313367191));
#29605=CARTESIAN_POINT('Ctrl Pts',(82.1808156244406,73.3843234751008,203.516750361292));
#29606=CARTESIAN_POINT('Ctrl Pts',(80.2239717765268,72.3390221629042,203.456395634484));
#29607=CARTESIAN_POINT('Ctrl Pts',(79.1309222146226,72.0106634510243,203.423813267573));
#29608=CARTESIAN_POINT('Ctrl Pts',(76.9217750892174,71.8044827977391,203.359985324643));
#29609=CARTESIAN_POINT('Ctrl Pts',(75.8284320666291,71.9125028996057,203.330311434025));
#29610=CARTESIAN_POINT('Ctrl Pts',(73.7018082415606,72.5471160907228,203.270037764671));
#29611=CARTESIAN_POINT('Ctrl Pts',(72.6937001635906,73.0833811311108,203.237460863907));
#29612=CARTESIAN_POINT('Ctrl Pts',(70.9787202124067,74.492326251948,203.173593367182));
#29613=CARTESIAN_POINT('Ctrl Pts',(70.2779830201882,75.3388184047491,203.143810801366));
#29614=CARTESIAN_POINT('Ctrl Pts',(69.2921616440775,77.1437362025972,203.088046020435));
#29615=CARTESIAN_POINT('Ctrl Pts',(68.9767211862975,78.0660485396747,203.060383345032));
#29616=CARTESIAN_POINT('Ctrl Pts',(68.6698040180304,79.9778001095946,203.004579469033));
#29617=CARTESIAN_POINT('Ctrl Pts',(68.680844924591,80.9533421379321,202.976845194334));
#29618=CARTESIAN_POINT('Ctrl Pts',(68.8559951920603,81.9059493368125,202.950490121702));
#29619=CARTESIAN_POINT('Origin',(77.215862801455,80.3688697834411,196.));
#29620=CARTESIAN_POINT('',(79.2246973681942,88.6280818332357,205.75));
#29621=CARTESIAN_POINT('',(79.2246973681943,88.6280818332357,205.562499995903));
#29622=CARTESIAN_POINT('',(79.2246973681942,88.6280818332357,196.));
#29623=CARTESIAN_POINT('Ctrl Pts',(79.2246973681942,88.6280818332357,204.25));
#29624=CARTESIAN_POINT('Ctrl Pts',(79.0547950240752,88.6694060781853,204.254655943656));
#29625=CARTESIAN_POINT('Ctrl Pts',(78.8834444842995,88.7055298532413,204.259376138516));
#29626=CARTESIAN_POINT('Ctrl Pts',(77.6286107155098,88.9297303181128,204.294121525883));
#29627=CARTESIAN_POINT('Ctrl Pts',(76.519059945055,88.9112969084925,204.325802721434));
#29628=CARTESIAN_POINT('Ctrl Pts',(74.3493693210737,88.448816367255,204.389640835724));
#29629=CARTESIAN_POINT('Ctrl Pts',(73.3116823951001,88.0016672512237,204.420071743722));
#29630=CARTESIAN_POINT('Ctrl Pts',(71.4858223196629,86.7425777384377,204.480423978711));
#29631=CARTESIAN_POINT('Ctrl Pts',(70.7107049238398,85.949222473407,204.512067202917));
#29632=CARTESIAN_POINT('Ctrl Pts',(69.4936797724917,84.0935283363631,204.575944076656));
#29633=CARTESIAN_POINT('Ctrl Pts',(69.0705221214295,83.0444081245762,204.606516264026));
#29634=CARTESIAN_POINT('Ctrl Pts',(68.6595137231166,80.8641421504103,204.666791215114));
#29635=CARTESIAN_POINT('Ctrl Pts',(68.6671715184264,79.755537398259,204.698397796675));
#29636=CARTESIAN_POINT('Ctrl Pts',(69.1084701239968,77.5799369350521,204.762310511639));
#29637=CARTESIAN_POINT('Ctrl Pts',(69.5467986618995,76.5356865569769,204.79302029213));
#29638=CARTESIAN_POINT('Ctrl Pts',(70.7902410520497,74.6972968893464,204.85322160152));
#29639=CARTESIAN_POINT('Ctrl Pts',(71.5757281294194,73.9156436995867,204.884792934278));
#29640=CARTESIAN_POINT('Ctrl Pts',(73.4211507565819,72.6805157070973,204.948738754213));
#29641=CARTESIAN_POINT('Ctrl Pts',(74.4687521441418,72.2470550435054,204.979581987296));
#29642=CARTESIAN_POINT('Ctrl Pts',(76.6468976599112,71.8172241620404,205.039713277092));
#29643=CARTESIAN_POINT('Ctrl Pts',(77.75457057589,71.8152712787778,205.071250802282));
#29644=CARTESIAN_POINT('Ctrl Pts',(79.935352918856,72.2375993840587,205.135227169339));
#29645=CARTESIAN_POINT('Ctrl Pts',(80.985471132995,72.6680198729736,205.166199347506));
#29646=CARTESIAN_POINT('Ctrl Pts',(82.8349758522186,73.8974710690159,205.226264197649));
#29647=CARTESIAN_POINT('Ctrl Pts',(83.6223835547801,74.6759082239084,205.257769387555));
#29648=CARTESIAN_POINT('Ctrl Pts',(84.8735979709579,76.5120935576774,205.321773917147));
#29649=CARTESIAN_POINT('Ctrl Pts',(85.3162529196888,77.5583271120912,205.352870247422));
#29650=CARTESIAN_POINT('Ctrl Pts',(85.7628018663327,79.7345273984181,205.412872176407));
#29651=CARTESIAN_POINT('Ctrl Pts',(85.7732716972006,80.841304840974,205.44434651953));
#29652=CARTESIAN_POINT('Ctrl Pts',(85.3742595987554,82.9918949455739,205.507359870613));
#29653=CARTESIAN_POINT('Ctrl Pts',(84.9707173507996,84.0160228988743,205.537859900258));
#29654=CARTESIAN_POINT('Ctrl Pts',(83.7753048448417,85.8924753032416,205.597591168971));
#29655=CARTESIAN_POINT('Ctrl Pts',(82.9805478176727,86.7174735805474,205.630115476302));
#29656=CARTESIAN_POINT('Ctrl Pts',(81.1914960263918,87.953499975151,205.692765029491));
#29657=CARTESIAN_POINT('Ctrl Pts',(80.2346455730534,88.3824386832226,205.722323737133));
#29658=CARTESIAN_POINT('Ctrl Pts',(79.2246973681942,88.6280818332357,205.75));
#29659=CARTESIAN_POINT('Ctrl Pts',(79.2246973681943,88.6280818332357,205.562499995903));
#29660=CARTESIAN_POINT('Ctrl Pts',(79.5746236203243,88.5429715410128,205.552910740839));
#29661=CARTESIAN_POINT('Ctrl Pts',(79.9194864351651,88.4355396208418,205.543059605121));
#29662=CARTESIAN_POINT('Ctrl Pts',(81.3049358839305,87.90468798277,205.501795396723));
#29663=CARTESIAN_POINT('Ctrl Pts',(82.2629315361387,87.299679234003,205.469215109508));
#29664=CARTESIAN_POINT('Ctrl Pts',(83.8639035856507,85.7760330146877,205.406049115479));
#29665=CARTESIAN_POINT('Ctrl Pts',(84.5007511559166,84.8815467321273,205.377540967558));
#29666=CARTESIAN_POINT('Ctrl Pts',(85.4170056442561,82.869327389813,205.316180072339));
#29667=CARTESIAN_POINT('Ctrl Pts',(85.6752527768043,81.7651846868092,205.283591952461));
#29668=CARTESIAN_POINT('Ctrl Pts',(85.7465099051162,79.5555383723896,205.220346699203));
#29669=CARTESIAN_POINT('Ctrl Pts',(85.5725187913987,78.4715730813878,205.191752596847));
#29670=CARTESIAN_POINT('Ctrl Pts',(84.8130090264641,76.3944131651278,205.130505297389));
#29671=CARTESIAN_POINT('Ctrl Pts',(84.221574323948,75.4259072756991,205.097911367659));
#29672=CARTESIAN_POINT('Ctrl Pts',(82.7207727390167,73.8015912345431,205.034590827215));
#29673=CARTESIAN_POINT('Ctrl Pts',(81.8360768739623,73.1517524198025,205.005903411154));
#29674=CARTESIAN_POINT('Ctrl Pts',(79.8364829948426,72.2051002983537,204.944767604828));
#29675=CARTESIAN_POINT('Ctrl Pts',(78.7345582667739,71.9303700942887,204.912169730469));
#29676=CARTESIAN_POINT('Ctrl Pts',(76.5246780325853,71.8274817001122,204.848777877421));
#29677=CARTESIAN_POINT('Ctrl Pts',(75.4385197825051,71.9859065952006,204.819990974591));
#29678=CARTESIAN_POINT('Ctrl Pts',(73.3493287236972,72.7159957160027,204.758964195714));
#29679=CARTESIAN_POINT('Ctrl Pts',(72.3711691691772,73.2945898915279,204.726364075756));
#29680=CARTESIAN_POINT('Ctrl Pts',(70.7251666730187,74.7738812984265,204.662904854891));
#29681=CARTESIAN_POINT('Ctrl Pts',(70.063223191121,75.6494689288741,204.63401347033));
#29682=CARTESIAN_POINT('Ctrl Pts',(69.0883868988755,77.6371261520451,204.573092928327));
#29683=CARTESIAN_POINT('Ctrl Pts',(68.7983523247012,78.7367775367209,204.540492090979));
#29684=CARTESIAN_POINT('Ctrl Pts',(68.6660525183857,80.9466834842794,204.476969388502));
#29685=CARTESIAN_POINT('Ctrl Pts',(68.8100623931427,82.0348832452754,204.44796967565));
#29686=CARTESIAN_POINT('Ctrl Pts',(69.5128719382302,84.1350181467491,204.387152295575));
#29687=CARTESIAN_POINT('Ctrl Pts',(70.0794714028321,85.1219503069534,204.354552097251));
#29688=CARTESIAN_POINT('Ctrl Pts',(71.5387480542039,86.7878789204938,204.290969715752));
#29689=CARTESIAN_POINT('Ctrl Pts',(72.4059527581372,87.4609796926977,204.261858928146));
#29690=CARTESIAN_POINT('Ctrl Pts',(74.3824659498379,88.4616684098053,204.201141392504));
#29691=CARTESIAN_POINT('Ctrl Pts',(75.4798478652081,88.7657554928307,204.168543020111));
#29692=CARTESIAN_POINT('Ctrl Pts',(77.4851947546304,88.9103627885004,204.110791644394));
#29693=CARTESIAN_POINT('Ctrl Pts',(78.3691374440652,88.8361741232926,204.085945457012));
#29694=CARTESIAN_POINT('Ctrl Pts',(79.2246973681943,88.6280818332357,204.062499995903));
#29695=CARTESIAN_POINT('Origin',(77.215862801455,80.3688697834411,196.));
#29696=CARTESIAN_POINT('',(79.2246973785439,88.6280818307184,207.249999999433));
#29697=CARTESIAN_POINT('',(79.2246973681942,88.6280818332357,207.062499995903));
#29698=CARTESIAN_POINT('',(79.2246973681942,88.6280818332357,196.));
#29699=CARTESIAN_POINT('Ctrl Pts',(79.2246973681942,88.6280818332357,205.75));
#29700=CARTESIAN_POINT('Ctrl Pts',(79.1755458686982,88.6400366335967,205.751346930282));
#29701=CARTESIAN_POINT('Ctrl Pts',(79.1262688644913,88.6515572453659,205.752699355763));
#29702=CARTESIAN_POINT('Ctrl Pts',(77.9698628699743,88.9110389610774,205.784485466601));
#29703=CARTESIAN_POINT('Ctrl Pts',(76.8242753044325,88.9352980517108,205.817004105249));
#29704=CARTESIAN_POINT('Ctrl Pts',(74.6339424779926,88.5404260675109,205.88113100013));
#29705=CARTESIAN_POINT('Ctrl Pts',(73.6073941539547,88.1418598722174,205.911779931708));
#29706=CARTESIAN_POINT('Ctrl Pts',(71.7242201023183,86.9551933032193,205.971422048223));
#29707=CARTESIAN_POINT('Ctrl Pts',(70.8949618400678,86.1640289638711,206.003935228454));
#29708=CARTESIAN_POINT('Ctrl Pts',(69.620934520418,84.3385238803041,206.068079312029));
#29709=CARTESIAN_POINT('Ctrl Pts',(69.1745364768424,83.3316264994655,206.098796541174));
#29710=CARTESIAN_POINT('Ctrl Pts',(68.6771272706965,81.1615714590069,206.158398447979));
#29711=CARTESIAN_POINT('Ctrl Pts',(68.6477002044747,80.0155565132701,206.190906394971));
#29712=CARTESIAN_POINT('Ctrl Pts',(69.0330778830864,77.8225891951059,206.255066316178));
#29713=CARTESIAN_POINT('Ctrl Pts',(69.427334389355,76.7939435507699,206.285847856963));
#29714=CARTESIAN_POINT('Ctrl Pts',(70.6064211219714,74.9049697459813,206.345412270952));
#29715=CARTESIAN_POINT('Ctrl Pts',(71.3944614102049,74.0720398398838,206.377915219963));
#29716=CARTESIAN_POINT('Ctrl Pts',(73.2154483653594,72.7900438620707,206.442089728917));
#29717=CARTESIAN_POINT('Ctrl Pts',(74.2208922163273,72.339435211705,206.472931710179));
#29718=CARTESIAN_POINT('Ctrl Pts',(76.3897696237588,71.8332387536346,206.532461203267));
#29719=CARTESIAN_POINT('Ctrl Pts',(77.5361354964002,71.799347654986,206.564959395507));
#29720=CARTESIAN_POINT('Ctrl Pts',(79.7313610613022,72.1765215240137,206.629147336906));
#29721=CARTESIAN_POINT('Ctrl Pts',(80.7618173201636,72.5670590561585,206.660046018682));
#29722=CARTESIAN_POINT('Ctrl Pts',(82.6557795940566,73.7396013264785,206.719543019744));
#29723=CARTESIAN_POINT('Ctrl Pts',(83.4918644198226,74.5249366555228,206.752036698882));
#29724=CARTESIAN_POINT('Ctrl Pts',(84.7807228499175,76.3420153261727,206.816237005651));
#29725=CARTESIAN_POINT('Ctrl Pts',(85.2349594869248,77.3462073878713,206.847188791585));
#29726=CARTESIAN_POINT('Ctrl Pts',(85.7487184883279,79.5140581565082,206.906655589377));
#29727=CARTESIAN_POINT('Ctrl Pts',(85.7864527063175,80.6607126246621,206.939144998628));
#29728=CARTESIAN_POINT('Ctrl Pts',(85.4163437395074,82.8578694327888,207.003356685832));
#29729=CARTESIAN_POINT('Ctrl Pts',(85.029005309143,83.8898837484398,207.034358132052));
#29730=CARTESIAN_POINT('Ctrl Pts',(83.8620951489767,85.7881249973492,207.093796878944));
#29731=CARTESIAN_POINT('Ctrl Pts',(83.0790932824303,86.6269136567377,207.12628225868));
#29732=CARTESIAN_POINT('Ctrl Pts',(81.2722283004464,87.9167784342393,207.190262047185));
#29733=CARTESIAN_POINT('Ctrl Pts',(80.2777067148035,88.3719651996675,207.221143704834));
#29734=CARTESIAN_POINT('Ctrl Pts',(79.2246973785512,88.6280818307166,207.249999999716));
#29735=CARTESIAN_POINT('Ctrl Pts',(79.2246973681942,88.6280818332357,207.062499995903));
#29736=CARTESIAN_POINT('Ctrl Pts',(79.7626736033752,88.4972333635754,207.047757485714));
#29737=CARTESIAN_POINT('Ctrl Pts',(80.2878070141477,88.3138381978238,207.032419967914));
#29738=CARTESIAN_POINT('Ctrl Pts',(81.8034440810387,87.6108494868901,206.985198722085));
#29739=CARTESIAN_POINT('Ctrl Pts',(82.7124722494979,86.9475821107349,206.952766759942));
#29740=CARTESIAN_POINT('Ctrl Pts',(84.2077811049857,85.3243310536124,206.890364902975));
#29741=CARTESIAN_POINT('Ctrl Pts',(84.7861500033284,84.3856184999572,206.862154478088));
#29742=CARTESIAN_POINT('Ctrl Pts',(85.5639568106204,82.3191697074304,206.799861643146));
#29743=CARTESIAN_POINT('Ctrl Pts',(85.7475839193358,81.2079590741808,206.767402352516));
#29744=CARTESIAN_POINT('Ctrl Pts',(85.6759637513273,79.0019994762435,206.704894189922));
#29745=CARTESIAN_POINT('Ctrl Pts',(85.4306991084728,77.9279460999686,206.67669199462));
#29746=CARTESIAN_POINT('Ctrl Pts',(84.5372763828389,75.9086662499856,206.614513511158));
#29747=CARTESIAN_POINT('Ctrl Pts',(83.8887715100878,74.9866037317871,206.58202939494));
#29748=CARTESIAN_POINT('Ctrl Pts',(82.2910355884302,73.4636121941794,206.519417470665));
#29749=CARTESIAN_POINT('Ctrl Pts',(81.3639040595534,72.8699554007518,206.49120940288));
#29750=CARTESIAN_POINT('Ctrl Pts',(79.3111974045988,72.0557329190648,206.429146835329));
#29751=CARTESIAN_POINT('Ctrl Pts',(78.2013681697702,71.8525659891692,206.396640441623));
#29752=CARTESIAN_POINT('Ctrl Pts',(75.9940307549196,71.886794457265,206.333927617057));
#29753=CARTESIAN_POINT('Ctrl Pts',(74.9173768924445,72.1132389779678,206.305699924668));
#29754=CARTESIAN_POINT('Ctrl Pts',(72.882372475416,72.9714597388853,206.243754368681));
#29755=CARTESIAN_POINT('Ctrl Pts',(71.9477061598788,73.6051938323627,206.21122825658));
#29756=CARTESIAN_POINT('Ctrl Pts',(70.3976584377957,75.177600839623,206.148417673761));
#29757=CARTESIAN_POINT('Ctrl Pts',(69.7890434344216,76.0934119573733,206.120157136224));
#29758=CARTESIAN_POINT('Ctrl Pts',(68.9393305596217,78.1323667575335,206.058329206286));
#29759=CARTESIAN_POINT('Ctrl Pts',(68.7170550880179,79.2405233244568,206.025785912758));
#29760=CARTESIAN_POINT('Ctrl Pts',(68.7147121793083,81.4489260707761,205.962880954843));
#29761=CARTESIAN_POINT('Ctrl Pts',(68.922869605621,82.5281167816675,205.93457504872));
#29762=CARTESIAN_POINT('Ctrl Pts',(69.7467658319345,84.5780988313576,205.872864873705));
#29763=CARTESIAN_POINT('Ctrl Pts',(70.3659340359109,85.5247843303221,205.840306882449));
#29764=CARTESIAN_POINT('Ctrl Pts',(71.9135396100891,87.1009227330191,205.777311132512));
#29765=CARTESIAN_POINT('Ctrl Pts',(72.8184293434143,87.723986727704,205.748948176635));
#29766=CARTESIAN_POINT('Ctrl Pts',(74.8438249563057,88.6078323869357,205.687355403308));
#29767=CARTESIAN_POINT('Ctrl Pts',(75.9500663190504,88.8485384995735,205.65478511637));
#29768=CARTESIAN_POINT('Ctrl Pts',(77.7976988006892,88.8800156615273,205.602025887436));
#29769=CARTESIAN_POINT('Ctrl Pts',(78.5213987089167,88.7991406036099,205.581772943243));
#29770=CARTESIAN_POINT('Ctrl Pts',(79.2246973681943,88.6280818332357,205.562499995903));
#29771=CARTESIAN_POINT('Origin',(77.215862801455,80.368869783441,196.656249997952));
#29772=CARTESIAN_POINT('',(79.0328184976949,87.8391824855399,207.718749997952));
#29773=CARTESIAN_POINT('',(79.0328184976949,87.8391824855399,208.093749997952));
#29774=CARTESIAN_POINT('',(79.0328184976949,87.8391824855399,196.656249997952));
#29775=CARTESIAN_POINT('',(75.3989071052151,72.8985570813421,208.468749997952));
#29776=CARTESIAN_POINT('Ctrl Pts',(79.0328184976949,87.8391824855399,207.718749997952));
#29777=CARTESIAN_POINT('Ctrl Pts',(75.9385136613175,88.5917901771535,207.812499997952));
#29778=CARTESIAN_POINT('Ctrl Pts',(73.2183357261436,86.9359602466059,207.906249997952));
#29779=CARTESIAN_POINT('Ctrl Pts',(70.4981577909697,85.2801303160583,207.999999997952));
#29780=CARTESIAN_POINT('Ctrl Pts',(69.7455500993561,82.1858254796809,208.093749997952));
#29781=CARTESIAN_POINT('Ctrl Pts',(68.9929424077425,79.0915206433035,208.187499997952));
#29782=CARTESIAN_POINT('Ctrl Pts',(70.6487723382901,76.3713427081296,208.281249997952));
#29783=CARTESIAN_POINT('Ctrl Pts',(72.3046022688377,73.6511647729557,208.374999997952));
#29784=CARTESIAN_POINT('Ctrl Pts',(75.3989071052151,72.8985570813421,208.468749997952));
#29785=CARTESIAN_POINT('',(75.3989071052151,72.8985570813421,208.843749997952));
#29786=CARTESIAN_POINT('',(75.3989071052151,72.8985570813421,208.656249997952));
#29787=CARTESIAN_POINT('Ctrl Pts',(79.0328184976949,87.8391824855399,208.093749997952));
#29788=CARTESIAN_POINT('Ctrl Pts',(75.9385136613175,88.5917901771535,208.187499997952));
#29789=CARTESIAN_POINT('Ctrl Pts',(73.2183357261436,86.9359602466059,208.281249997952));
#29790=CARTESIAN_POINT('Ctrl Pts',(70.4981577909697,85.2801303160583,208.374999997952));
#29791=CARTESIAN_POINT('Ctrl Pts',(69.7455500993561,82.1858254796809,208.468749997952));
#29792=CARTESIAN_POINT('Ctrl Pts',(68.9929424077425,79.0915206433035,208.562499997952));
#29793=CARTESIAN_POINT('Ctrl Pts',(70.6487723382901,76.3713427081296,208.656249997952));
#29794=CARTESIAN_POINT('Ctrl Pts',(72.3046022688377,73.6511647729557,208.749999997952));
#29795=CARTESIAN_POINT('Ctrl Pts',(75.3989071052151,72.8985570813421,208.843749997952));
#29796=CARTESIAN_POINT('Origin',(77.215862801455,80.368869783441,196.656249997952));
#29797=CARTESIAN_POINT('',(79.0328184976949,87.8391824855399,206.218749997952));
#29798=CARTESIAN_POINT('',(79.0328184976949,87.8391824855399,206.593749997952));
#29799=CARTESIAN_POINT('',(79.0328184976949,87.8391824855399,196.656249997952));
#29800=CARTESIAN_POINT('Ctrl Pts',(79.0328184976949,87.8391824855399,206.218749997952));
#29801=CARTESIAN_POINT('Ctrl Pts',(75.9385136613175,88.5917901771535,206.312499997952));
#29802=CARTESIAN_POINT('Ctrl Pts',(73.2183357261436,86.9359602466059,206.406249997952));
#29803=CARTESIAN_POINT('Ctrl Pts',(70.4981577909697,85.2801303160583,206.499999997952));
#29804=CARTESIAN_POINT('Ctrl Pts',(69.7455500993561,82.1858254796809,206.593749997952));
#29805=CARTESIAN_POINT('Ctrl Pts',(68.9929424077425,79.0915206433035,206.687499997952));
#29806=CARTESIAN_POINT('Ctrl Pts',(70.6487723382901,76.3713427081296,206.781249997952));
#29807=CARTESIAN_POINT('Ctrl Pts',(72.3046022688378,73.6511647729557,206.874999997952));
#29808=CARTESIAN_POINT('Ctrl Pts',(75.3989071052151,72.8985570813421,206.968749997952));
#29809=CARTESIAN_POINT('Ctrl Pts',(78.4932119415925,72.1459493897285,207.062499997952));
#29810=CARTESIAN_POINT('Ctrl Pts',(81.2133898767664,73.8017793202761,207.156249997952));
#29811=CARTESIAN_POINT('Ctrl Pts',(83.9335678119403,75.4576092508238,207.249999997952));
#29812=CARTESIAN_POINT('Ctrl Pts',(84.6861755035539,78.5519140872011,207.343749997952));
#29813=CARTESIAN_POINT('Ctrl Pts',(85.4387831951675,81.6462189235785,207.437499997952));
#29814=CARTESIAN_POINT('Ctrl Pts',(83.7829532646199,84.3663968587524,207.531249997952));
#29815=CARTESIAN_POINT('Ctrl Pts',(82.1271233340723,87.0865747939263,207.624999997952));
#29816=CARTESIAN_POINT('Ctrl Pts',(79.0328184976949,87.8391824855399,207.718749997952));
#29817=CARTESIAN_POINT('Ctrl Pts',(79.0328184976949,87.8391824855399,206.593749997952));
#29818=CARTESIAN_POINT('Ctrl Pts',(75.9385136613175,88.5917901771535,206.687499997952));
#29819=CARTESIAN_POINT('Ctrl Pts',(73.2183357261436,86.9359602466059,206.781249997952));
#29820=CARTESIAN_POINT('Ctrl Pts',(70.4981577909697,85.2801303160583,206.874999997952));
#29821=CARTESIAN_POINT('Ctrl Pts',(69.7455500993561,82.1858254796809,206.968749997952));
#29822=CARTESIAN_POINT('Ctrl Pts',(68.9929424077425,79.0915206433035,207.062499997952));
#29823=CARTESIAN_POINT('Ctrl Pts',(70.6487723382901,76.3713427081296,207.156249997952));
#29824=CARTESIAN_POINT('Ctrl Pts',(72.3046022688378,73.6511647729557,207.249999997952));
#29825=CARTESIAN_POINT('Ctrl Pts',(75.3989071052151,72.8985570813421,207.343749997952));
#29826=CARTESIAN_POINT('Ctrl Pts',(78.4932119415925,72.1459493897285,207.437499997952));
#29827=CARTESIAN_POINT('Ctrl Pts',(81.2133898767664,73.8017793202761,207.531249997952));
#29828=CARTESIAN_POINT('Ctrl Pts',(83.9335678119403,75.4576092508238,207.624999997952));
#29829=CARTESIAN_POINT('Ctrl Pts',(84.6861755035539,78.5519140872011,207.718749997952));
#29830=CARTESIAN_POINT('Ctrl Pts',(85.4387831951675,81.6462189235785,207.812499997952));
#29831=CARTESIAN_POINT('Ctrl Pts',(83.7829532646199,84.3663968587524,207.906249997952));
#29832=CARTESIAN_POINT('Ctrl Pts',(82.1271233340723,87.0865747939263,207.999999997952));
#29833=CARTESIAN_POINT('Ctrl Pts',(79.0328184976949,87.8391824855399,208.093749997952));
#29834=CARTESIAN_POINT('Origin',(77.215862801455,80.368869783441,196.656249997952));
#29835=CARTESIAN_POINT('',(79.0328184976949,87.8391824855399,204.718749997952));
#29836=CARTESIAN_POINT('',(79.0328184976949,87.8391824855399,205.093749997952));
#29837=CARTESIAN_POINT('',(79.0328184976949,87.8391824855399,196.656249997952));
#29838=CARTESIAN_POINT('Ctrl Pts',(79.0328184976949,87.8391824855399,204.718749997952));
#29839=CARTESIAN_POINT('Ctrl Pts',(75.9385136613175,88.5917901771535,204.812499997952));
#29840=CARTESIAN_POINT('Ctrl Pts',(73.2183357261436,86.9359602466059,204.906249997952));
#29841=CARTESIAN_POINT('Ctrl Pts',(70.4981577909697,85.2801303160583,204.999999997952));
#29842=CARTESIAN_POINT('Ctrl Pts',(69.7455500993561,82.1858254796809,205.093749997952));
#29843=CARTESIAN_POINT('Ctrl Pts',(68.9929424077425,79.0915206433035,205.187499997952));
#29844=CARTESIAN_POINT('Ctrl Pts',(70.6487723382901,76.3713427081296,205.281249997952));
#29845=CARTESIAN_POINT('Ctrl Pts',(72.3046022688378,73.6511647729557,205.374999997952));
#29846=CARTESIAN_POINT('Ctrl Pts',(75.3989071052151,72.8985570813421,205.468749997952));
#29847=CARTESIAN_POINT('Ctrl Pts',(78.4932119415925,72.1459493897285,205.562499997952));
#29848=CARTESIAN_POINT('Ctrl Pts',(81.2133898767664,73.8017793202761,205.656249997952));
#29849=CARTESIAN_POINT('Ctrl Pts',(83.9335678119403,75.4576092508238,205.749999997952));
#29850=CARTESIAN_POINT('Ctrl Pts',(84.6861755035539,78.5519140872011,205.843749997952));
#29851=CARTESIAN_POINT('Ctrl Pts',(85.4387831951675,81.6462189235785,205.937499997952));
#29852=CARTESIAN_POINT('Ctrl Pts',(83.7829532646199,84.3663968587524,206.031249997952));
#29853=CARTESIAN_POINT('Ctrl Pts',(82.1271233340723,87.0865747939263,206.124999997952));
#29854=CARTESIAN_POINT('Ctrl Pts',(79.0328184976949,87.8391824855399,206.218749997952));
#29855=CARTESIAN_POINT('Ctrl Pts',(79.0328184976949,87.8391824855399,205.093749997952));
#29856=CARTESIAN_POINT('Ctrl Pts',(75.9385136613175,88.5917901771535,205.187499997952));
#29857=CARTESIAN_POINT('Ctrl Pts',(73.2183357261436,86.9359602466059,205.281249997952));
#29858=CARTESIAN_POINT('Ctrl Pts',(70.4981577909697,85.2801303160583,205.374999997952));
#29859=CARTESIAN_POINT('Ctrl Pts',(69.7455500993561,82.1858254796809,205.468749997952));
#29860=CARTESIAN_POINT('Ctrl Pts',(68.9929424077425,79.0915206433035,205.562499997952));
#29861=CARTESIAN_POINT('Ctrl Pts',(70.6487723382901,76.3713427081296,205.656249997952));
#29862=CARTESIAN_POINT('Ctrl Pts',(72.3046022688378,73.6511647729557,205.749999997952));
#29863=CARTESIAN_POINT('Ctrl Pts',(75.3989071052151,72.8985570813421,205.843749997952));
#29864=CARTESIAN_POINT('Ctrl Pts',(78.4932119415925,72.1459493897285,205.937499997952));
#29865=CARTESIAN_POINT('Ctrl Pts',(81.2133898767664,73.8017793202761,206.031249997952));
#29866=CARTESIAN_POINT('Ctrl Pts',(83.9335678119403,75.4576092508238,206.124999997952));
#29867=CARTESIAN_POINT('Ctrl Pts',(84.6861755035539,78.5519140872011,206.218749997952));
#29868=CARTESIAN_POINT('Ctrl Pts',(85.4387831951675,81.6462189235785,206.312499997952));
#29869=CARTESIAN_POINT('Ctrl Pts',(83.7829532646199,84.3663968587524,206.406249997952));
#29870=CARTESIAN_POINT('Ctrl Pts',(82.1271233340723,87.0865747939263,206.499999997952));
#29871=CARTESIAN_POINT('Ctrl Pts',(79.0328184976949,87.8391824855399,206.593749997952));
#29872=CARTESIAN_POINT('Origin',(77.215862801455,80.368869783441,196.656249997952));
#29873=CARTESIAN_POINT('',(79.0328184976949,87.8391824855399,203.218749997952));
#29874=CARTESIAN_POINT('',(79.0328184976949,87.8391824855399,203.593749997952));
#29875=CARTESIAN_POINT('',(79.0328184976949,87.8391824855399,196.656249997952));
#29876=CARTESIAN_POINT('Ctrl Pts',(79.0328184976949,87.8391824855399,203.218749997952));
#29877=CARTESIAN_POINT('Ctrl Pts',(75.9385136613175,88.5917901771535,203.312499997952));
#29878=CARTESIAN_POINT('Ctrl Pts',(73.2183357261436,86.9359602466059,203.406249997952));
#29879=CARTESIAN_POINT('Ctrl Pts',(70.4981577909697,85.2801303160583,203.499999997952));
#29880=CARTESIAN_POINT('Ctrl Pts',(69.7455500993561,82.1858254796809,203.593749997952));
#29881=CARTESIAN_POINT('Ctrl Pts',(68.9929424077425,79.0915206433035,203.687499997952));
#29882=CARTESIAN_POINT('Ctrl Pts',(70.6487723382901,76.3713427081296,203.781249997952));
#29883=CARTESIAN_POINT('Ctrl Pts',(72.3046022688378,73.6511647729557,203.874999997952));
#29884=CARTESIAN_POINT('Ctrl Pts',(75.3989071052151,72.8985570813421,203.968749997952));
#29885=CARTESIAN_POINT('Ctrl Pts',(78.4932119415925,72.1459493897285,204.062499997952));
#29886=CARTESIAN_POINT('Ctrl Pts',(81.2133898767664,73.8017793202761,204.156249997952));
#29887=CARTESIAN_POINT('Ctrl Pts',(83.9335678119403,75.4576092508238,204.249999997952));
#29888=CARTESIAN_POINT('Ctrl Pts',(84.6861755035539,78.5519140872011,204.343749997952));
#29889=CARTESIAN_POINT('Ctrl Pts',(85.4387831951675,81.6462189235785,204.437499997952));
#29890=CARTESIAN_POINT('Ctrl Pts',(83.7829532646199,84.3663968587524,204.531249997952));
#29891=CARTESIAN_POINT('Ctrl Pts',(82.1271233340723,87.0865747939263,204.624999997952));
#29892=CARTESIAN_POINT('Ctrl Pts',(79.0328184976949,87.8391824855399,204.718749997952));
#29893=CARTESIAN_POINT('Ctrl Pts',(79.0328184976949,87.8391824855399,203.593749997952));
#29894=CARTESIAN_POINT('Ctrl Pts',(75.9385136613175,88.5917901771535,203.687499997952));
#29895=CARTESIAN_POINT('Ctrl Pts',(73.2183357261436,86.9359602466059,203.781249997952));
#29896=CARTESIAN_POINT('Ctrl Pts',(70.4981577909697,85.2801303160583,203.874999997952));
#29897=CARTESIAN_POINT('Ctrl Pts',(69.7455500993561,82.1858254796809,203.968749997952));
#29898=CARTESIAN_POINT('Ctrl Pts',(68.9929424077425,79.0915206433035,204.062499997952));
#29899=CARTESIAN_POINT('Ctrl Pts',(70.6487723382901,76.3713427081296,204.156249997952));
#29900=CARTESIAN_POINT('Ctrl Pts',(72.3046022688378,73.6511647729557,204.249999997952));
#29901=CARTESIAN_POINT('Ctrl Pts',(75.3989071052151,72.8985570813421,204.343749997952));
#29902=CARTESIAN_POINT('Ctrl Pts',(78.4932119415925,72.1459493897285,204.437499997952));
#29903=CARTESIAN_POINT('Ctrl Pts',(81.2133898767664,73.8017793202761,204.531249997952));
#29904=CARTESIAN_POINT('Ctrl Pts',(83.9335678119403,75.4576092508238,204.624999997952));
#29905=CARTESIAN_POINT('Ctrl Pts',(84.6861755035539,78.5519140872011,204.718749997952));
#29906=CARTESIAN_POINT('Ctrl Pts',(85.4387831951675,81.6462189235785,204.812499997952));
#29907=CARTESIAN_POINT('Ctrl Pts',(83.7829532646199,84.3663968587524,204.906249997952));
#29908=CARTESIAN_POINT('Ctrl Pts',(82.1271233340723,87.0865747939263,204.999999997952));
#29909=CARTESIAN_POINT('Ctrl Pts',(79.0328184976949,87.8391824855399,205.093749997952));
#29910=CARTESIAN_POINT('Origin',(77.215862801455,80.368869783441,196.656249997952));
#29911=CARTESIAN_POINT('',(79.0328184976949,87.8391824855399,201.718749997952));
#29912=CARTESIAN_POINT('',(79.0328184976949,87.8391824855399,202.093749997952));
#29913=CARTESIAN_POINT('',(79.0328184976949,87.8391824855399,196.656249997952));
#29914=CARTESIAN_POINT('Ctrl Pts',(79.0328184976949,87.8391824855399,201.718749997952));
#29915=CARTESIAN_POINT('Ctrl Pts',(75.9385136613175,88.5917901771536,201.812499997952));
#29916=CARTESIAN_POINT('Ctrl Pts',(73.2183357261436,86.9359602466059,201.906249997952));
#29917=CARTESIAN_POINT('Ctrl Pts',(70.4981577909697,85.2801303160583,201.999999997952));
#29918=CARTESIAN_POINT('Ctrl Pts',(69.7455500993561,82.1858254796809,202.093749997952));
#29919=CARTESIAN_POINT('Ctrl Pts',(68.9929424077425,79.0915206433035,202.187499997952));
#29920=CARTESIAN_POINT('Ctrl Pts',(70.6487723382901,76.3713427081296,202.281249997952));
#29921=CARTESIAN_POINT('Ctrl Pts',(72.3046022688378,73.6511647729557,202.374999997952));
#29922=CARTESIAN_POINT('Ctrl Pts',(75.3989071052151,72.8985570813421,202.468749997952));
#29923=CARTESIAN_POINT('Ctrl Pts',(78.4932119415925,72.1459493897285,202.562499997952));
#29924=CARTESIAN_POINT('Ctrl Pts',(81.2133898767664,73.8017793202761,202.656249997952));
#29925=CARTESIAN_POINT('Ctrl Pts',(83.9335678119403,75.4576092508238,202.749999997952));
#29926=CARTESIAN_POINT('Ctrl Pts',(84.6861755035539,78.5519140872011,202.843749997952));
#29927=CARTESIAN_POINT('Ctrl Pts',(85.4387831951675,81.6462189235785,202.937499997952));
#29928=CARTESIAN_POINT('Ctrl Pts',(83.7829532646199,84.3663968587524,203.031249997952));
#29929=CARTESIAN_POINT('Ctrl Pts',(82.1271233340723,87.0865747939263,203.124999997952));
#29930=CARTESIAN_POINT('Ctrl Pts',(79.0328184976949,87.8391824855399,203.218749997952));
#29931=CARTESIAN_POINT('Ctrl Pts',(79.0328184976949,87.8391824855399,202.093749997952));
#29932=CARTESIAN_POINT('Ctrl Pts',(75.9385136613175,88.5917901771535,202.187499997952));
#29933=CARTESIAN_POINT('Ctrl Pts',(73.2183357261436,86.9359602466059,202.281249997952));
#29934=CARTESIAN_POINT('Ctrl Pts',(70.4981577909697,85.2801303160583,202.374999997952));
#29935=CARTESIAN_POINT('Ctrl Pts',(69.7455500993561,82.1858254796809,202.468749997952));
#29936=CARTESIAN_POINT('Ctrl Pts',(68.9929424077425,79.0915206433035,202.562499997952));
#29937=CARTESIAN_POINT('Ctrl Pts',(70.6487723382901,76.3713427081296,202.656249997952));
#29938=CARTESIAN_POINT('Ctrl Pts',(72.3046022688378,73.6511647729557,202.749999997952));
#29939=CARTESIAN_POINT('Ctrl Pts',(75.3989071052151,72.8985570813421,202.843749997952));
#29940=CARTESIAN_POINT('Ctrl Pts',(78.4932119415925,72.1459493897285,202.937499997952));
#29941=CARTESIAN_POINT('Ctrl Pts',(81.2133898767664,73.8017793202761,203.031249997952));
#29942=CARTESIAN_POINT('Ctrl Pts',(83.9335678119403,75.4576092508238,203.124999997952));
#29943=CARTESIAN_POINT('Ctrl Pts',(84.6861755035539,78.5519140872011,203.218749997952));
#29944=CARTESIAN_POINT('Ctrl Pts',(85.4387831951675,81.6462189235785,203.312499997952));
#29945=CARTESIAN_POINT('Ctrl Pts',(83.7829532646199,84.3663968587524,203.406249997952));
#29946=CARTESIAN_POINT('Ctrl Pts',(82.1271233340723,87.0865747939263,203.499999997952));
#29947=CARTESIAN_POINT('Ctrl Pts',(79.0328184976949,87.8391824855399,203.593749997952));
#29948=CARTESIAN_POINT('Origin',(77.215862801455,80.368869783441,196.656249997952));
#29949=CARTESIAN_POINT('',(79.0328184976949,87.8391824855399,200.218749997952));
#29950=CARTESIAN_POINT('',(79.0328184976949,87.8391824855399,200.593749997952));
#29951=CARTESIAN_POINT('',(79.0328184976949,87.8391824855399,196.656249997952));
#29952=CARTESIAN_POINT('Ctrl Pts',(79.0328184976949,87.8391824855399,200.218749997952));
#29953=CARTESIAN_POINT('Ctrl Pts',(75.9385136613175,88.5917901771536,200.312499997952));
#29954=CARTESIAN_POINT('Ctrl Pts',(73.2183357261436,86.9359602466059,200.406249997952));
#29955=CARTESIAN_POINT('Ctrl Pts',(70.4981577909697,85.2801303160583,200.499999997952));
#29956=CARTESIAN_POINT('Ctrl Pts',(69.7455500993561,82.1858254796809,200.593749997952));
#29957=CARTESIAN_POINT('Ctrl Pts',(68.9929424077425,79.0915206433036,200.687499997952));
#29958=CARTESIAN_POINT('Ctrl Pts',(70.6487723382901,76.3713427081296,200.781249997952));
#29959=CARTESIAN_POINT('Ctrl Pts',(72.3046022688378,73.6511647729557,200.874999997952));
#29960=CARTESIAN_POINT('Ctrl Pts',(75.3989071052151,72.8985570813421,200.968749997952));
#29961=CARTESIAN_POINT('Ctrl Pts',(78.4932119415925,72.1459493897285,201.062499997952));
#29962=CARTESIAN_POINT('Ctrl Pts',(81.2133898767664,73.8017793202761,201.156249997952));
#29963=CARTESIAN_POINT('Ctrl Pts',(83.9335678119403,75.4576092508238,201.249999997952));
#29964=CARTESIAN_POINT('Ctrl Pts',(84.6861755035539,78.5519140872011,201.343749997952));
#29965=CARTESIAN_POINT('Ctrl Pts',(85.4387831951675,81.6462189235785,201.437499997952));
#29966=CARTESIAN_POINT('Ctrl Pts',(83.7829532646199,84.3663968587524,201.531249997952));
#29967=CARTESIAN_POINT('Ctrl Pts',(82.1271233340723,87.0865747939263,201.624999997952));
#29968=CARTESIAN_POINT('Ctrl Pts',(79.0328184976949,87.8391824855399,201.718749997952));
#29969=CARTESIAN_POINT('Ctrl Pts',(79.0328184976949,87.8391824855399,200.593749997952));
#29970=CARTESIAN_POINT('Ctrl Pts',(75.9385136613175,88.5917901771536,200.687499997952));
#29971=CARTESIAN_POINT('Ctrl Pts',(73.2183357261436,86.9359602466059,200.781249997952));
#29972=CARTESIAN_POINT('Ctrl Pts',(70.4981577909697,85.2801303160583,200.874999997952));
#29973=CARTESIAN_POINT('Ctrl Pts',(69.7455500993561,82.1858254796809,200.968749997952));
#29974=CARTESIAN_POINT('Ctrl Pts',(68.9929424077425,79.0915206433036,201.062499997952));
#29975=CARTESIAN_POINT('Ctrl Pts',(70.6487723382901,76.3713427081296,201.156249997952));
#29976=CARTESIAN_POINT('Ctrl Pts',(72.3046022688378,73.6511647729557,201.249999997952));
#29977=CARTESIAN_POINT('Ctrl Pts',(75.3989071052151,72.8985570813421,201.343749997952));
#29978=CARTESIAN_POINT('Ctrl Pts',(78.4932119415925,72.1459493897285,201.437499997952));
#29979=CARTESIAN_POINT('Ctrl Pts',(81.2133898767664,73.8017793202761,201.531249997952));
#29980=CARTESIAN_POINT('Ctrl Pts',(83.9335678119403,75.4576092508238,201.624999997952));
#29981=CARTESIAN_POINT('Ctrl Pts',(84.6861755035539,78.5519140872011,201.718749997952));
#29982=CARTESIAN_POINT('Ctrl Pts',(85.4387831951675,81.6462189235785,201.812499997952));
#29983=CARTESIAN_POINT('Ctrl Pts',(83.7829532646199,84.3663968587524,201.906249997952));
#29984=CARTESIAN_POINT('Ctrl Pts',(82.1271233340723,87.0865747939263,201.999999997952));
#29985=CARTESIAN_POINT('Ctrl Pts',(79.0328184976949,87.8391824855399,202.093749997952));
#29986=CARTESIAN_POINT('Origin',(77.215862801455,80.368869783441,196.656249997952));
#29987=CARTESIAN_POINT('',(79.0328184976949,87.8391824855399,198.718749997952));
#29988=CARTESIAN_POINT('',(79.0328184976949,87.8391824855399,199.093749997952));
#29989=CARTESIAN_POINT('',(79.0328184976949,87.8391824855399,196.656249997952));
#29990=CARTESIAN_POINT('Ctrl Pts',(79.0328184976949,87.8391824855399,198.718749997952));
#29991=CARTESIAN_POINT('Ctrl Pts',(75.9385136613175,88.5917901771536,198.812499997952));
#29992=CARTESIAN_POINT('Ctrl Pts',(73.2183357261436,86.9359602466059,198.906249997952));
#29993=CARTESIAN_POINT('Ctrl Pts',(70.4981577909697,85.2801303160583,198.999999997952));
#29994=CARTESIAN_POINT('Ctrl Pts',(69.7455500993561,82.1858254796809,199.093749997952));
#29995=CARTESIAN_POINT('Ctrl Pts',(68.9929424077425,79.0915206433036,199.187499997952));
#29996=CARTESIAN_POINT('Ctrl Pts',(70.6487723382901,76.3713427081296,199.281249997952));
#29997=CARTESIAN_POINT('Ctrl Pts',(72.3046022688378,73.6511647729557,199.374999997952));
#29998=CARTESIAN_POINT('Ctrl Pts',(75.3989071052151,72.8985570813421,199.468749997952));
#29999=CARTESIAN_POINT('Ctrl Pts',(78.4932119415925,72.1459493897285,199.562499997952));
#30000=CARTESIAN_POINT('Ctrl Pts',(81.2133898767664,73.8017793202761,199.656249997952));
#30001=CARTESIAN_POINT('Ctrl Pts',(83.9335678119403,75.4576092508238,199.749999997952));
#30002=CARTESIAN_POINT('Ctrl Pts',(84.6861755035539,78.5519140872012,199.843749997952));
#30003=CARTESIAN_POINT('Ctrl Pts',(85.4387831951675,81.6462189235785,199.937499997952));
#30004=CARTESIAN_POINT('Ctrl Pts',(83.7829532646199,84.3663968587524,200.031249997952));
#30005=CARTESIAN_POINT('Ctrl Pts',(82.1271233340723,87.0865747939263,200.124999997952));
#30006=CARTESIAN_POINT('Ctrl Pts',(79.0328184976949,87.8391824855399,200.218749997952));
#30007=CARTESIAN_POINT('Ctrl Pts',(79.0328184976949,87.8391824855399,199.093749997952));
#30008=CARTESIAN_POINT('Ctrl Pts',(75.9385136613175,88.5917901771536,199.187499997952));
#30009=CARTESIAN_POINT('Ctrl Pts',(73.2183357261436,86.9359602466059,199.281249997952));
#30010=CARTESIAN_POINT('Ctrl Pts',(70.4981577909697,85.2801303160583,199.374999997952));
#30011=CARTESIAN_POINT('Ctrl Pts',(69.7455500993561,82.1858254796809,199.468749997952));
#30012=CARTESIAN_POINT('Ctrl Pts',(68.9929424077425,79.0915206433036,199.562499997952));
#30013=CARTESIAN_POINT('Ctrl Pts',(70.6487723382901,76.3713427081296,199.656249997952));
#30014=CARTESIAN_POINT('Ctrl Pts',(72.3046022688378,73.6511647729557,199.749999997952));
#30015=CARTESIAN_POINT('Ctrl Pts',(75.3989071052151,72.8985570813421,199.843749997952));
#30016=CARTESIAN_POINT('Ctrl Pts',(78.4932119415925,72.1459493897285,199.937499997952));
#30017=CARTESIAN_POINT('Ctrl Pts',(81.2133898767664,73.8017793202761,200.031249997952));
#30018=CARTESIAN_POINT('Ctrl Pts',(83.9335678119403,75.4576092508238,200.124999997952));
#30019=CARTESIAN_POINT('Ctrl Pts',(84.6861755035539,78.5519140872012,200.218749997952));
#30020=CARTESIAN_POINT('Ctrl Pts',(85.4387831951675,81.6462189235785,200.312499997952));
#30021=CARTESIAN_POINT('Ctrl Pts',(83.7829532646199,84.3663968587524,200.406249997952));
#30022=CARTESIAN_POINT('Ctrl Pts',(82.1271233340723,87.0865747939263,200.499999997952));
#30023=CARTESIAN_POINT('Ctrl Pts',(79.0328184976949,87.8391824855399,200.593749997952));
#30024=CARTESIAN_POINT('Origin',(77.215862801455,80.368869783441,196.656249997952));
#30025=CARTESIAN_POINT('',(79.0328184976949,87.83918248554,197.218749997952));
#30026=CARTESIAN_POINT('',(79.0328184976949,87.83918248554,197.593749997952));
#30027=CARTESIAN_POINT('',(79.0328184976949,87.8391824855399,196.656249997952));
#30028=CARTESIAN_POINT('Ctrl Pts',(79.0328184976949,87.83918248554,197.218749997952));
#30029=CARTESIAN_POINT('Ctrl Pts',(75.9385136613175,88.5917901771536,197.312499997952));
#30030=CARTESIAN_POINT('Ctrl Pts',(73.2183357261436,86.9359602466059,197.406249997952));
#30031=CARTESIAN_POINT('Ctrl Pts',(70.4981577909697,85.2801303160583,197.499999997952));
#30032=CARTESIAN_POINT('Ctrl Pts',(69.7455500993561,82.1858254796809,197.593749997952));
#30033=CARTESIAN_POINT('Ctrl Pts',(68.9929424077425,79.0915206433036,197.687499997952));
#30034=CARTESIAN_POINT('Ctrl Pts',(70.6487723382901,76.3713427081296,197.781249997952));
#30035=CARTESIAN_POINT('Ctrl Pts',(72.3046022688378,73.6511647729557,197.874999997952));
#30036=CARTESIAN_POINT('Ctrl Pts',(75.3989071052151,72.8985570813421,197.968749997952));
#30037=CARTESIAN_POINT('Ctrl Pts',(78.4932119415925,72.1459493897285,198.062499997952));
#30038=CARTESIAN_POINT('Ctrl Pts',(81.2133898767664,73.8017793202762,198.156249997952));
#30039=CARTESIAN_POINT('Ctrl Pts',(83.9335678119403,75.4576092508238,198.249999997952));
#30040=CARTESIAN_POINT('Ctrl Pts',(84.6861755035539,78.5519140872012,198.343749997952));
#30041=CARTESIAN_POINT('Ctrl Pts',(85.4387831951675,81.6462189235785,198.437499997952));
#30042=CARTESIAN_POINT('Ctrl Pts',(83.7829532646199,84.3663968587524,198.531249997952));
#30043=CARTESIAN_POINT('Ctrl Pts',(82.1271233340723,87.0865747939263,198.624999997952));
#30044=CARTESIAN_POINT('Ctrl Pts',(79.0328184976949,87.8391824855399,198.718749997952));
#30045=CARTESIAN_POINT('Ctrl Pts',(79.0328184976949,87.83918248554,197.593749997952));
#30046=CARTESIAN_POINT('Ctrl Pts',(75.9385136613175,88.5917901771536,197.687499997952));
#30047=CARTESIAN_POINT('Ctrl Pts',(73.2183357261436,86.9359602466059,197.781249997952));
#30048=CARTESIAN_POINT('Ctrl Pts',(70.4981577909697,85.2801303160583,197.874999997952));
#30049=CARTESIAN_POINT('Ctrl Pts',(69.7455500993561,82.1858254796809,197.968749997952));
#30050=CARTESIAN_POINT('Ctrl Pts',(68.9929424077425,79.0915206433036,198.062499997952));
#30051=CARTESIAN_POINT('Ctrl Pts',(70.6487723382901,76.3713427081296,198.156249997952));
#30052=CARTESIAN_POINT('Ctrl Pts',(72.3046022688378,73.6511647729557,198.249999997952));
#30053=CARTESIAN_POINT('Ctrl Pts',(75.3989071052151,72.8985570813421,198.343749997952));
#30054=CARTESIAN_POINT('Ctrl Pts',(78.4932119415925,72.1459493897285,198.437499997952));
#30055=CARTESIAN_POINT('Ctrl Pts',(81.2133898767664,73.8017793202762,198.531249997952));
#30056=CARTESIAN_POINT('Ctrl Pts',(83.9335678119403,75.4576092508238,198.624999997952));
#30057=CARTESIAN_POINT('Ctrl Pts',(84.6861755035539,78.5519140872012,198.718749997952));
#30058=CARTESIAN_POINT('Ctrl Pts',(85.4387831951675,81.6462189235785,198.812499997952));
#30059=CARTESIAN_POINT('Ctrl Pts',(83.7829532646199,84.3663968587524,198.906249997952));
#30060=CARTESIAN_POINT('Ctrl Pts',(82.1271233340723,87.0865747939263,198.999999997952));
#30061=CARTESIAN_POINT('Ctrl Pts',(79.0328184976949,87.8391824855399,199.093749997952));
#30062=CARTESIAN_POINT('Origin',(77.215862801455,80.368869783441,202.950490121702));
#30063=CARTESIAN_POINT('',(70.3188266909529,84.6163270098801,201.781598171062));
#30064=CARTESIAN_POINT('',(70.3188266908911,84.6163270097798,202.632217951621));
#30065=CARTESIAN_POINT('',(70.3188266908911,84.6163270097798,202.950490121702));
#30066=CARTESIAN_POINT('',(71.4950332612281,74.6345773796942,202.950490121702));
#30067=CARTESIAN_POINT('Ctrl Pts',(70.3188266908911,84.6163270097798,202.632217951621));
#30068=CARTESIAN_POINT('Ctrl Pts',(69.8260630992339,83.8161757417328,202.660549743681));
#30069=CARTESIAN_POINT('Ctrl Pts',(69.4758927081056,82.9356925528463,202.687664763062));
#30070=CARTESIAN_POINT('Ctrl Pts',(69.0654723363739,80.9572904623708,202.744886064915));
#30071=CARTESIAN_POINT('Ctrl Pts',(69.0596817908794,79.8671815276535,202.777438263858));
#30072=CARTESIAN_POINT('Ctrl Pts',(69.4230173888357,78.0169388556641,202.834421549943));
#30073=CARTESIAN_POINT('Ctrl Pts',(69.6956273873066,77.2534017968305,202.858506272242));
#30074=CARTESIAN_POINT('Ctrl Pts',(70.452887584812,75.8403870443048,202.904251327559));
#30075=CARTESIAN_POINT('Ctrl Pts',(70.9308791578428,75.1974069727192,202.926669622759));
#30076=CARTESIAN_POINT('Ctrl Pts',(71.4950332612281,74.6345773796942,202.950490121702));
#30077=CARTESIAN_POINT('',(80.1444697952855,87.9209066660103,202.950490121702));
#30078=CARTESIAN_POINT('Origin',(77.215862801455,80.368869783441,202.950490121702));
#30079=CARTESIAN_POINT('Ctrl Pts',(80.1444697952855,87.9209066660103,202.950490121702));
#30080=CARTESIAN_POINT('Ctrl Pts',(80.7200382197996,87.6977067876635,202.932453294557));
#30081=CARTESIAN_POINT('Ctrl Pts',(81.2681907870714,87.4094459354855,202.913924504458));
#30082=CARTESIAN_POINT('Ctrl Pts',(82.2902634071623,86.7127185595319,202.876533681128));
#30083=CARTESIAN_POINT('Ctrl Pts',(82.7605307726769,86.3060937699065,202.857793704478));
#30084=CARTESIAN_POINT('Ctrl Pts',(83.884971986828,85.0825658474528,202.80850017344));
#30085=CARTESIAN_POINT('Ctrl Pts',(84.4354526815245,84.1863912748104,202.780263866786));
#30086=CARTESIAN_POINT('Ctrl Pts',(85.1733087176293,82.216853288982,202.717976598169));
#30087=CARTESIAN_POINT('Ctrl Pts',(85.3467097290497,81.1596354998922,202.685575488723));
#30088=CARTESIAN_POINT('Ctrl Pts',(85.2766300294487,79.0566091684042,202.623049623368));
#30089=CARTESIAN_POINT('Ctrl Pts',(85.0408547860707,78.0306016065895,202.594775699681));
#30090=CARTESIAN_POINT('Ctrl Pts',(84.1862092473497,76.1087855526369,202.532598460018));
#30091=CARTESIAN_POINT('Ctrl Pts',(83.5693696737583,75.2339905450627,202.500229467398));
#30092=CARTESIAN_POINT('Ctrl Pts',(82.0454202384975,73.782856088795,202.437597096895));
#30093=CARTESIAN_POINT('Ctrl Pts',(81.1571548977831,73.2157991039416,202.409271700632));
#30094=CARTESIAN_POINT('Ctrl Pts',(79.2002098388061,72.4445722857407,202.347205861164));
#30095=CARTESIAN_POINT('Ctrl Pts',(78.1479962948602,72.2532532406794,202.314871124405));
#30096=CARTESIAN_POINT('Ctrl Pts',(76.0437079241934,72.2862584322486,202.252135423023));
#30097=CARTESIAN_POINT('Ctrl Pts',(75.0115965537525,72.5047890330912,202.223745140531));
#30098=CARTESIAN_POINT('Ctrl Pts',(73.0753240127736,73.3271254291722,202.161791655021));
#30099=CARTESIAN_POINT('Ctrl Pts',(72.1916127489154,73.9278208919559,202.129493139258));
#30100=CARTESIAN_POINT('Ctrl Pts',(70.7136942080754,75.426517773662,202.066657580305));
#30101=CARTESIAN_POINT('Ctrl Pts',(70.1302477279942,76.3069612374748,202.038189616412));
#30102=CARTESIAN_POINT('Ctrl Pts',(69.3263609564473,78.2512964686591,201.976349011223));
#30103=CARTESIAN_POINT('Ctrl Pts',(69.1175769021875,79.2983139470911,201.944088483078));
#30104=CARTESIAN_POINT('Ctrl Pts',(69.1141855440971,81.4035063400024,201.881156792816));
#30105=CARTESIAN_POINT('Ctrl Pts',(69.3157744439333,82.4416101002022,201.852599130526));
#30106=CARTESIAN_POINT('Ctrl Pts',(69.8791381422001,83.8310072859288,201.808620460806));
#30107=CARTESIAN_POINT('Ctrl Pts',(70.0831214561213,84.2335880134999,201.795150210652));
#30108=CARTESIAN_POINT('Ctrl Pts',(70.3188266910146,84.6163270099804,201.781598171062));
#30109=CARTESIAN_POINT('Origin',(77.215862801455,80.368869783441,202.950490121702));
#30110=CARTESIAN_POINT('',(70.3188266909498,84.6163270098751,200.281598171063));
#30111=CARTESIAN_POINT('',(70.3188266908911,84.6163270097798,201.132217951621));
#30112=CARTESIAN_POINT('',(70.3188266908911,84.6163270097798,202.950490121702));
#30113=CARTESIAN_POINT('Ctrl Pts',(70.3188266908911,84.6163270097798,201.132217951621));
#30114=CARTESIAN_POINT('Ctrl Pts',(70.3172417146298,84.6137533197046,201.132309080955));
#30115=CARTESIAN_POINT('Ctrl Pts',(70.3156581350604,84.6111786711708,201.132400208759));
#30116=CARTESIAN_POINT('Ctrl Pts',(69.7713840908533,83.7251645777047,201.163747832253));
#30117=CARTESIAN_POINT('Ctrl Pts',(69.4033391753829,82.7457136988302,201.193005655864));
#30118=CARTESIAN_POINT('Ctrl Pts',(69.0500898072157,80.6632671197291,201.253601856235));
#30119=CARTESIAN_POINT('Ctrl Pts',(69.0831793119235,79.5777427661445,201.28619754089));
#30120=CARTESIAN_POINT('Ctrl Pts',(69.5626100780708,77.5205335311856,201.34990521851));
#30121=CARTESIAN_POINT('Ctrl Pts',(69.9897154545897,76.5651853971245,201.379276027556));
#30122=CARTESIAN_POINT('Ctrl Pts',(71.203353071391,74.8355585884899,201.439781139428));
#30123=CARTESIAN_POINT('Ctrl Pts',(71.9907437379569,74.086685699147,201.472372902096));
#30124=CARTESIAN_POINT('Ctrl Pts',(73.7791390912364,72.9611310339534,201.536128323692));
#30125=CARTESIAN_POINT('Ctrl Pts',(74.7548697221244,72.5824014579692,201.565611729204));
#30126=CARTESIAN_POINT('Ctrl Pts',(76.8348627554146,72.2065251754741,201.626029557126));
#30127=CARTESIAN_POINT('Ctrl Pts',(77.9218751377021,72.228201927325,201.658616729351));
#30128=CARTESIAN_POINT('Ctrl Pts',(79.9854219362805,72.6867079499083,201.72241666865));
#30129=CARTESIAN_POINT('Ctrl Pts',(80.9454462136871,73.1041483757411,201.752011531474));
#30130=CARTESIAN_POINT('Ctrl Pts',(82.688556916364,74.3009367306872,201.812345948119));
#30131=CARTESIAN_POINT('Ctrl Pts',(83.4460459700937,75.0816302105106,201.844927994003));
#30132=CARTESIAN_POINT('Ctrl Pts',(84.5898541948341,76.8602014006922,201.908769379002));
#30133=CARTESIAN_POINT('Ctrl Pts',(84.978188276254,77.8325937969514,201.938473901633));
#30134=CARTESIAN_POINT('Ctrl Pts',(85.3743549930091,79.9102875085715,201.998728813384));
#30135=CARTESIAN_POINT('Ctrl Pts',(85.3629298992261,80.9985354452161,202.0313053181));
#30136=CARTESIAN_POINT('Ctrl Pts',(84.9232223320722,83.0676784708673,202.09518523474));
#30137=CARTESIAN_POINT('Ctrl Pts',(84.5144310737503,84.0318929266988,202.124997052606));
#30138=CARTESIAN_POINT('Ctrl Pts',(83.3327545004861,85.7869845925951,202.185176368123));
#30139=CARTESIAN_POINT('Ctrl Pts',(82.5581157282637,86.5521173931964,202.21774702605));
#30140=CARTESIAN_POINT('Ctrl Pts',(80.7883960140716,87.7121957815709,202.281662719573));
#30141=CARTESIAN_POINT('Ctrl Pts',(79.8189762333589,88.1090956952885,202.311578989822));
#30142=CARTESIAN_POINT('Ctrl Pts',(77.7434069598192,88.5233170270438,202.371686591791));
#30143=CARTESIAN_POINT('Ctrl Pts',(76.6541382901548,88.5210265687059,202.404251194614));
#30144=CARTESIAN_POINT('Ctrl Pts',(74.5800853029275,88.0980732750149,202.468200068939));
#30145=CARTESIAN_POINT('Ctrl Pts',(73.6121445296276,87.6969649715002,202.498217555134));
#30146=CARTESIAN_POINT('Ctrl Pts',(71.8464791513764,86.5287362676304,202.558257275313));
#30147=CARTESIAN_POINT('Ctrl Pts',(71.0746108794289,85.7595227767601,202.590815700345));
#30148=CARTESIAN_POINT('Ctrl Pts',(70.4221941385349,84.7808451037534,202.626356078363));
#30149=CARTESIAN_POINT('Ctrl Pts',(70.3697490250245,84.6990148765756,202.629290135917));
#30150=CARTESIAN_POINT('Ctrl Pts',(70.3188266908911,84.6163270097798,202.632217951621));
#30151=CARTESIAN_POINT('Ctrl Pts',(70.3188266910146,84.6163270099805,201.781598171062));
#30152=CARTESIAN_POINT('Ctrl Pts',(70.6346499752365,85.1291619791441,201.763439687425));
#30153=CARTESIAN_POINT('Ctrl Pts',(71.0074275501507,85.6063726542895,201.745134356569));
#30154=CARTESIAN_POINT('Ctrl Pts',(72.1651851227176,86.7876714914651,201.695626618392));
#30155=CARTESIAN_POINT('Ctrl Pts',(73.0379884544506,87.3871121495928,201.666968157683));
#30156=CARTESIAN_POINT('Ctrl Pts',(74.9698735097578,88.2225480250084,201.605353172529));
#30157=CARTESIAN_POINT('Ctrl Pts',(76.0115921888612,88.4481283097861,201.573173028118));
#30158=CARTESIAN_POINT('Ctrl Pts',(78.1173401778328,88.4867821887547,201.510061026804));
#30159=CARTESIAN_POINT('Ctrl Pts',(79.1612477309362,88.3016270442561,201.481291699509));
#30160=CARTESIAN_POINT('Ctrl Pts',(81.1244989095788,87.5414248151742,201.419788608629));
#30161=CARTESIAN_POINT('Ctrl Pts',(82.0244543490064,86.9719281445366,201.387650380247));
#30162=CARTESIAN_POINT('Ctrl Pts',(83.5529616295436,85.5222393134006,201.324454466035));
#30163=CARTESIAN_POINT('Ctrl Pts',(84.1678129225914,84.6568089217546,201.29556532486));
#30164=CARTESIAN_POINT('Ctrl Pts',(85.0333440550814,82.7370483636183,201.234172975973));
#30165=CARTESIAN_POINT('Ctrl Pts',(85.2748712972383,81.7006392555677,201.202077479976));
#30166=CARTESIAN_POINT('Ctrl Pts',(85.347256719068,79.5946582363799,201.138801915413));
#30167=CARTESIAN_POINT('Ctrl Pts',(85.1778473710755,78.545202808651,201.109785196217));
#30168=CARTESIAN_POINT('Ctrl Pts',(84.4467539234772,76.5696790931711,201.048502055368));
#30169=CARTESIAN_POINT('Ctrl Pts',(83.8919287680293,75.6625209770227,201.01644985588));
#30170=CARTESIAN_POINT('Ctrl Pts',(82.4654008385435,74.1107318072355,200.953098924926));
#30171=CARTESIAN_POINT('Ctrl Pts',(81.6070029673053,73.4812132857151,200.923948082438));
#30172=CARTESIAN_POINT('Ctrl Pts',(79.698894063828,72.5873146266685,200.86277225941));
#30173=CARTESIAN_POINT('Ctrl Pts',(78.667716588934,72.330828984707,200.830763671953));
#30174=CARTESIAN_POINT('Ctrl Pts',(76.5617866497835,72.2265656625823,200.767341640629));
#30175=CARTESIAN_POINT('Ctrl Pts',(75.5070939175263,72.3810654616141,200.738051358696));
#30176=CARTESIAN_POINT('Ctrl Pts',(73.5202164800736,73.0847288407394,200.676980636246));
#30177=CARTESIAN_POINT('Ctrl Pts',(72.6065080593912,73.6257036645629,200.645015735532));
#30178=CARTESIAN_POINT('Ctrl Pts',(71.0330250648484,75.0302888775848,200.581526816573));
#30179=CARTESIAN_POINT('Ctrl Pts',(70.3897088999477,75.8820534253532,200.552092994835));
#30180=CARTESIAN_POINT('Ctrl Pts',(69.4693695179899,77.7791056656777,200.491124860899));
#30181=CARTESIAN_POINT('Ctrl Pts',(69.1990100576524,78.80520960397,200.459203492272));
#30182=CARTESIAN_POINT('Ctrl Pts',(69.0649627904852,80.9108509365622,200.395651814124));
#30183=CARTESIAN_POINT('Ctrl Pts',(69.2055019588525,81.9704299535114,200.366071533627));
#30184=CARTESIAN_POINT('Ctrl Pts',(69.7415482612329,83.5492937006154,200.317954575517));
#30185=CARTESIAN_POINT('Ctrl Pts',(70.001111301679,84.10041963382,200.299865442624));
#30186=CARTESIAN_POINT('Ctrl Pts',(70.3188266910085,84.6163270099704,200.281598171063));
#30187=CARTESIAN_POINT('Origin',(77.215862801455,80.368869783441,202.950490121702));
#30188=CARTESIAN_POINT('',(70.3188266909419,84.6163270098623,198.781598171064));
#30189=CARTESIAN_POINT('',(70.318826690899,84.6163270097926,199.63221795162));
#30190=CARTESIAN_POINT('',(70.3188266908911,84.6163270097798,202.950490121702));
#30191=CARTESIAN_POINT('Ctrl Pts',(70.3188266909068,84.6163270098053,199.63221795162));
#30192=CARTESIAN_POINT('Ctrl Pts',(70.2393441858636,84.4872630361786,199.636787854599));
#30193=CARTESIAN_POINT('Ctrl Pts',(70.1634077264338,84.3558435843596,199.641351970946));
#30194=CARTESIAN_POINT('Ctrl Pts',(69.5914552814193,83.2983166682045,199.677381204738));
#30195=CARTESIAN_POINT('Ctrl Pts',(69.2762289647801,82.2860188469412,199.706154022544));
#30196=CARTESIAN_POINT('Ctrl Pts',(69.049346466731,80.1929696435868,199.76765375273));
#30197=CARTESIAN_POINT('Ctrl Pts',(69.1416437199601,79.1319920852377,199.799790702254));
#30198=CARTESIAN_POINT('Ctrl Pts',(69.72689956906,77.1082630134724,199.862989082657));
#30199=CARTESIAN_POINT('Ctrl Pts',(70.213067098747,76.1644705992131,199.8918819662));
#30200=CARTESIAN_POINT('Ctrl Pts',(71.5204958144094,74.5136133971232,199.953270995215));
#30201=CARTESIAN_POINT('Ctrl Pts',(72.3300247830745,73.8228966637599,199.985365191647));
#30202=CARTESIAN_POINT('Ctrl Pts',(74.1529397406286,72.7989829593244,200.048149141923));
#30203=CARTESIAN_POINT('Ctrl Pts',(75.1458801342046,72.4695128292969,200.076773411079));
#30204=CARTESIAN_POINT('Ctrl Pts',(77.2362417195835,72.1983692987134,200.137987336794));
#30205=CARTESIAN_POINT('Ctrl Pts',(78.3153946330038,72.2726695921714,200.170583925419));
#30206=CARTESIAN_POINT('Ctrl Pts',(80.3487608864749,72.8276873702844,200.233929942969));
#30207=CARTESIAN_POINT('Ctrl Pts',(81.2870999465542,73.2900641784442,200.262649225009));
#30208=CARTESIAN_POINT('Ctrl Pts',(82.9666836821889,74.564801845728,200.323752854912));
#30209=CARTESIAN_POINT('Ctrl Pts',(83.6834821369912,75.3759773993898,200.35635280953));
#30210=CARTESIAN_POINT('Ctrl Pts',(84.7418259215178,77.1995991904948,200.419768590968));
#30211=CARTESIAN_POINT('Ctrl Pts',(85.0852147287464,78.1876618288599,200.448588621887));
#30212=CARTESIAN_POINT('Ctrl Pts',(85.3860521089365,80.2753408185713,200.509584521462));
#30213=CARTESIAN_POINT('Ctrl Pts',(85.3266158971152,81.3569733667024,200.542186210058));
#30214=CARTESIAN_POINT('Ctrl Pts',(84.7988723170437,83.3991143600469,200.605667849549));
#30215=CARTESIAN_POINT('Ctrl Pts',(84.349290528312,84.3436134559467,200.63459320526));
#30216=CARTESIAN_POINT('Ctrl Pts',(83.0966406729893,86.0414996244146,200.695484249101));
#30217=CARTESIAN_POINT('Ctrl Pts',(82.2939699054705,86.7700434490427,200.728086209688));
#30218=CARTESIAN_POINT('Ctrl Pts',(80.4830103856543,87.8528709165616,200.791629868083));
#30219=CARTESIAN_POINT('Ctrl Pts',(79.4994484969199,88.2091323257396,200.820664000294));
#30220=CARTESIAN_POINT('Ctrl Pts',(77.4144256644832,88.5373657539617,200.881453331427));
#30221=CARTESIAN_POINT('Ctrl Pts',(76.3306814324689,88.4916846307376,200.914054271892));
#30222=CARTESIAN_POINT('Ctrl Pts',(74.2805969035862,87.9891671339348,200.97765620027));
#30223=CARTESIAN_POINT('Ctrl Pts',(73.3304235899278,87.5513501534359,201.006801489692));
#30224=CARTESIAN_POINT('Ctrl Pts',(71.6183120197023,86.3208529792364,201.067405589061));
#30225=CARTESIAN_POINT('Ctrl Pts',(70.8807822911543,85.5288325068369,201.09990791597));
#30226=CARTESIAN_POINT('Ctrl Pts',(70.3188266908911,84.6163270097798,201.132217951621));
#30227=CARTESIAN_POINT('Ctrl Pts',(70.3188266910085,84.6163270099704,200.281598171063));
#30228=CARTESIAN_POINT('Ctrl Pts',(70.5494760509144,84.990856258714,200.26833682259));
#30229=CARTESIAN_POINT('Ctrl Pts',(70.8107716985665,85.346825340615,200.254981594731));
#30230=CARTESIAN_POINT('Ctrl Pts',(71.7956911801604,86.4807937792226,200.209714589911));
#30231=CARTESIAN_POINT('Ctrl Pts',(72.6412648242632,87.1369478572639,200.179986060603));
#30232=CARTESIAN_POINT('Ctrl Pts',(74.5279489603352,88.0816765747758,200.119214561012));
#30233=CARTESIAN_POINT('Ctrl Pts',(75.5492051502349,88.3647710802179,200.087378950053));
#30234=CARTESIAN_POINT('Ctrl Pts',(77.6543705112786,88.5263515257473,200.023713673883));
#30235=CARTESIAN_POINT('Ctrl Pts',(78.7184587991564,88.3987480480752,199.993836167195));
#30236=CARTESIAN_POINT('Ctrl Pts',(80.7251668609644,87.7442181246045,199.933158299535));
#30237=CARTESIAN_POINT('Ctrl Pts',(81.6500361236621,87.228096915081,199.901364537007));
#30238=CARTESIAN_POINT('Ctrl Pts',(83.2617789132175,85.8631001076693,199.837648139127));
#30239=CARTESIAN_POINT('Ctrl Pts',(83.9297566222614,85.0232472997634,199.807621908919));
#30240=CARTESIAN_POINT('Ctrl Pts',(84.8967679163405,83.1461787161077,199.747034333491));
#30241=CARTESIAN_POINT('Ctrl Pts',(85.1914422263021,82.1294915496872,199.715281513417));
#30242=CARTESIAN_POINT('Ctrl Pts',(85.3782270383223,80.0249398293957,199.65151756514));
#30243=CARTESIAN_POINT('Ctrl Pts',(85.2624934312454,78.9567316649269,199.621343760249));
#30244=CARTESIAN_POINT('Ctrl Pts',(84.6211639777199,76.9150092839013,199.560046631192));
#30245=CARTESIAN_POINT('Ctrl Pts',(84.0974234210483,75.963003022243,199.527454303479));
#30246=CARTESIAN_POINT('Ctrl Pts',(82.7337030830622,74.3489818669681,199.46370506325));
#30247=CARTESIAN_POINT('Ctrl Pts',(81.9184130962896,73.6926772458593,199.43423663281));
#30248=CARTESIAN_POINT('Ctrl Pts',(80.0498760145395,72.7048473490567,199.373807380033));
#30249=CARTESIAN_POINT('Ctrl Pts',(79.0073788716093,72.3964650338568,199.341219561468));
#30250=CARTESIAN_POINT('Ctrl Pts',(76.9019593562372,72.2087547767503,199.277425381815));
#30251=CARTESIAN_POINT('Ctrl Pts',(75.8606373243966,72.3159647763489,199.247845301973));
#30252=CARTESIAN_POINT('Ctrl Pts',(73.8370986097,72.9288433392431,199.187499979936));
#30253=CARTESIAN_POINT('Ctrl Pts',(72.8788631864418,73.443527337106,199.154917223455));
#30254=CARTESIAN_POINT('Ctrl Pts',(71.2503195670516,74.7922455908759,199.091081197233));
#30255=CARTESIAN_POINT('Ctrl Pts',(70.5858156746814,75.6013956219914,199.061391182953));
#30256=CARTESIAN_POINT('Ctrl Pts',(69.5792063812086,77.461529421012,199.001125887885));
#30257=CARTESIAN_POINT('Ctrl Pts',(69.2606031890589,78.5020856953131,198.968548623791));
#30258=CARTESIAN_POINT('Ctrl Pts',(69.0531349771153,80.6071381987141,198.904673686263));
#30259=CARTESIAN_POINT('Ctrl Pts',(69.1507593252483,81.6498393210891,198.874876031648));
#30260=CARTESIAN_POINT('Ctrl Pts',(69.6458614565071,83.3402031113327,198.824767605201));
#30261=CARTESIAN_POINT('Ctrl Pts',(69.9409909796789,84.0027960417003,198.803322103162));
#30262=CARTESIAN_POINT('Ctrl Pts',(70.3188266909927,84.6163270099447,198.781598171064));
#30263=CARTESIAN_POINT('Origin',(77.215862801455,80.368869783441,202.950490121702));
#30264=CARTESIAN_POINT('',(70.318826690926,84.6163270098365,197.281598171066));
#30265=CARTESIAN_POINT('',(70.3188266909362,84.6163270098531,198.132217951616));
#30266=CARTESIAN_POINT('',(70.3188266908911,84.6163270097798,202.950490121702));
#30267=CARTESIAN_POINT('',(75.3015616260917,72.4983265359896,196.230940107676));
#30268=CARTESIAN_POINT('Ctrl Pts',(70.3188266909609,84.6163270098932,197.281598171066));
#30269=CARTESIAN_POINT('Ctrl Pts',(70.4672117059276,84.8572751235334,197.273066669429));
#30270=CARTESIAN_POINT('Ctrl Pts',(70.6284024015044,85.0907395806919,197.264489304094));
#30271=CARTESIAN_POINT('Ctrl Pts',(71.4368717282468,86.1389942955801,197.224464651716));
#30272=CARTESIAN_POINT('Ctrl Pts',(72.2244576005149,86.8323619240314,197.193856836177));
#30273=CARTESIAN_POINT('Ctrl Pts',(74.0544848742302,87.9044441075959,197.134187348814));
#30274=CARTESIAN_POINT('Ctrl Pts',(75.0875048590491,88.2586825940275,197.101669877795));
#30275=CARTESIAN_POINT('Ctrl Pts',(77.1905611236561,88.5353160193394,197.037533500101));
#30276=CARTESIAN_POINT('Ctrl Pts',(78.2381050913792,88.4711088330216,197.006855826311));
#30277=CARTESIAN_POINT('Ctrl Pts',(80.2918553536182,87.9397354292445,196.947227736429));
#30278=CARTESIAN_POINT('Ctrl Pts',(81.2740996783364,87.4618459870212,196.914715572296));
#30279=CARTESIAN_POINT('Ctrl Pts',(82.959969005163,86.1737918459698,196.850562764639));
#30280=CARTESIAN_POINT('Ctrl Pts',(83.6571133639445,85.3890222970249,196.819819237289));
#30281=CARTESIAN_POINT('Ctrl Pts',(84.7376864138108,83.562991640004,196.76022977423));
#30282=CARTESIAN_POINT('Ctrl Pts',(85.0965441593794,82.5310366958102,196.727722688161));
#30283=CARTESIAN_POINT('Ctrl Pts',(85.3821786975059,80.4283223688934,196.663554741923));
#30284=CARTESIAN_POINT('Ctrl Pts',(85.3223066388472,79.3801465048748,196.632749261312));
#30285=CARTESIAN_POINT('Ctrl Pts',(84.7991430709567,77.3234506679724,196.573195798819));
#30286=CARTESIAN_POINT('Ctrl Pts',(84.3249937825088,76.3388782270904,196.540693554184));
#30287=CARTESIAN_POINT('Ctrl Pts',(83.0430855394691,74.6473245170452,196.476511663731));
#30288=CARTESIAN_POINT('Ctrl Pts',(82.2607486008549,73.9469168163812,196.445648007422));
#30289=CARTESIAN_POINT('Ctrl Pts',(80.4381814533099,72.8590216837296,196.386128062267));
#30290=CARTESIAN_POINT('Ctrl Pts',(79.4071611147434,72.4961812791765,196.353630418377));
#30291=CARTESIAN_POINT('Ctrl Pts',(77.3236635410519,72.205417441165,196.290012972736));
#30292=CARTESIAN_POINT('Ctrl Pts',(76.2942419888476,72.2568833311894,196.259486529753));
#30293=CARTESIAN_POINT('Ctrl Pts',(75.3015616260917,72.4983265359896,196.230940107676));
#30294=CARTESIAN_POINT('',(75.3015616260917,72.4983265359896,197.081559888227));
#30295=CARTESIAN_POINT('',(75.3015616260917,72.4983265359896,202.950490121702));
#30296=CARTESIAN_POINT('Ctrl Pts',(75.3015616260917,72.4983265359896,197.081559888227));
#30297=CARTESIAN_POINT('Ctrl Pts',(76.1388972823187,72.2946668163879,197.105639076212));
#30298=CARTESIAN_POINT('Ctrl Pts',(77.0033661482917,72.2259366208603,197.131155580565));
#30299=CARTESIAN_POINT('Ctrl Pts',(78.7315041943876,72.364297891176,197.18344519351));
#30300=CARTESIAN_POINT('Ctrl Pts',(79.5837955806926,72.5737898395195,197.209889408713));
#30301=CARTESIAN_POINT('Ctrl Pts',(81.3413422722311,73.321337767,197.265886083455));
#30302=CARTESIAN_POINT('Ctrl Pts',(82.2095133426904,73.9073883603634,197.294186427988));
#30303=CARTESIAN_POINT('Ctrl Pts',(83.6976207414577,75.3955000355644,197.35708183513));
#30304=CARTESIAN_POINT('Ctrl Pts',(84.2954742747404,76.2912814451157,197.389624320124));
#30305=CARTESIAN_POINT('Ctrl Pts',(85.0989511242683,78.2369163591494,197.451469750634));
#30306=CARTESIAN_POINT('Ctrl Pts',(85.3070670685511,79.2640083597879,197.479726448372));
#30307=CARTESIAN_POINT('Ctrl Pts',(85.3243366751421,81.3680350452673,197.542527381558));
#30308=CARTESIAN_POINT('Ctrl Pts',(85.1226940733133,82.4250130682218,197.575052437086));
#30309=CARTESIAN_POINT('Ctrl Pts',(84.3318171518148,84.3754507528462,197.637015022373));
#30310=CARTESIAN_POINT('Ctrl Pts',(83.7597793243371,85.2542205198593,197.665240601487));
#30311=CARTESIAN_POINT('Ctrl Pts',(82.2969958342311,86.7661999260792,197.727943723931));
#30312=CARTESIAN_POINT('Ctrl Pts',(81.4129558227272,87.37801921126,197.760448825333));
#30313=CARTESIAN_POINT('Ctrl Pts',(79.4819616351216,88.2146112337875,197.822527899281));
#30314=CARTESIAN_POINT('Ctrl Pts',(78.4573165640372,88.4404033069567,197.850735560505));
#30315=CARTESIAN_POINT('Ctrl Pts',(76.3544674416585,88.4928955888731,197.913337779465));
#30316=CARTESIAN_POINT('Ctrl Pts',(75.2960506701693,88.3096588978678,197.945820383995));
#30317=CARTESIAN_POINT('Ctrl Pts',(73.3325354514835,87.5530310304496,198.008014804058));
#30318=CARTESIAN_POINT('Ctrl Pts',(72.4428601018535,86.9953958706751,198.036218254823));
#30319=CARTESIAN_POINT('Ctrl Pts',(71.1549043755846,85.7908277885468,198.088618145068));
#30320=CARTESIAN_POINT('Ctrl Pts',(70.696419591884,85.2294637017675,198.110507980075));
#30321=CARTESIAN_POINT('Ctrl Pts',(70.3188266909814,84.6163270099265,198.132217951616));
#30322=CARTESIAN_POINT('Origin',(77.215862801455,80.368869783441,202.950490121702));
#30323=CARTESIAN_POINT('Ctrl Pts',(70.3188266909814,84.6163270099264,198.132217951616));
#30324=CARTESIAN_POINT('Ctrl Pts',(70.1413522775646,84.3281434279028,198.14242196884));
#30325=CARTESIAN_POINT('Ctrl Pts',(69.9817464533539,84.0285235129716,198.152586256108));
#30326=CARTESIAN_POINT('Ctrl Pts',(69.4105242617287,82.7711208473259,198.19348250062));
#30327=CARTESIAN_POINT('Ctrl Pts',(69.166673393273,81.74896734013,198.22169577383));
#30328=CARTESIAN_POINT('Ctrl Pts',(69.0784407110988,79.6475902217734,198.284088075341));
#30329=CARTESIAN_POINT('Ctrl Pts',(69.2430030358506,78.5880302005555,198.316518151265));
#30330=CARTESIAN_POINT('Ctrl Pts',(69.9647537190728,76.6115536643663,198.378938016748));
#30331=CARTESIAN_POINT('Ctrl Pts',(70.5077748665416,75.7108053684881,198.407175252907));
#30332=CARTESIAN_POINT('Ctrl Pts',(71.9180205367237,74.1504457791517,198.469459225153));
#30333=CARTESIAN_POINT('Ctrl Pts',(72.777309908536,73.5106505239144,198.501859398185));
#30334=CARTESIAN_POINT('Ctrl Pts',(74.6773605643387,72.6065204667344,198.564388520805));
#30335=CARTESIAN_POINT('Ctrl Pts',(75.69700422083,72.3444613591024,198.592663796792));
#30336=CARTESIAN_POINT('Ctrl Pts',(77.7966308120636,72.2204529179664,198.654837692736));
#30337=CARTESIAN_POINT('Ctrl Pts',(78.8570154818378,72.3663330781034,198.687205682111));
#30338=CARTESIAN_POINT('Ctrl Pts',(80.8461512194974,73.0530460903665,198.749841218891));
#30339=CARTESIAN_POINT('Ctrl Pts',(81.7579907861586,73.581429485084,198.778168379625));
#30340=CARTESIAN_POINT('Ctrl Pts',(83.3422023416221,74.9651645597405,198.840230840417));
#30341=CARTESIAN_POINT('Ctrl Pts',(83.9956095848265,75.8117785632511,198.872564511952));
#30342=CARTESIAN_POINT('Ctrl Pts',(84.9332439357261,77.6959210616337,198.935303278946));
#30343=CARTESIAN_POINT('Ctrl Pts',(85.2134215592527,78.713067021492,198.963695721928));
#30344=CARTESIAN_POINT('Ctrl Pts',(85.3727593018409,80.8106928555144,199.025645806591));
#30345=CARTESIAN_POINT('Ctrl Pts',(85.2453091984721,81.8715783097193,199.0579432008));
#30346=CARTESIAN_POINT('Ctrl Pts',(84.5933209928205,83.8728999526277,199.120781716382));
#30347=CARTESIAN_POINT('Ctrl Pts',(84.0794091641949,84.7957027711809,199.149252215542));
#30348=CARTESIAN_POINT('Ctrl Pts',(82.7218679072689,86.4031226790794,199.211089410695));
#30349=CARTESIAN_POINT('Ctrl Pts',(81.8878888578483,87.0696489005427,199.243348767287));
#30350=CARTESIAN_POINT('Ctrl Pts',(80.0196578434461,88.0400144799904,199.306283298298));
#30351=CARTESIAN_POINT('Ctrl Pts',(79.0049690157344,88.3379869113588,199.334843844877));
#30352=CARTESIAN_POINT('Ctrl Pts',(76.9095526933233,88.5317517568567,199.39656806787));
#30353=CARTESIAN_POINT('Ctrl Pts',(75.8484785462801,88.4222349338808,199.428787846007));
#30354=CARTESIAN_POINT('Ctrl Pts',(73.8355883492947,87.804203559603,199.491814455515));
#30355=CARTESIAN_POINT('Ctrl Pts',(72.9020920155522,87.3044176972546,199.520476119952));
#30356=CARTESIAN_POINT('Ctrl Pts',(71.3900198791337,86.0685626015633,199.577640350897));
#30357=CARTESIAN_POINT('Ctrl Pts',(70.7916687049813,85.3841295495084,199.605031564789));
#30358=CARTESIAN_POINT('Ctrl Pts',(70.3188266909068,84.6163270098053,199.63221795162));
#30359=CARTESIAN_POINT('Ctrl Pts',(70.3188266909927,84.6163270099447,198.781598171064));
#30360=CARTESIAN_POINT('Ctrl Pts',(70.5038298807908,84.9167358457598,198.770961281504));
#30361=CARTESIAN_POINT('Ctrl Pts',(70.7086598717006,85.205383306225,198.760257644138));
#30362=CARTESIAN_POINT('Ctrl Pts',(71.587249389392,86.2854632173503,198.71820432847));
#30363=CARTESIAN_POINT('Ctrl Pts',(72.390925193891,86.9572847581389,198.68830181755));
#30364=CARTESIAN_POINT('Ctrl Pts',(74.2435020092774,87.9805881515105,198.628184868632));
#30365=CARTESIAN_POINT('Ctrl Pts',(75.2822503678208,88.308278486667,198.595619448935));
#30366=CARTESIAN_POINT('Ctrl Pts',(77.3869003895154,88.533341078713,198.531674857992));
#30367=CARTESIAN_POINT('Ctrl Pts',(78.4308312232629,88.4442368646137,198.501670679398));
#30368=CARTESIAN_POINT('Ctrl Pts',(80.4673097402838,87.8656830225203,198.441622119844));
#30369=CARTESIAN_POINT('Ctrl Pts',(81.43585444097,87.366416915855,198.409062866107));
#30370=CARTESIAN_POINT('Ctrl Pts',(83.0887376501164,86.0431687325628,198.345087217402));
#30371=CARTESIAN_POINT('Ctrl Pts',(83.7670434343762,85.244339479377,198.314984884182));
#30372=CARTESIAN_POINT('Ctrl Pts',(84.8050863821067,83.3985028320405,198.255000943989));
#30373=CARTESIAN_POINT('Ctrl Pts',(85.1407999985339,82.361415368789,198.222447913808));
#30374=CARTESIAN_POINT('Ctrl Pts',(85.381420595943,80.2571809134547,198.158443514381));
#30375=CARTESIAN_POINT('Ctrl Pts',(85.2998387937799,79.212161411866,198.12824678984));
#30376=CARTESIAN_POINT('Ctrl Pts',(84.7355441492512,77.1704006602766,198.068323787707));
#30377=CARTESIAN_POINT('Ctrl Pts',(84.2427169191899,76.1976580453656,198.035776973544));
#30378=CARTESIAN_POINT('Ctrl Pts',(82.930082792761,74.5347482518195,197.971745981676));
#30379=CARTESIAN_POINT('Ctrl Pts',(82.1355176169891,73.8507332996321,197.941458811811));
#30380=CARTESIAN_POINT('Ctrl Pts',(80.2956487101043,72.7997548517861,197.881593170842));
#30381=CARTESIAN_POINT('Ctrl Pts',(79.2600688353045,72.4570005266266,197.849052510037));
#30382=CARTESIAN_POINT('Ctrl Pts',(77.1562459994661,72.2027080806856,197.784996940664));
#30383=CARTESIAN_POINT('Ctrl Pts',(76.1102688351415,72.2776878585382,197.754623393498));
#30384=CARTESIAN_POINT('Ctrl Pts',(74.0639176042385,72.829470336233,197.694811653939));
#30385=CARTESIAN_POINT('Ctrl Pts',(73.0875324344894,73.3166318441385,197.662277037938));
#30386=CARTESIAN_POINT('Ctrl Pts',(71.4158653900587,74.6199362622047,197.598198768693));
#30387=CARTESIAN_POINT('Ctrl Pts',(70.726852071004,75.4107705712388,197.567742980565));
#30388=CARTESIAN_POINT('Ctrl Pts',(69.6645815554747,77.2453897532126,197.507981809798));
#30389=CARTESIAN_POINT('Ctrl Pts',(69.3156818670123,78.279615370696,197.475453092547));
#30390=CARTESIAN_POINT('Ctrl Pts',(69.049440848975,80.3830427593049,197.411353870224));
#30391=CARTESIAN_POINT('Ctrl Pts',(69.1186568230227,81.4298576069505,197.380819998922));
#30392=CARTESIAN_POINT('Ctrl Pts',(69.5870600798276,83.2055036450499,197.329105944861));
#30393=CARTESIAN_POINT('Ctrl Pts',(69.9025454780671,83.9403680998025,197.305532554534));
#30394=CARTESIAN_POINT('Ctrl Pts',(70.3188266909609,84.6163270098932,197.281598171066));
#30395=CARTESIAN_POINT('Origin',(77.215862801455,80.368869783441,202.750490121702));
#30396=CARTESIAN_POINT('',(81.6703452938459,91.5114720703838,202.750490121702));
#30397=CARTESIAN_POINT('',(85.1614376461066,89.3615245854469,202.750490121702));
#30398=CARTESIAN_POINT('Origin',(77.215862801455,80.368869783441,202.750490121702));
#30399=CARTESIAN_POINT('',(85.1490627147209,89.3414301279668,202.750490121702));
#30400=CARTESIAN_POINT('',(85.1490627147209,89.3414301279668,202.750490121702));
#30401=CARTESIAN_POINT('',(81.6579703624602,91.4913776129038,202.750490121702));
#30402=CARTESIAN_POINT('',(85.1490627147209,89.3414301279668,202.750490121702));
#30403=CARTESIAN_POINT('',(81.6579703624602,91.4913776129038,202.750490121702));
#30404=CARTESIAN_POINT('Origin',(85.1490627147209,89.3414301279668,192.750490121702));
#30405=CARTESIAN_POINT('',(85.1490627147209,89.3414301279668,196.17168857984));
#30406=CARTESIAN_POINT('',(81.6579703624602,91.4913776129038,196.17168857984));
#30407=CARTESIAN_POINT('Ctrl Pts',(85.1490627147208,89.3414301279668,196.17168857984));
#30408=CARTESIAN_POINT('Ctrl Pts',(83.4035165385905,90.4164038704353,195.897880393518));
#30409=CARTESIAN_POINT('Ctrl Pts',(81.6579703624602,91.4913776129037,196.17168857984));
#30410=CARTESIAN_POINT('',(81.6579703624602,91.4913776129038,192.750490121702));
#30411=CARTESIAN_POINT('',(85.1490627147209,89.3414301279668,192.750490121702));
#30412=CARTESIAN_POINT('Origin',(85.1490627147209,89.3414301279668,192.750490121702));
#30413=CARTESIAN_POINT('',(86.223563176935,91.0862077899414,197.750490121702));
#30414=CARTESIAN_POINT('Ctrl Pts',(86.223563176935,91.0862077899414,197.750490121702));
#30415=CARTESIAN_POINT('Ctrl Pts',(85.6444681226414,90.1458711866332,196.898024398674));
#30416=CARTESIAN_POINT('Ctrl Pts',(85.1490627147209,89.3414301279668,196.17168857984));
#30417=CARTESIAN_POINT('',(86.223563176935,91.0862077899414,202.750490121702));
#30418=CARTESIAN_POINT('',(85.1490627147209,89.3414301279668,202.750490121702));
#30419=CARTESIAN_POINT('',(86.223563176935,91.0862077899414,202.950490121702));
#30420=CARTESIAN_POINT('Origin',(81.6579703624602,91.4913776129038,192.750490121702));
#30421=CARTESIAN_POINT('',(82.7324708246743,93.2361552748783,197.750490121702));
#30422=CARTESIAN_POINT('Ctrl Pts',(81.6579703624601,91.4913776129037,196.17168857984));
#30423=CARTESIAN_POINT('Ctrl Pts',(82.1533757703807,92.2958186715703,196.898024398674));
#30424=CARTESIAN_POINT('Ctrl Pts',(82.7324708246743,93.2361552748783,197.750490121702));
#30425=CARTESIAN_POINT('',(82.7324708246743,93.2361552748783,202.750490121702));
#30426=CARTESIAN_POINT('',(82.7324708246743,93.2361552748783,202.950490121702));
#30427=CARTESIAN_POINT('',(81.6579703624602,91.4913776129038,202.750490121702));
#30428=CARTESIAN_POINT('Origin',(77.215862801455,80.368869783441,202.750490121702));
#30429=CARTESIAN_POINT('',(86.1884231459808,72.435669870175,202.750490121702));
#30430=CARTESIAN_POINT('',(86.2085176034608,72.4232949387893,202.750490121702));
#30431=CARTESIAN_POINT('',(86.1884231459808,72.435669870175,202.750490121702));
#30432=CARTESIAN_POINT('',(88.3383706309178,75.9267622224358,202.750490121702));
#30433=CARTESIAN_POINT('',(86.1884231459808,72.435669870175,202.750490121702));
#30434=CARTESIAN_POINT('',(88.3584650883978,75.9143872910501,202.750490121702));
#30435=CARTESIAN_POINT('',(88.3383706309178,75.9267622224358,202.750490121702));
#30436=CARTESIAN_POINT('Origin',(77.215862801455,80.368869783441,202.750490121702));
#30437=CARTESIAN_POINT('Origin',(88.3383706309178,75.9267622224358,192.750490121702));
#30438=CARTESIAN_POINT('',(88.3383706309178,75.9267622224358,196.17168857984));
#30439=CARTESIAN_POINT('',(90.0831482928923,74.8522617602217,197.750490121702));
#30440=CARTESIAN_POINT('Ctrl Pts',(88.3383706309177,75.9267622224358,196.17168857984));
#30441=CARTESIAN_POINT('Ctrl Pts',(89.1428116895835,75.4313568145157,196.898024398673));
#30442=CARTESIAN_POINT('Ctrl Pts',(90.0831482928923,74.8522617602217,197.750490121702));
#30443=CARTESIAN_POINT('',(90.0831482928923,74.8522617602217,202.750490121702));
#30444=CARTESIAN_POINT('',(90.0831482928923,74.8522617602217,202.950490121702));
#30445=CARTESIAN_POINT('',(88.3383706309178,75.9267622224358,202.750490121702));
#30446=CARTESIAN_POINT('',(88.3383706309178,75.9267622224358,192.750490121702));
#30447=CARTESIAN_POINT('Origin',(86.1884231459808,72.435669870175,192.750490121702));
#30448=CARTESIAN_POINT('',(86.1884231459808,72.435669870175,196.17168857984));
#30449=CARTESIAN_POINT('Ctrl Pts',(86.1884231459808,72.435669870175,196.17168857984));
#30450=CARTESIAN_POINT('Ctrl Pts',(87.2633968884493,74.1812160463054,195.897880393518));
#30451=CARTESIAN_POINT('Ctrl Pts',(88.3383706309177,75.9267622224357,196.17168857984));
#30452=CARTESIAN_POINT('',(86.1884231459808,72.435669870175,192.750490121702));
#30453=CARTESIAN_POINT('Origin',(86.1884231459808,72.435669870175,192.750490121702));
#30454=CARTESIAN_POINT('',(87.9332008079553,71.3611694079609,197.750490121702));
#30455=CARTESIAN_POINT('Ctrl Pts',(87.9332008079553,71.3611694079609,197.750490121702));
#30456=CARTESIAN_POINT('Ctrl Pts',(86.9928642046467,71.9402644622549,196.898024398673));
#30457=CARTESIAN_POINT('Ctrl Pts',(86.1884231459808,72.435669870175,196.17168857984));
#30458=CARTESIAN_POINT('',(87.9332008079553,71.3611694079609,202.750490121702));
#30459=CARTESIAN_POINT('',(86.1884231459808,72.435669870175,202.750490121702));
#30460=CARTESIAN_POINT('',(87.9332008079553,71.3611694079609,202.950490121702));
#30461=CARTESIAN_POINT('Origin',(77.215862801455,80.368869783441,202.750490121702));
#30462=CARTESIAN_POINT('',(69.2826628881893,71.396309438915,202.750490121702));
#30463=CARTESIAN_POINT('',(69.2702879568036,71.3762149814349,202.750490121702));
#30464=CARTESIAN_POINT('',(69.2826628881893,71.396309438915,202.750490121702));
#30465=CARTESIAN_POINT('',(72.7737552404501,69.2463619539781,202.750490121702));
#30466=CARTESIAN_POINT('',(69.2826628881893,71.396309438915,202.750490121702));
#30467=CARTESIAN_POINT('',(72.7613803090644,69.2262674964981,202.750490121702));
#30468=CARTESIAN_POINT('',(72.7737552404501,69.2463619539781,202.750490121702));
#30469=CARTESIAN_POINT('Origin',(77.215862801455,80.368869783441,202.750490121702));
#30470=CARTESIAN_POINT('Origin',(72.7737552404501,69.2463619539781,192.750490121702));
#30471=CARTESIAN_POINT('',(72.7737552404501,69.2463619539781,196.17168857984));
#30472=CARTESIAN_POINT('',(71.699254778236,67.5015842920036,197.750490121702));
#30473=CARTESIAN_POINT('Ctrl Pts',(72.7737552404501,69.2463619539781,196.17168857984));
#30474=CARTESIAN_POINT('Ctrl Pts',(72.2783498325298,68.4419208953121,196.898024398673));
#30475=CARTESIAN_POINT('Ctrl Pts',(71.699254778236,67.5015842920036,197.750490121702));
#30476=CARTESIAN_POINT('',(71.699254778236,67.5015842920036,202.750490121702));
#30477=CARTESIAN_POINT('',(71.699254778236,67.5015842920036,202.950490121702));
#30478=CARTESIAN_POINT('',(72.7737552404501,69.2463619539781,202.750490121702));
#30479=CARTESIAN_POINT('',(72.7737552404501,69.2463619539781,192.750490121702));
#30480=CARTESIAN_POINT('Origin',(69.2826628881893,71.396309438915,192.750490121702));
#30481=CARTESIAN_POINT('',(69.2826628881893,71.396309438915,196.17168857984));
#30482=CARTESIAN_POINT('Ctrl Pts',(69.2826628881894,71.396309438915,196.17168857984));
#30483=CARTESIAN_POINT('Ctrl Pts',(71.0282090643197,70.3213356964465,195.897880393518));
#30484=CARTESIAN_POINT('Ctrl Pts',(72.7737552404501,69.2463619539781,196.17168857984));
#30485=CARTESIAN_POINT('',(69.2826628881893,71.396309438915,192.750490121702));
#30486=CARTESIAN_POINT('Origin',(69.2826628881893,71.396309438915,192.750490121702));
#30487=CARTESIAN_POINT('',(68.2081624259752,69.6515317769404,197.750490121702));
#30488=CARTESIAN_POINT('Ctrl Pts',(68.2081624259752,69.6515317769404,197.750490121702));
#30489=CARTESIAN_POINT('Ctrl Pts',(68.7872574802692,70.5918683802492,196.898024398673));
#30490=CARTESIAN_POINT('Ctrl Pts',(69.2826628881893,71.396309438915,196.17168857984));
#30491=CARTESIAN_POINT('',(68.2081624259752,69.6515317769404,202.750490121702));
#30492=CARTESIAN_POINT('',(69.2826628881893,71.396309438915,202.750490121702));
#30493=CARTESIAN_POINT('',(68.2081624259752,69.6515317769404,202.950490121702));
#30494=CARTESIAN_POINT('Origin',(77.215862801455,80.368869783441,202.750490121702));
#30495=CARTESIAN_POINT('',(68.2433024569292,88.3020696967067,202.750490121702));
#30496=CARTESIAN_POINT('',(68.223207999449,88.3144446280925,202.750490121702));
#30497=CARTESIAN_POINT('',(68.2433024569292,88.3020696967067,202.750490121702));
#30498=CARTESIAN_POINT('',(66.0933549719922,84.810977344446,202.750490121702));
#30499=CARTESIAN_POINT('',(68.2433024569292,88.3020696967067,202.750490121702));
#30500=CARTESIAN_POINT('',(66.0732605145121,84.8233522758317,202.750490121702));
#30501=CARTESIAN_POINT('',(66.0933549719922,84.810977344446,202.750490121702));
#30502=CARTESIAN_POINT('',(66.9980315265455,86.6613990076467,202.750490121702));
#30503=CARTESIAN_POINT('Origin',(77.215862801455,80.368869783441,202.750490121702));
#30504=CARTESIAN_POINT('Origin',(77.215862801455,80.368869783441,202.750490121702));
#30505=CARTESIAN_POINT('Origin',(66.0933549719922,84.810977344446,192.750490121702));
#30506=CARTESIAN_POINT('',(66.0933549719922,84.810977344446,196.17168857984));
#30507=CARTESIAN_POINT('',(64.3485773100176,85.8854778066601,197.750490121702));
#30508=CARTESIAN_POINT('Ctrl Pts',(66.0933549719923,84.810977344446,196.17168857984));
#30509=CARTESIAN_POINT('Ctrl Pts',(65.2889139133265,85.3063827523661,196.898024398673));
#30510=CARTESIAN_POINT('Ctrl Pts',(64.3485773100176,85.8854778066601,197.750490121702));
#30511=CARTESIAN_POINT('',(64.3485773100176,85.8854778066601,202.750490121702));
#30512=CARTESIAN_POINT('',(64.3485773100176,85.8854778066601,202.950490121702));
#30513=CARTESIAN_POINT('',(66.0933549719922,84.810977344446,202.750490121702));
#30514=CARTESIAN_POINT('',(66.0933549719922,84.810977344446,192.750490121702));
#30515=CARTESIAN_POINT('Origin',(68.2433024569292,88.3020696967067,192.750490121702));
#30516=CARTESIAN_POINT('',(68.2433024569292,88.3020696967067,196.17168857984));
#30517=CARTESIAN_POINT('',(67.1683287144608,86.5565235205765,196.033766787946));
#30518=CARTESIAN_POINT('Ctrl Pts',(68.2433024569291,88.3020696967066,196.17168857984));
#30519=CARTESIAN_POINT('Ctrl Pts',(67.7018200900497,87.42280870864,196.033766787946));
#30520=CARTESIAN_POINT('Ctrl Pts',(67.1683287144608,86.5565235205765,196.033766787946));
#30521=CARTESIAN_POINT('Ctrl Pts',(67.1683287144608,86.5565235205765,196.033766787946));
#30522=CARTESIAN_POINT('Ctrl Pts',(66.6348373388718,85.6902383325128,196.033766787946));
#30523=CARTESIAN_POINT('Ctrl Pts',(66.0933549719923,84.810977344446,196.17168857984));
#30524=CARTESIAN_POINT('',(68.2433024569292,88.3020696967067,192.750490121702));
#30525=CARTESIAN_POINT('Origin',(68.2433024569292,88.3020696967067,192.750490121702));
#30526=CARTESIAN_POINT('',(66.4985247949545,89.3765701589209,197.750490121702));
#30527=CARTESIAN_POINT('Ctrl Pts',(66.4985247949545,89.3765701589209,197.750490121702));
#30528=CARTESIAN_POINT('Ctrl Pts',(67.4388613982627,88.7974751046273,196.898024398674));
#30529=CARTESIAN_POINT('Ctrl Pts',(68.2433024569292,88.3020696967067,196.17168857984));
#30530=CARTESIAN_POINT('',(66.4985247949545,89.3765701589209,202.750490121702));
#30531=CARTESIAN_POINT('',(68.2433024569292,88.3020696967067,202.750490121702));
#30532=CARTESIAN_POINT('',(66.4985247949545,89.3765701589209,202.950490121702));
#30533=CARTESIAN_POINT('Origin',(77.215862801455,80.368869783441,202.950490121702));
#30534=CARTESIAN_POINT('Origin',(77.215862801455,80.368869783441,202.750490121702));
#30535=CARTESIAN_POINT('Origin',(77.215862801455,80.368869783441,197.750490121702));
#30536=CARTESIAN_POINT('Origin',(83.5083920256607,90.5867010583505,202.750490121702));
#30537=CARTESIAN_POINT('Origin',(77.215862801455,80.368869783441,202.750490121702));
#30538=CARTESIAN_POINT('Origin',(77.215862801455,80.368869783441,202.950490121702));
#30539=CARTESIAN_POINT('',(66.9980315265455,86.6613990076467,202.950490121702));
#30540=CARTESIAN_POINT('Origin',(77.215862801455,80.368869783441,202.950490121702));
#30541=CARTESIAN_POINT('',(66.9980315265455,86.6613990076467,202.950490121702));
#30542=CARTESIAN_POINT('Origin',(77.215862801455,80.368869783441,202.750490121702));
#30543=CARTESIAN_POINT('Origin',(77.215862801455,80.368869783441,202.750490121702));
#30544=CARTESIAN_POINT('Origin',(77.215862801455,80.368869783441,202.750490121702));
#30545=CARTESIAN_POINT('Origin',(81.4633200277938,87.2659058940049,202.950490121702));
#30546=CARTESIAN_POINT('Ctrl Pts',(68.8559951920602,81.9059493368123,202.950490121702));
#30547=CARTESIAN_POINT('Ctrl Pts',(68.7642152247191,81.2289065497019,202.950490121702));
#30548=CARTESIAN_POINT('Ctrl Pts',(68.7558437672831,80.5431690260287,202.950490121702));
#30549=CARTESIAN_POINT('Ctrl Pts',(68.9037765039421,79.208383788559,202.950490121702));
#30550=CARTESIAN_POINT('Ctrl Pts',(69.0539008969734,78.5636087221873,202.950490121702));
#30551=CARTESIAN_POINT('Ctrl Pts',(69.5077654228198,77.3091162265887,202.950490121702));
#30552=CARTESIAN_POINT('Ctrl Pts',(69.8131562970982,76.7051358769036,202.950490121702));
#30553=CARTESIAN_POINT('Ctrl Pts',(70.3807100616133,75.8558168618057,202.950490121702));
#30554=CARTESIAN_POINT('Ctrl Pts',(70.5846181218229,75.5896281769766,202.950490121702));
#30555=CARTESIAN_POINT('Ctrl Pts',(71.0222837417832,75.0866685278261,202.950490121702));
#30556=CARTESIAN_POINT('Ctrl Pts',(71.2518555252683,74.8532966906131,202.950490121702));
#30557=CARTESIAN_POINT('Ctrl Pts',(71.4950332612282,74.6345773796944,202.950490121702));
#30558=CARTESIAN_POINT('Ctrl Pts',(80.1444697952855,87.9209066660103,202.950490121702));
#30559=CARTESIAN_POINT('Ctrl Pts',(79.3727964197385,88.2659773938407,202.950490121702));
#30560=CARTESIAN_POINT('Ctrl Pts',(78.6856433791405,88.4271476868973,202.950490121702));
#30561=CARTESIAN_POINT('Ctrl Pts',(77.5319949492831,88.6233670935503,202.950490121702));
#30562=CARTESIAN_POINT('Ctrl Pts',(76.8660965396909,88.6557827059197,202.950490121702));
#30563=CARTESIAN_POINT('Ctrl Pts',(75.5487931964297,88.5618133194148,202.950490121702));
#30564=CARTESIAN_POINT('Ctrl Pts',(74.9019787775752,88.4376650266567,202.950490121702));
#30565=CARTESIAN_POINT('Ctrl Pts',(73.6122724742245,88.0273485574021,202.950490121702));
#30566=CARTESIAN_POINT('Ctrl Pts',(72.9824334762108,87.7347023571041,202.950490121702));
#30567=CARTESIAN_POINT('Ctrl Pts',(72.3914232244021,87.3670683207338,202.950490121702));
#30568=CARTESIAN_POINT('Origin',(77.215862801455,80.368869783441,202.950490121702));
#30569=CARTESIAN_POINT('',(70.3188266908911,84.6163270097798,195.150490121702));
#30570=CARTESIAN_POINT('Origin',(77.215862801455,80.368869783441,195.150490121702));
#30571=CARTESIAN_POINT('',(70.3188266908911,84.6163270097798,196.));
#30572=CARTESIAN_POINT('',(70.3188266908911,84.6163270097798,202.950490121702));
#30573=CARTESIAN_POINT('Origin',(77.215862801455,80.368869783441,196.));
#30574=CARTESIAN_POINT('Origin',(77.215862801455,80.368869783441,199.24883868241));
#30575=CARTESIAN_POINT('',(67.6632584598299,86.2517269543706,195.58019743297));
#30576=CARTESIAN_POINT('Origin',(77.215862801455,80.368869783441,195.58019743297));
#30577=CARTESIAN_POINT('Origin',(69.4466522947436,85.1534451837547,199.24883868241));
#30578=CARTESIAN_POINT('Origin',(77.215862801455,80.368869783441,197.750490121702));
#30579=CARTESIAN_POINT('Origin',(77.215862801455,80.368869783441,197.750490121702));
#30580=CARTESIAN_POINT('Origin',(77.215862801455,80.368869783441,197.750490121702));
#30581=CARTESIAN_POINT('',(65.295059647394,87.7101538783476,197.750490121702));
#30582=CARTESIAN_POINT('Origin',(77.215862801455,80.368869783441,197.750490121702));
#30583=CARTESIAN_POINT('Origin',(77.215862801455,80.368869783441,202.950490121702));
#30584=CARTESIAN_POINT('Origin',(77.215862801455,80.368869783441,202.750490121702));
#30585=CARTESIAN_POINT('Origin',(77.215862801455,80.368869783441,202.950490121702));
#30586=CARTESIAN_POINT('Origin',(77.215862801455,80.368869783441,202.750490121702));
#30587=CARTESIAN_POINT('Origin',(77.215862801455,80.368869783441,202.950490121702));
#30588=CARTESIAN_POINT('Origin',(77.215862801455,80.368869783441,202.750490121702));
#30589=CARTESIAN_POINT('Origin',(83.5083920256607,90.5867010583505,202.750490121702));
#30590=CARTESIAN_POINT('Origin',(83.5083920256607,90.5867010583505,202.750490121702));
#30591=CARTESIAN_POINT('Origin',(83.5083920256607,90.5867010583505,202.750490121702));
#30592=CARTESIAN_POINT('Ctrl Pts',(75.2070279073809,72.1096563878274,197.312500795565));
#30593=CARTESIAN_POINT('Ctrl Pts',(78.6281061103777,71.2775697301335,197.406250795565));
#30594=CARTESIAN_POINT('Ctrl Pts',(81.6355478248763,73.1082632082519,197.500000795565));
#30595=CARTESIAN_POINT('Ctrl Pts',(84.6429895393749,74.9389566863702,197.593750795565));
#30596=CARTESIAN_POINT('Ctrl Pts',(85.4750761970687,78.360034889367,197.687500795565));
#30597=CARTESIAN_POINT('Ctrl Pts',(86.3071628547625,81.7811130923637,197.781250795565));
#30598=CARTESIAN_POINT('Ctrl Pts',(84.4764693766442,84.7885548068623,197.875000795565));
#30599=CARTESIAN_POINT('Ctrl Pts',(82.6457758985258,87.7959965213609,197.968750795565));
#30600=CARTESIAN_POINT('Ctrl Pts',(79.2246976955291,88.6280831790547,198.062500795565));
#30601=CARTESIAN_POINT('Ctrl Pts',(75.8036194925323,89.4601698367485,198.156250795565));
#30602=CARTESIAN_POINT('Ctrl Pts',(72.7961777780337,87.6294763586302,198.250000795565));
#30603=CARTESIAN_POINT('Ctrl Pts',(69.7887360635351,85.7987828805119,198.343750795565));
#30604=CARTESIAN_POINT('Ctrl Pts',(68.9566494058413,82.3777046775151,198.437500795565));
#30605=CARTESIAN_POINT('Ctrl Pts',(68.1245627481475,78.9566264745184,198.531250795565));
#30606=CARTESIAN_POINT('Ctrl Pts',(69.9552562262659,75.9491847600198,198.625000795565));
#30607=CARTESIAN_POINT('Ctrl Pts',(71.7859497043842,72.9417430455211,198.718750795565));
#30608=CARTESIAN_POINT('Ctrl Pts',(75.2070279073809,72.1096563878274,198.812500795565));
#30609=CARTESIAN_POINT('Ctrl Pts',(78.6281061103777,71.2775697301335,198.906250795565));
#30610=CARTESIAN_POINT('Ctrl Pts',(81.6355478248763,73.1082632082519,199.000000795565));
#30611=CARTESIAN_POINT('Ctrl Pts',(84.6429895393749,74.9389566863702,199.093750795565));
#30612=CARTESIAN_POINT('Ctrl Pts',(85.4750761970687,78.360034889367,199.187500795565));
#30613=CARTESIAN_POINT('Ctrl Pts',(86.3071628547625,81.7811130923637,199.281250795565));
#30614=CARTESIAN_POINT('Ctrl Pts',(84.4764693766442,84.7885548068623,199.375000795565));
#30615=CARTESIAN_POINT('Ctrl Pts',(82.6457758985258,87.7959965213609,199.468750795565));
#30616=CARTESIAN_POINT('Ctrl Pts',(79.2246976955291,88.6280831790547,199.562500795565));
#30617=CARTESIAN_POINT('Ctrl Pts',(75.8036194925323,89.4601698367485,199.656250795565));
#30618=CARTESIAN_POINT('Ctrl Pts',(72.7961777780337,87.6294763586302,199.750000795565));
#30619=CARTESIAN_POINT('Ctrl Pts',(69.7887360635351,85.7987828805119,199.843750795565));
#30620=CARTESIAN_POINT('Ctrl Pts',(68.9566494058413,82.3777046775151,199.937500795565));
#30621=CARTESIAN_POINT('Ctrl Pts',(68.1245627481475,78.9566264745184,200.031250795565));
#30622=CARTESIAN_POINT('Ctrl Pts',(69.9552562262659,75.9491847600198,200.125000795565));
#30623=CARTESIAN_POINT('Ctrl Pts',(71.7859497043842,72.9417430455211,200.218750795565));
#30624=CARTESIAN_POINT('Ctrl Pts',(75.2070279073809,72.1096563878274,200.312500795565));
#30625=CARTESIAN_POINT('Ctrl Pts',(78.6281061103777,71.2775697301335,200.406250795565));
#30626=CARTESIAN_POINT('Ctrl Pts',(81.6355478248763,73.1082632082519,200.500000795565));
#30627=CARTESIAN_POINT('Ctrl Pts',(84.6429895393749,74.9389566863702,200.593750795565));
#30628=CARTESIAN_POINT('Ctrl Pts',(85.4750761970687,78.360034889367,200.687500795565));
#30629=CARTESIAN_POINT('Ctrl Pts',(86.3071628547625,81.7811130923637,200.781250795565));
#30630=CARTESIAN_POINT('Ctrl Pts',(84.4764693766442,84.7885548068623,200.875000795565));
#30631=CARTESIAN_POINT('Ctrl Pts',(82.6457758985258,87.7959965213609,200.968750795565));
#30632=CARTESIAN_POINT('Ctrl Pts',(79.2246976955291,88.6280831790547,201.062500795565));
#30633=CARTESIAN_POINT('Ctrl Pts',(75.8036194925323,89.4601698367485,201.156250795565));
#30634=CARTESIAN_POINT('Ctrl Pts',(72.7961777780337,87.6294763586302,201.250000795565));
#30635=CARTESIAN_POINT('Ctrl Pts',(69.7887360635351,85.7987828805119,201.343750795565));
#30636=CARTESIAN_POINT('Ctrl Pts',(68.9566494058413,82.3777046775151,201.437500795565));
#30637=CARTESIAN_POINT('Ctrl Pts',(68.1245627481475,78.9566264745183,201.531250795565));
#30638=CARTESIAN_POINT('Ctrl Pts',(69.9552562262659,75.9491847600198,201.625000795565));
#30639=CARTESIAN_POINT('Ctrl Pts',(71.7859497043842,72.9417430455211,201.718750795565));
#30640=CARTESIAN_POINT('Ctrl Pts',(75.2070279073809,72.1096563878273,201.812500795565));
#30641=CARTESIAN_POINT('Ctrl Pts',(78.6281061103777,71.2775697301335,201.906250795565));
#30642=CARTESIAN_POINT('Ctrl Pts',(81.6355478248763,73.1082632082519,202.000000795565));
#30643=CARTESIAN_POINT('Ctrl Pts',(84.6429895393749,74.9389566863702,202.093750795565));
#30644=CARTESIAN_POINT('Ctrl Pts',(85.4750761970687,78.360034889367,202.187500795565));
#30645=CARTESIAN_POINT('Ctrl Pts',(86.3071628547625,81.7811130923637,202.281250795565));
#30646=CARTESIAN_POINT('Ctrl Pts',(84.4764693766442,84.7885548068623,202.375000795565));
#30647=CARTESIAN_POINT('Ctrl Pts',(82.6457758985258,87.7959965213609,202.468750795565));
#30648=CARTESIAN_POINT('Ctrl Pts',(79.2246976955291,88.6280831790547,202.562500795565));
#30649=CARTESIAN_POINT('Ctrl Pts',(75.8036194925323,89.4601698367485,202.656250795565));
#30650=CARTESIAN_POINT('Ctrl Pts',(72.7961777780337,87.6294763586302,202.750000795565));
#30651=CARTESIAN_POINT('Ctrl Pts',(69.7887360635351,85.7987828805119,202.843750795565));
#30652=CARTESIAN_POINT('Ctrl Pts',(68.9566494058413,82.3777046775151,202.937500795565));
#30653=CARTESIAN_POINT('Ctrl Pts',(68.1245627481475,78.9566264745183,203.031250795565));
#30654=CARTESIAN_POINT('Ctrl Pts',(69.9552562262658,75.9491847600198,203.125000795565));
#30655=CARTESIAN_POINT('Ctrl Pts',(71.7859497043842,72.9417430455211,203.218750795565));
#30656=CARTESIAN_POINT('Ctrl Pts',(75.2070279073809,72.1096563878273,203.312500795565));
#30657=CARTESIAN_POINT('Ctrl Pts',(78.6281061103777,71.2775697301335,203.406250795565));
#30658=CARTESIAN_POINT('Ctrl Pts',(81.6355478248763,73.1082632082519,203.500000795565));
#30659=CARTESIAN_POINT('Ctrl Pts',(84.6429895393749,74.9389566863702,203.593750795565));
#30660=CARTESIAN_POINT('Ctrl Pts',(85.4750761970687,78.360034889367,203.687500795565));
#30661=CARTESIAN_POINT('Ctrl Pts',(86.3071628547625,81.7811130923637,203.781250795565));
#30662=CARTESIAN_POINT('Ctrl Pts',(84.4764693766442,84.7885548068623,203.875000795565));
#30663=CARTESIAN_POINT('Ctrl Pts',(82.6457758985258,87.7959965213609,203.968750795565));
#30664=CARTESIAN_POINT('Ctrl Pts',(79.2246976955291,88.6280831790547,204.062500795565));
#30665=CARTESIAN_POINT('Ctrl Pts',(75.8036194925323,89.4601698367485,204.156250795565));
#30666=CARTESIAN_POINT('Ctrl Pts',(72.7961777780337,87.6294763586302,204.250000795565));
#30667=CARTESIAN_POINT('Ctrl Pts',(69.7887360635351,85.7987828805118,204.343750795565));
#30668=CARTESIAN_POINT('Ctrl Pts',(68.9566494058413,82.3777046775151,204.437500795565));
#30669=CARTESIAN_POINT('Ctrl Pts',(68.1245627481475,78.9566264745183,204.531250795565));
#30670=CARTESIAN_POINT('Ctrl Pts',(69.9552562262658,75.9491847600198,204.625000795565));
#30671=CARTESIAN_POINT('Ctrl Pts',(71.7859497043842,72.9417430455211,204.718750795565));
#30672=CARTESIAN_POINT('Ctrl Pts',(75.2070279073809,72.1096563878273,204.812500795565));
#30673=CARTESIAN_POINT('Ctrl Pts',(78.6281061103777,71.2775697301335,204.906250795565));
#30674=CARTESIAN_POINT('Ctrl Pts',(81.6355478248763,73.1082632082519,205.000000795565));
#30675=CARTESIAN_POINT('Ctrl Pts',(84.6429895393749,74.9389566863702,205.093750795565));
#30676=CARTESIAN_POINT('Ctrl Pts',(85.4750761970687,78.360034889367,205.187500795565));
#30677=CARTESIAN_POINT('Ctrl Pts',(86.3071628547625,81.7811130923637,205.281250795565));
#30678=CARTESIAN_POINT('Ctrl Pts',(84.4764693766442,84.7885548068623,205.375000795565));
#30679=CARTESIAN_POINT('Ctrl Pts',(82.6457758985258,87.7959965213609,205.468750795565));
#30680=CARTESIAN_POINT('Ctrl Pts',(79.2246976955291,88.6280831790547,205.562500795565));
#30681=CARTESIAN_POINT('Ctrl Pts',(75.8036194925323,89.4601698367485,205.656250795565));
#30682=CARTESIAN_POINT('Ctrl Pts',(72.7961777780337,87.6294763586302,205.750000795565));
#30683=CARTESIAN_POINT('Ctrl Pts',(69.7887360635351,85.7987828805118,205.843750795565));
#30684=CARTESIAN_POINT('Ctrl Pts',(68.9566494058413,82.3777046775151,205.937500795565));
#30685=CARTESIAN_POINT('Ctrl Pts',(68.1245627481475,78.9566264745183,206.031250795565));
#30686=CARTESIAN_POINT('Ctrl Pts',(69.9552562262658,75.9491847600198,206.125000795565));
#30687=CARTESIAN_POINT('Ctrl Pts',(71.7859497043842,72.9417430455211,206.218750795565));
#30688=CARTESIAN_POINT('Ctrl Pts',(75.2070279073809,72.1096563878273,206.312500795565));
#30689=CARTESIAN_POINT('Ctrl Pts',(78.6281061103777,71.2775697301335,206.406250795565));
#30690=CARTESIAN_POINT('Ctrl Pts',(81.6355478248763,73.1082632082519,206.500000795565));
#30691=CARTESIAN_POINT('Ctrl Pts',(84.6429895393749,74.9389566863702,206.593750795565));
#30692=CARTESIAN_POINT('Ctrl Pts',(85.4750761970687,78.3600348893669,206.687500795565));
#30693=CARTESIAN_POINT('Ctrl Pts',(86.3071628547625,81.7811130923637,206.781250795565));
#30694=CARTESIAN_POINT('Ctrl Pts',(84.4764693766442,84.7885548068623,206.875000795565));
#30695=CARTESIAN_POINT('Ctrl Pts',(82.6457758985258,87.7959965213609,206.968750795565));
#30696=CARTESIAN_POINT('Ctrl Pts',(79.2246976955291,88.6280831790547,207.062500795565));
#30697=CARTESIAN_POINT('Ctrl Pts',(75.8036194925323,89.4601698367485,207.156250795565));
#30698=CARTESIAN_POINT('Ctrl Pts',(72.7961777780337,87.6294763586302,207.250000795565));
#30699=CARTESIAN_POINT('Ctrl Pts',(69.7887360635351,85.7987828805118,207.343750795565));
#30700=CARTESIAN_POINT('Ctrl Pts',(68.9566494058413,82.3777046775151,207.437500795565));
#30701=CARTESIAN_POINT('Ctrl Pts',(68.1245627481475,78.9566264745183,207.531250795565));
#30702=CARTESIAN_POINT('Ctrl Pts',(69.9552562262658,75.9491847600198,207.625000795565));
#30703=CARTESIAN_POINT('Ctrl Pts',(71.7859497043842,72.9417430455211,207.718750795565));
#30704=CARTESIAN_POINT('Ctrl Pts',(75.2070279073809,72.1096563878273,207.812500795565));
#30705=CARTESIAN_POINT('Ctrl Pts',(78.6281061103777,71.2775697301335,207.906250795565));
#30706=CARTESIAN_POINT('Ctrl Pts',(81.6355478248763,73.1082632082518,208.000000795565));
#30707=CARTESIAN_POINT('Ctrl Pts',(84.6429895393749,74.9389566863702,208.093750795565));
#30708=CARTESIAN_POINT('Ctrl Pts',(85.4750761970687,78.3600348893669,208.187500795565));
#30709=CARTESIAN_POINT('Ctrl Pts',(86.3071628547625,81.7811130923637,208.281250795565));
#30710=CARTESIAN_POINT('Ctrl Pts',(84.4764693766442,84.7885548068623,208.375000795565));
#30711=CARTESIAN_POINT('Ctrl Pts',(82.6457758985258,87.7959965213609,208.468750795565));
#30712=CARTESIAN_POINT('Ctrl Pts',(79.2246976955291,88.6280831790547,208.562500795565));
#30713=CARTESIAN_POINT('Ctrl Pts',(75.8036194925323,89.4601698367485,208.656250795565));
#30714=CARTESIAN_POINT('Ctrl Pts',(72.7961777780337,87.6294763586302,208.750000795565));
#30715=CARTESIAN_POINT('Ctrl Pts',(69.7887360635351,85.7987828805118,208.843750795565));
#30716=CARTESIAN_POINT('Ctrl Pts',(68.9566494058413,82.3777046775151,208.937500795565));
#30717=CARTESIAN_POINT('Ctrl Pts',(68.1245627481475,78.9566264745183,209.031250795565));
#30718=CARTESIAN_POINT('Ctrl Pts',(69.9552562262658,75.9491847600198,209.125000795565));
#30719=CARTESIAN_POINT('Ctrl Pts',(71.7859497043842,72.9417430455211,209.218750795565));
#30720=CARTESIAN_POINT('Ctrl Pts',(75.2070279073809,72.1096563878273,209.312500795565));
#30721=CARTESIAN_POINT('Ctrl Pts',(75.3989071052151,72.8985570813421,196.843749997952));
#30722=CARTESIAN_POINT('Ctrl Pts',(78.4932119415925,72.1459493897285,196.937499997952));
#30723=CARTESIAN_POINT('Ctrl Pts',(81.2133898767664,73.8017793202762,197.031249997952));
#30724=CARTESIAN_POINT('Ctrl Pts',(83.9335678119403,75.4576092508238,197.124999997952));
#30725=CARTESIAN_POINT('Ctrl Pts',(84.6861755035539,78.5519140872012,197.218749997952));
#30726=CARTESIAN_POINT('Ctrl Pts',(85.4387831951675,81.6462189235785,197.312499997952));
#30727=CARTESIAN_POINT('Ctrl Pts',(83.7829532646199,84.3663968587524,197.406249997952));
#30728=CARTESIAN_POINT('Ctrl Pts',(82.1271233340723,87.0865747939263,197.499999997952));
#30729=CARTESIAN_POINT('Ctrl Pts',(79.0328184976949,87.83918248554,197.593749997952));
#30730=CARTESIAN_POINT('Ctrl Pts',(75.9385136613175,88.5917901771536,197.687499997952));
#30731=CARTESIAN_POINT('Ctrl Pts',(73.2183357261436,86.9359602466059,197.781249997952));
#30732=CARTESIAN_POINT('Ctrl Pts',(70.4981577909697,85.2801303160583,197.874999997952));
#30733=CARTESIAN_POINT('Ctrl Pts',(69.7455500993561,82.1858254796809,197.968749997952));
#30734=CARTESIAN_POINT('Ctrl Pts',(68.9929424077425,79.0915206433035,198.062499997952));
#30735=CARTESIAN_POINT('Ctrl Pts',(70.6487723382901,76.3713427081296,198.156249997952));
#30736=CARTESIAN_POINT('Ctrl Pts',(72.3046022688378,73.6511647729557,198.249999997952));
#30737=CARTESIAN_POINT('Ctrl Pts',(75.3989071052151,72.8985570813421,198.343749997952));
#30738=CARTESIAN_POINT('Ctrl Pts',(78.4932119415925,72.1459493897285,198.437499997952));
#30739=CARTESIAN_POINT('Ctrl Pts',(81.2133898767664,73.8017793202762,198.531249997952));
#30740=CARTESIAN_POINT('Ctrl Pts',(83.9335678119403,75.4576092508238,198.624999997952));
#30741=CARTESIAN_POINT('Ctrl Pts',(84.6861755035539,78.5519140872012,198.718749997952));
#30742=CARTESIAN_POINT('Ctrl Pts',(85.4387831951675,81.6462189235785,198.812499997952));
#30743=CARTESIAN_POINT('Ctrl Pts',(83.7829532646199,84.3663968587524,198.906249997952));
#30744=CARTESIAN_POINT('Ctrl Pts',(82.1271233340723,87.0865747939263,198.999999997952));
#30745=CARTESIAN_POINT('Ctrl Pts',(79.0328184976949,87.8391824855399,199.093749997952));
#30746=CARTESIAN_POINT('Ctrl Pts',(75.9385136613175,88.5917901771536,199.187499997952));
#30747=CARTESIAN_POINT('Ctrl Pts',(73.2183357261436,86.9359602466059,199.281249997952));
#30748=CARTESIAN_POINT('Ctrl Pts',(70.4981577909697,85.2801303160583,199.374999997952));
#30749=CARTESIAN_POINT('Ctrl Pts',(69.7455500993561,82.1858254796809,199.468749997952));
#30750=CARTESIAN_POINT('Ctrl Pts',(68.9929424077425,79.0915206433035,199.562499997952));
#30751=CARTESIAN_POINT('Ctrl Pts',(70.6487723382901,76.3713427081296,199.656249997952));
#30752=CARTESIAN_POINT('Ctrl Pts',(72.3046022688378,73.6511647729557,199.749999997952));
#30753=CARTESIAN_POINT('Ctrl Pts',(75.3989071052151,72.8985570813421,199.843749997952));
#30754=CARTESIAN_POINT('Ctrl Pts',(78.4932119415925,72.1459493897285,199.937499997952));
#30755=CARTESIAN_POINT('Ctrl Pts',(81.2133898767664,73.8017793202761,200.031249997952));
#30756=CARTESIAN_POINT('Ctrl Pts',(83.9335678119403,75.4576092508238,200.124999997952));
#30757=CARTESIAN_POINT('Ctrl Pts',(84.6861755035539,78.5519140872012,200.218749997952));
#30758=CARTESIAN_POINT('Ctrl Pts',(85.4387831951675,81.6462189235785,200.312499997952));
#30759=CARTESIAN_POINT('Ctrl Pts',(83.7829532646199,84.3663968587524,200.406249997952));
#30760=CARTESIAN_POINT('Ctrl Pts',(82.1271233340723,87.0865747939263,200.499999997952));
#30761=CARTESIAN_POINT('Ctrl Pts',(79.0328184976949,87.8391824855399,200.593749997952));
#30762=CARTESIAN_POINT('Ctrl Pts',(75.9385136613175,88.5917901771536,200.687499997952));
#30763=CARTESIAN_POINT('Ctrl Pts',(73.2183357261436,86.9359602466059,200.781249997952));
#30764=CARTESIAN_POINT('Ctrl Pts',(70.4981577909697,85.2801303160583,200.874999997952));
#30765=CARTESIAN_POINT('Ctrl Pts',(69.7455500993561,82.1858254796809,200.968749997952));
#30766=CARTESIAN_POINT('Ctrl Pts',(68.9929424077425,79.0915206433035,201.062499997952));
#30767=CARTESIAN_POINT('Ctrl Pts',(70.6487723382901,76.3713427081296,201.156249997952));
#30768=CARTESIAN_POINT('Ctrl Pts',(72.3046022688378,73.6511647729557,201.249999997952));
#30769=CARTESIAN_POINT('Ctrl Pts',(75.3989071052151,72.8985570813421,201.343749997952));
#30770=CARTESIAN_POINT('Ctrl Pts',(78.4932119415925,72.1459493897285,201.437499997952));
#30771=CARTESIAN_POINT('Ctrl Pts',(81.2133898767664,73.8017793202761,201.531249997952));
#30772=CARTESIAN_POINT('Ctrl Pts',(83.9335678119403,75.4576092508238,201.624999997952));
#30773=CARTESIAN_POINT('Ctrl Pts',(84.6861755035539,78.5519140872011,201.718749997952));
#30774=CARTESIAN_POINT('Ctrl Pts',(85.4387831951675,81.6462189235785,201.812499997952));
#30775=CARTESIAN_POINT('Ctrl Pts',(83.7829532646199,84.3663968587524,201.906249997952));
#30776=CARTESIAN_POINT('Ctrl Pts',(82.1271233340723,87.0865747939263,201.999999997952));
#30777=CARTESIAN_POINT('Ctrl Pts',(79.0328184976949,87.8391824855399,202.093749997952));
#30778=CARTESIAN_POINT('Ctrl Pts',(75.9385136613175,88.5917901771535,202.187499997952));
#30779=CARTESIAN_POINT('Ctrl Pts',(73.2183357261436,86.9359602466059,202.281249997952));
#30780=CARTESIAN_POINT('Ctrl Pts',(70.4981577909697,85.2801303160583,202.374999997952));
#30781=CARTESIAN_POINT('Ctrl Pts',(69.7455500993561,82.1858254796809,202.468749997952));
#30782=CARTESIAN_POINT('Ctrl Pts',(68.9929424077425,79.0915206433035,202.562499997952));
#30783=CARTESIAN_POINT('Ctrl Pts',(70.6487723382901,76.3713427081296,202.656249997952));
#30784=CARTESIAN_POINT('Ctrl Pts',(72.3046022688378,73.6511647729557,202.749999997952));
#30785=CARTESIAN_POINT('Ctrl Pts',(75.3989071052151,72.8985570813421,202.843749997952));
#30786=CARTESIAN_POINT('Ctrl Pts',(78.4932119415925,72.1459493897285,202.937499997952));
#30787=CARTESIAN_POINT('Ctrl Pts',(81.2133898767664,73.8017793202761,203.031249997952));
#30788=CARTESIAN_POINT('Ctrl Pts',(83.9335678119403,75.4576092508238,203.124999997952));
#30789=CARTESIAN_POINT('Ctrl Pts',(84.6861755035539,78.5519140872011,203.218749997952));
#30790=CARTESIAN_POINT('Ctrl Pts',(85.4387831951675,81.6462189235785,203.312499997952));
#30791=CARTESIAN_POINT('Ctrl Pts',(83.7829532646199,84.3663968587524,203.406249997952));
#30792=CARTESIAN_POINT('Ctrl Pts',(82.1271233340723,87.0865747939263,203.499999997952));
#30793=CARTESIAN_POINT('Ctrl Pts',(79.0328184976949,87.8391824855399,203.593749997952));
#30794=CARTESIAN_POINT('Ctrl Pts',(75.9385136613175,88.5917901771535,203.687499997952));
#30795=CARTESIAN_POINT('Ctrl Pts',(73.2183357261436,86.9359602466059,203.781249997952));
#30796=CARTESIAN_POINT('Ctrl Pts',(70.4981577909697,85.2801303160583,203.874999997952));
#30797=CARTESIAN_POINT('Ctrl Pts',(69.7455500993561,82.1858254796809,203.968749997952));
#30798=CARTESIAN_POINT('Ctrl Pts',(68.9929424077425,79.0915206433035,204.062499997952));
#30799=CARTESIAN_POINT('Ctrl Pts',(70.6487723382901,76.3713427081296,204.156249997952));
#30800=CARTESIAN_POINT('Ctrl Pts',(72.3046022688378,73.6511647729557,204.249999997952));
#30801=CARTESIAN_POINT('Ctrl Pts',(75.3989071052151,72.8985570813421,204.343749997952));
#30802=CARTESIAN_POINT('Ctrl Pts',(78.4932119415925,72.1459493897285,204.437499997952));
#30803=CARTESIAN_POINT('Ctrl Pts',(81.2133898767664,73.8017793202761,204.531249997952));
#30804=CARTESIAN_POINT('Ctrl Pts',(83.9335678119403,75.4576092508238,204.624999997952));
#30805=CARTESIAN_POINT('Ctrl Pts',(84.6861755035539,78.5519140872011,204.718749997952));
#30806=CARTESIAN_POINT('Ctrl Pts',(85.4387831951675,81.6462189235785,204.812499997952));
#30807=CARTESIAN_POINT('Ctrl Pts',(83.7829532646199,84.3663968587524,204.906249997952));
#30808=CARTESIAN_POINT('Ctrl Pts',(82.1271233340722,87.0865747939263,204.999999997952));
#30809=CARTESIAN_POINT('Ctrl Pts',(79.0328184976949,87.8391824855399,205.093749997952));
#30810=CARTESIAN_POINT('Ctrl Pts',(75.9385136613175,88.5917901771535,205.187499997952));
#30811=CARTESIAN_POINT('Ctrl Pts',(73.2183357261436,86.9359602466059,205.281249997952));
#30812=CARTESIAN_POINT('Ctrl Pts',(70.4981577909697,85.2801303160583,205.374999997952));
#30813=CARTESIAN_POINT('Ctrl Pts',(69.7455500993561,82.1858254796809,205.468749997952));
#30814=CARTESIAN_POINT('Ctrl Pts',(68.9929424077425,79.0915206433035,205.562499997952));
#30815=CARTESIAN_POINT('Ctrl Pts',(70.6487723382901,76.3713427081296,205.656249997952));
#30816=CARTESIAN_POINT('Ctrl Pts',(72.3046022688378,73.6511647729557,205.749999997952));
#30817=CARTESIAN_POINT('Ctrl Pts',(75.3989071052151,72.8985570813421,205.843749997952));
#30818=CARTESIAN_POINT('Ctrl Pts',(78.4932119415925,72.1459493897285,205.937499997952));
#30819=CARTESIAN_POINT('Ctrl Pts',(81.2133898767664,73.8017793202761,206.031249997952));
#30820=CARTESIAN_POINT('Ctrl Pts',(83.9335678119403,75.4576092508238,206.124999997952));
#30821=CARTESIAN_POINT('Ctrl Pts',(84.6861755035539,78.5519140872011,206.218749997952));
#30822=CARTESIAN_POINT('Ctrl Pts',(85.4387831951675,81.6462189235785,206.312499997952));
#30823=CARTESIAN_POINT('Ctrl Pts',(83.7829532646199,84.3663968587524,206.406249997952));
#30824=CARTESIAN_POINT('Ctrl Pts',(82.1271233340722,87.0865747939263,206.499999997952));
#30825=CARTESIAN_POINT('Ctrl Pts',(79.0328184976949,87.8391824855399,206.593749997952));
#30826=CARTESIAN_POINT('Ctrl Pts',(75.9385136613175,88.5917901771535,206.687499997952));
#30827=CARTESIAN_POINT('Ctrl Pts',(73.2183357261436,86.9359602466059,206.781249997952));
#30828=CARTESIAN_POINT('Ctrl Pts',(70.4981577909697,85.2801303160583,206.874999997952));
#30829=CARTESIAN_POINT('Ctrl Pts',(69.7455500993561,82.1858254796809,206.968749997952));
#30830=CARTESIAN_POINT('Ctrl Pts',(68.9929424077425,79.0915206433035,207.062499997952));
#30831=CARTESIAN_POINT('Ctrl Pts',(70.6487723382901,76.3713427081296,207.156249997952));
#30832=CARTESIAN_POINT('Ctrl Pts',(72.3046022688378,73.6511647729557,207.249999997952));
#30833=CARTESIAN_POINT('Ctrl Pts',(75.3989071052151,72.8985570813421,207.343749997952));
#30834=CARTESIAN_POINT('Ctrl Pts',(78.4932119415925,72.1459493897285,207.437499997952));
#30835=CARTESIAN_POINT('Ctrl Pts',(81.2133898767664,73.8017793202761,207.531249997952));
#30836=CARTESIAN_POINT('Ctrl Pts',(83.9335678119403,75.4576092508238,207.624999997952));
#30837=CARTESIAN_POINT('Ctrl Pts',(84.6861755035539,78.5519140872011,207.718749997952));
#30838=CARTESIAN_POINT('Ctrl Pts',(85.4387831951675,81.6462189235785,207.812499997952));
#30839=CARTESIAN_POINT('Ctrl Pts',(83.7829532646199,84.3663968587524,207.906249997952));
#30840=CARTESIAN_POINT('Ctrl Pts',(82.1271233340722,87.0865747939263,207.999999997952));
#30841=CARTESIAN_POINT('Ctrl Pts',(79.0328184976949,87.8391824855399,208.093749997952));
#30842=CARTESIAN_POINT('Ctrl Pts',(75.9385136613175,88.5917901771535,208.187499997952));
#30843=CARTESIAN_POINT('Ctrl Pts',(73.2183357261436,86.9359602466059,208.281249997952));
#30844=CARTESIAN_POINT('Ctrl Pts',(70.4981577909697,85.2801303160583,208.374999997952));
#30845=CARTESIAN_POINT('Ctrl Pts',(69.7455500993561,82.1858254796809,208.468749997952));
#30846=CARTESIAN_POINT('Ctrl Pts',(68.9929424077425,79.0915206433035,208.562499997952));
#30847=CARTESIAN_POINT('Ctrl Pts',(70.6487723382901,76.3713427081296,208.656249997952));
#30848=CARTESIAN_POINT('Ctrl Pts',(72.3046022688377,73.6511647729557,208.749999997952));
#30849=CARTESIAN_POINT('Ctrl Pts',(75.3989071052151,72.8985570813421,208.843749997952));
#30850=CARTESIAN_POINT('',(75.3989071052151,72.8985570813421,196.843749997952));
#30851=CARTESIAN_POINT('',(75.3029676699654,72.5041074074942,197.078124996927));
#30852=CARTESIAN_POINT('Ctrl Pts',(75.3989071052151,72.8985570813421,196.843749997952));
#30853=CARTESIAN_POINT('Ctrl Pts',(78.4932119415925,72.1459493897285,196.937499997952));
#30854=CARTESIAN_POINT('Ctrl Pts',(81.2133898767664,73.8017793202762,197.031249997952));
#30855=CARTESIAN_POINT('Ctrl Pts',(83.9335678119403,75.4576092508238,197.124999997952));
#30856=CARTESIAN_POINT('Ctrl Pts',(84.6861755035539,78.5519140872012,197.218749997952));
#30857=CARTESIAN_POINT('Ctrl Pts',(85.4387831951675,81.6462189235786,197.312499997952));
#30858=CARTESIAN_POINT('Ctrl Pts',(83.7829532646199,84.3663968587524,197.406249997952));
#30859=CARTESIAN_POINT('Ctrl Pts',(82.1271233340723,87.0865747939263,197.499999997952));
#30860=CARTESIAN_POINT('Ctrl Pts',(79.0328184976949,87.83918248554,197.593749997952));
#30861=CARTESIAN_POINT('',(75.2070282347158,72.1096577336463,209.312499995903));
#30862=CARTESIAN_POINT('',(75.3029676699654,72.5041074074942,209.078124996927));
#30863=CARTESIAN_POINT('',(81.6355472361212,73.1082644713496,208.));
#30864=CARTESIAN_POINT('Ctrl Pts',(81.6355472361214,73.1082644713497,208.));
#30865=CARTESIAN_POINT('Ctrl Pts',(84.6429883504424,74.9389576587352,208.093749998303));
#30866=CARTESIAN_POINT('Ctrl Pts',(85.4750748512497,78.3600352167018,208.187499995903));
#30867=CARTESIAN_POINT('Ctrl Pts',(86.3071613733569,81.781112862242,208.281249995903));
#30868=CARTESIAN_POINT('Ctrl Pts',(84.4764681935457,84.7885540866852,208.374999995903));
#30869=CARTESIAN_POINT('Ctrl Pts',(82.6457750137345,87.7959953111284,208.468749995903));
#30870=CARTESIAN_POINT('Ctrl Pts',(79.2246973681942,88.6280818332357,208.562499995903));
#30871=CARTESIAN_POINT('Ctrl Pts',(75.803619722654,89.460168355343,208.656249995903));
#30872=CARTESIAN_POINT('Ctrl Pts',(72.7961784982108,87.6294751755317,208.749999995903));
#30873=CARTESIAN_POINT('Ctrl Pts',(69.7887372737676,85.7987819957205,208.843749995903));
#30874=CARTESIAN_POINT('Ctrl Pts',(68.9566507516603,82.3777043501803,208.937499995903));
#30875=CARTESIAN_POINT('Ctrl Pts',(68.124564229553,78.95662670464,209.031249995903));
#30876=CARTESIAN_POINT('Ctrl Pts',(69.9552574093643,75.9491854801968,209.124999995903));
#30877=CARTESIAN_POINT('Ctrl Pts',(71.7859505891755,72.9417442557536,209.218749995903));
#30878=CARTESIAN_POINT('Ctrl Pts',(75.2070282347158,72.1096577336463,209.312499995903));
#30879=CARTESIAN_POINT('Ctrl Pts',(81.6355472361212,73.1082644713497,208.));
#30880=CARTESIAN_POINT('Ctrl Pts',(80.8763023374092,72.6460959996179,207.976332302027));
#30881=CARTESIAN_POINT('Ctrl Pts',(80.0492000646897,72.3058399894939,207.951271393806));
#30882=CARTESIAN_POINT('Ctrl Pts',(78.3088074180245,71.8915116109437,207.899872573309));
#30883=CARTESIAN_POINT('Ctrl Pts',(77.4056191879471,71.8234526459273,207.87384897067));
#30884=CARTESIAN_POINT('Ctrl Pts',(75.4144643689082,71.9896960664897,207.81787699499));
#30885=CARTESIAN_POINT('Ctrl Pts',(74.3483000261168,72.2921953447178,207.789415502797));
#30886=CARTESIAN_POINT('Ctrl Pts',(72.3787421826247,73.2917323325248,207.726588879605));
#30887=CARTESIAN_POINT('Ctrl Pts',(71.4963547690888,73.9836631758121,207.694289190011));
#30888=CARTESIAN_POINT('Ctrl Pts',(70.0567962100578,75.6571168902924,207.632330501293));
#30889=CARTESIAN_POINT('Ctrl Pts',(69.5092102801739,76.619155890067,207.603946128111));
#30890=CARTESIAN_POINT('Ctrl Pts',(68.8050736208812,78.712263806775,207.541219969294));
#30891=CARTESIAN_POINT('Ctrl Pts',(68.6607351367236,79.8252454036478,207.508884056451));
#30892=CARTESIAN_POINT('Ctrl Pts',(68.8075917415253,82.0275556159198,207.446812675813));
#30893=CARTESIAN_POINT('Ctrl Pts',(69.0911351356286,83.0963336594984,207.418492485847));
#30894=CARTESIAN_POINT('Ctrl Pts',(70.0557013989788,85.0826730046347,207.355870265652));
#30895=CARTESIAN_POINT('Ctrl Pts',(70.7335105098385,85.9784128363935,207.32350012221));
#30896=CARTESIAN_POINT('Ctrl Pts',(72.3821140895016,87.4457835655045,207.261317041861));
#30897=CARTESIAN_POINT('Ctrl Pts',(73.3325145913956,88.0087284623981,207.233047488343));
#30898=CARTESIAN_POINT('Ctrl Pts',(75.4124942858855,88.7496733152931,207.170532376289));
#30899=CARTESIAN_POINT('Ctrl Pts',(76.524761081961,88.9135985745502,207.138130168159));
#30900=CARTESIAN_POINT('Ctrl Pts',(78.1735146408528,88.8318190807521,207.091535997759));
#30901=CARTESIAN_POINT('Ctrl Pts',(78.7050820316669,88.7544645006295,207.07673935053));
#30902=CARTESIAN_POINT('Ctrl Pts',(79.2246973681942,88.6280818332357,207.062499995903));
#30903=CARTESIAN_POINT('Ctrl Pts',(75.3989071052151,72.8985570813421,196.468749997952));
#30904=CARTESIAN_POINT('Ctrl Pts',(78.4932119415925,72.1459493897285,196.562499997952));
#30905=CARTESIAN_POINT('Ctrl Pts',(81.2133898767664,73.8017793202762,196.656249997952));
#30906=CARTESIAN_POINT('Ctrl Pts',(83.9335678119403,75.4576092508238,196.749999997952));
#30907=CARTESIAN_POINT('Ctrl Pts',(84.6861755035539,78.5519140872012,196.843749997952));
#30908=CARTESIAN_POINT('Ctrl Pts',(85.4387831951675,81.6462189235785,196.937499997952));
#30909=CARTESIAN_POINT('Ctrl Pts',(83.7829532646199,84.3663968587524,197.031249997952));
#30910=CARTESIAN_POINT('Ctrl Pts',(82.1271233340723,87.0865747939263,197.124999997952));
#30911=CARTESIAN_POINT('Ctrl Pts',(79.0328184976949,87.83918248554,197.218749997952));
#30912=CARTESIAN_POINT('Ctrl Pts',(75.9385136613175,88.5917901771536,197.312499997952));
#30913=CARTESIAN_POINT('Ctrl Pts',(73.2183357261436,86.9359602466059,197.406249997952));
#30914=CARTESIAN_POINT('Ctrl Pts',(70.4981577909697,85.2801303160583,197.499999997952));
#30915=CARTESIAN_POINT('Ctrl Pts',(69.7455500993561,82.1858254796809,197.593749997952));
#30916=CARTESIAN_POINT('Ctrl Pts',(68.9929424077425,79.0915206433035,197.687499997952));
#30917=CARTESIAN_POINT('Ctrl Pts',(70.6487723382901,76.3713427081296,197.781249997952));
#30918=CARTESIAN_POINT('Ctrl Pts',(72.3046022688378,73.6511647729557,197.874999997952));
#30919=CARTESIAN_POINT('Ctrl Pts',(75.3989071052151,72.8985570813421,197.968749997952));
#30920=CARTESIAN_POINT('Ctrl Pts',(78.4932119415925,72.1459493897285,198.062499997952));
#30921=CARTESIAN_POINT('Ctrl Pts',(81.2133898767664,73.8017793202762,198.156249997952));
#30922=CARTESIAN_POINT('Ctrl Pts',(83.9335678119403,75.4576092508238,198.249999997952));
#30923=CARTESIAN_POINT('Ctrl Pts',(84.6861755035539,78.5519140872012,198.343749997952));
#30924=CARTESIAN_POINT('Ctrl Pts',(85.4387831951675,81.6462189235785,198.437499997952));
#30925=CARTESIAN_POINT('Ctrl Pts',(83.7829532646199,84.3663968587524,198.531249997952));
#30926=CARTESIAN_POINT('Ctrl Pts',(82.1271233340723,87.0865747939263,198.624999997952));
#30927=CARTESIAN_POINT('Ctrl Pts',(79.0328184976949,87.8391824855399,198.718749997952));
#30928=CARTESIAN_POINT('Ctrl Pts',(75.9385136613175,88.5917901771536,198.812499997952));
#30929=CARTESIAN_POINT('Ctrl Pts',(73.2183357261436,86.9359602466059,198.906249997952));
#30930=CARTESIAN_POINT('Ctrl Pts',(70.4981577909697,85.2801303160583,198.999999997952));
#30931=CARTESIAN_POINT('Ctrl Pts',(69.7455500993561,82.1858254796809,199.093749997952));
#30932=CARTESIAN_POINT('Ctrl Pts',(68.9929424077425,79.0915206433035,199.187499997952));
#30933=CARTESIAN_POINT('Ctrl Pts',(70.6487723382901,76.3713427081296,199.281249997952));
#30934=CARTESIAN_POINT('Ctrl Pts',(72.3046022688378,73.6511647729557,199.374999997952));
#30935=CARTESIAN_POINT('Ctrl Pts',(75.3989071052151,72.8985570813421,199.468749997952));
#30936=CARTESIAN_POINT('Ctrl Pts',(78.4932119415925,72.1459493897285,199.562499997952));
#30937=CARTESIAN_POINT('Ctrl Pts',(81.2133898767664,73.8017793202761,199.656249997952));
#30938=CARTESIAN_POINT('Ctrl Pts',(83.9335678119403,75.4576092508238,199.749999997952));
#30939=CARTESIAN_POINT('Ctrl Pts',(84.6861755035539,78.5519140872012,199.843749997952));
#30940=CARTESIAN_POINT('Ctrl Pts',(85.4387831951675,81.6462189235785,199.937499997952));
#30941=CARTESIAN_POINT('Ctrl Pts',(83.7829532646199,84.3663968587524,200.031249997952));
#30942=CARTESIAN_POINT('Ctrl Pts',(82.1271233340723,87.0865747939263,200.124999997952));
#30943=CARTESIAN_POINT('Ctrl Pts',(79.0328184976949,87.8391824855399,200.218749997952));
#30944=CARTESIAN_POINT('Ctrl Pts',(75.9385136613175,88.5917901771536,200.312499997952));
#30945=CARTESIAN_POINT('Ctrl Pts',(73.2183357261436,86.9359602466059,200.406249997952));
#30946=CARTESIAN_POINT('Ctrl Pts',(70.4981577909697,85.2801303160583,200.499999997952));
#30947=CARTESIAN_POINT('Ctrl Pts',(69.7455500993561,82.1858254796809,200.593749997952));
#30948=CARTESIAN_POINT('Ctrl Pts',(68.9929424077425,79.0915206433035,200.687499997952));
#30949=CARTESIAN_POINT('Ctrl Pts',(70.6487723382901,76.3713427081296,200.781249997952));
#30950=CARTESIAN_POINT('Ctrl Pts',(72.3046022688378,73.6511647729557,200.874999997952));
#30951=CARTESIAN_POINT('Ctrl Pts',(75.3989071052151,72.8985570813421,200.968749997952));
#30952=CARTESIAN_POINT('Ctrl Pts',(78.4932119415925,72.1459493897285,201.062499997952));
#30953=CARTESIAN_POINT('Ctrl Pts',(81.2133898767664,73.8017793202761,201.156249997952));
#30954=CARTESIAN_POINT('Ctrl Pts',(83.9335678119403,75.4576092508238,201.249999997952));
#30955=CARTESIAN_POINT('Ctrl Pts',(84.6861755035539,78.5519140872011,201.343749997952));
#30956=CARTESIAN_POINT('Ctrl Pts',(85.4387831951675,81.6462189235785,201.437499997952));
#30957=CARTESIAN_POINT('Ctrl Pts',(83.7829532646199,84.3663968587524,201.531249997952));
#30958=CARTESIAN_POINT('Ctrl Pts',(82.1271233340723,87.0865747939263,201.624999997952));
#30959=CARTESIAN_POINT('Ctrl Pts',(79.0328184976949,87.8391824855399,201.718749997952));
#30960=CARTESIAN_POINT('Ctrl Pts',(75.9385136613175,88.5917901771536,201.812499997952));
#30961=CARTESIAN_POINT('Ctrl Pts',(73.2183357261436,86.9359602466059,201.906249997952));
#30962=CARTESIAN_POINT('Ctrl Pts',(70.4981577909697,85.2801303160583,201.999999997952));
#30963=CARTESIAN_POINT('Ctrl Pts',(69.7455500993561,82.1858254796809,202.093749997952));
#30964=CARTESIAN_POINT('Ctrl Pts',(68.9929424077425,79.0915206433035,202.187499997952));
#30965=CARTESIAN_POINT('Ctrl Pts',(70.6487723382901,76.3713427081296,202.281249997952));
#30966=CARTESIAN_POINT('Ctrl Pts',(72.3046022688378,73.6511647729557,202.374999997952));
#30967=CARTESIAN_POINT('Ctrl Pts',(75.3989071052151,72.8985570813421,202.468749997952));
#30968=CARTESIAN_POINT('Ctrl Pts',(78.4932119415925,72.1459493897285,202.562499997952));
#30969=CARTESIAN_POINT('Ctrl Pts',(81.2133898767664,73.8017793202761,202.656249997952));
#30970=CARTESIAN_POINT('Ctrl Pts',(83.9335678119403,75.4576092508238,202.749999997952));
#30971=CARTESIAN_POINT('Ctrl Pts',(84.6861755035539,78.5519140872011,202.843749997952));
#30972=CARTESIAN_POINT('Ctrl Pts',(85.4387831951675,81.6462189235785,202.937499997952));
#30973=CARTESIAN_POINT('Ctrl Pts',(83.7829532646199,84.3663968587524,203.031249997952));
#30974=CARTESIAN_POINT('Ctrl Pts',(82.1271233340723,87.0865747939263,203.124999997952));
#30975=CARTESIAN_POINT('Ctrl Pts',(79.0328184976949,87.8391824855399,203.218749997952));
#30976=CARTESIAN_POINT('Ctrl Pts',(75.9385136613175,88.5917901771535,203.312499997952));
#30977=CARTESIAN_POINT('Ctrl Pts',(73.2183357261436,86.9359602466059,203.406249997952));
#30978=CARTESIAN_POINT('Ctrl Pts',(70.4981577909697,85.2801303160583,203.499999997952));
#30979=CARTESIAN_POINT('Ctrl Pts',(69.7455500993561,82.1858254796809,203.593749997952));
#30980=CARTESIAN_POINT('Ctrl Pts',(68.9929424077425,79.0915206433035,203.687499997952));
#30981=CARTESIAN_POINT('Ctrl Pts',(70.6487723382901,76.3713427081296,203.781249997952));
#30982=CARTESIAN_POINT('Ctrl Pts',(72.3046022688378,73.6511647729557,203.874999997952));
#30983=CARTESIAN_POINT('Ctrl Pts',(75.3989071052151,72.8985570813421,203.968749997952));
#30984=CARTESIAN_POINT('Ctrl Pts',(78.4932119415925,72.1459493897285,204.062499997952));
#30985=CARTESIAN_POINT('Ctrl Pts',(81.2133898767664,73.8017793202761,204.156249997952));
#30986=CARTESIAN_POINT('Ctrl Pts',(83.9335678119403,75.4576092508238,204.249999997952));
#30987=CARTESIAN_POINT('Ctrl Pts',(84.6861755035539,78.5519140872011,204.343749997952));
#30988=CARTESIAN_POINT('Ctrl Pts',(85.4387831951675,81.6462189235785,204.437499997952));
#30989=CARTESIAN_POINT('Ctrl Pts',(83.7829532646199,84.3663968587524,204.531249997952));
#30990=CARTESIAN_POINT('Ctrl Pts',(82.1271233340722,87.0865747939263,204.624999997952));
#30991=CARTESIAN_POINT('Ctrl Pts',(79.0328184976949,87.8391824855399,204.718749997952));
#30992=CARTESIAN_POINT('Ctrl Pts',(75.9385136613175,88.5917901771535,204.812499997952));
#30993=CARTESIAN_POINT('Ctrl Pts',(73.2183357261436,86.9359602466059,204.906249997952));
#30994=CARTESIAN_POINT('Ctrl Pts',(70.4981577909697,85.2801303160583,204.999999997952));
#30995=CARTESIAN_POINT('Ctrl Pts',(69.7455500993561,82.1858254796809,205.093749997952));
#30996=CARTESIAN_POINT('Ctrl Pts',(68.9929424077425,79.0915206433035,205.187499997952));
#30997=CARTESIAN_POINT('Ctrl Pts',(70.6487723382901,76.3713427081296,205.281249997952));
#30998=CARTESIAN_POINT('Ctrl Pts',(72.3046022688378,73.6511647729557,205.374999997952));
#30999=CARTESIAN_POINT('Ctrl Pts',(75.3989071052151,72.8985570813421,205.468749997952));
#31000=CARTESIAN_POINT('Ctrl Pts',(78.4932119415925,72.1459493897285,205.562499997952));
#31001=CARTESIAN_POINT('Ctrl Pts',(81.2133898767664,73.8017793202761,205.656249997952));
#31002=CARTESIAN_POINT('Ctrl Pts',(83.9335678119403,75.4576092508238,205.749999997952));
#31003=CARTESIAN_POINT('Ctrl Pts',(84.6861755035539,78.5519140872011,205.843749997952));
#31004=CARTESIAN_POINT('Ctrl Pts',(85.4387831951675,81.6462189235785,205.937499997952));
#31005=CARTESIAN_POINT('Ctrl Pts',(83.7829532646199,84.3663968587524,206.031249997952));
#31006=CARTESIAN_POINT('Ctrl Pts',(82.1271233340722,87.0865747939263,206.124999997952));
#31007=CARTESIAN_POINT('Ctrl Pts',(79.0328184976949,87.8391824855399,206.218749997952));
#31008=CARTESIAN_POINT('Ctrl Pts',(75.9385136613175,88.5917901771535,206.312499997952));
#31009=CARTESIAN_POINT('Ctrl Pts',(73.2183357261436,86.9359602466059,206.406249997952));
#31010=CARTESIAN_POINT('Ctrl Pts',(70.4981577909697,85.2801303160583,206.499999997952));
#31011=CARTESIAN_POINT('Ctrl Pts',(69.7455500993561,82.1858254796809,206.593749997952));
#31012=CARTESIAN_POINT('Ctrl Pts',(68.9929424077425,79.0915206433035,206.687499997952));
#31013=CARTESIAN_POINT('Ctrl Pts',(70.6487723382901,76.3713427081296,206.781249997952));
#31014=CARTESIAN_POINT('Ctrl Pts',(72.3046022688378,73.6511647729557,206.874999997952));
#31015=CARTESIAN_POINT('Ctrl Pts',(75.3989071052151,72.8985570813421,206.968749997952));
#31016=CARTESIAN_POINT('Ctrl Pts',(78.4932119415925,72.1459493897285,207.062499997952));
#31017=CARTESIAN_POINT('Ctrl Pts',(81.2133898767664,73.8017793202761,207.156249997952));
#31018=CARTESIAN_POINT('Ctrl Pts',(83.9335678119403,75.4576092508238,207.249999997952));
#31019=CARTESIAN_POINT('Ctrl Pts',(84.6861755035539,78.5519140872011,207.343749997952));
#31020=CARTESIAN_POINT('Ctrl Pts',(85.4387831951675,81.6462189235785,207.437499997952));
#31021=CARTESIAN_POINT('Ctrl Pts',(83.7829532646199,84.3663968587524,207.531249997952));
#31022=CARTESIAN_POINT('Ctrl Pts',(82.1271233340722,87.0865747939263,207.624999997952));
#31023=CARTESIAN_POINT('Ctrl Pts',(79.0328184976949,87.8391824855399,207.718749997952));
#31024=CARTESIAN_POINT('Ctrl Pts',(75.9385136613175,88.5917901771535,207.812499997952));
#31025=CARTESIAN_POINT('Ctrl Pts',(73.2183357261436,86.9359602466059,207.906249997952));
#31026=CARTESIAN_POINT('Ctrl Pts',(70.4981577909697,85.2801303160583,207.999999997952));
#31027=CARTESIAN_POINT('Ctrl Pts',(69.7455500993561,82.1858254796809,208.093749997952));
#31028=CARTESIAN_POINT('Ctrl Pts',(68.9929424077425,79.0915206433035,208.187499997952));
#31029=CARTESIAN_POINT('Ctrl Pts',(70.6487723382901,76.3713427081296,208.281249997952));
#31030=CARTESIAN_POINT('Ctrl Pts',(72.3046022688377,73.6511647729557,208.374999997952));
#31031=CARTESIAN_POINT('Ctrl Pts',(75.3989071052151,72.8985570813421,208.468749997952));
#31032=CARTESIAN_POINT('Ctrl Pts',(75.2070234291834,72.1096379759661,195.999988260337));
#31033=CARTESIAN_POINT('Ctrl Pts',(78.6281092586227,71.2775494633421,196.093738260337));
#31034=CARTESIAN_POINT('Ctrl Pts',(81.6355576774644,73.108247022536,196.187488260337));
#31035=CARTESIAN_POINT('Ctrl Pts',(84.643006096306,74.93894458173,196.281238260337));
#31036=CARTESIAN_POINT('Ctrl Pts',(85.47509460893,78.3600304111694,196.374988260337));
#31037=CARTESIAN_POINT('Ctrl Pts',(86.3071831215539,81.7811162406088,196.468738260337));
#31038=CARTESIAN_POINT('Ctrl Pts',(84.47648556236,84.7885646594504,196.562488260337));
#31039=CARTESIAN_POINT('Ctrl Pts',(82.645788003166,87.796013078292,196.656238260337));
#31040=CARTESIAN_POINT('Ctrl Pts',(79.2247021737267,88.628101590916,196.749988260337));
#31041=CARTESIAN_POINT('Ctrl Pts',(75.8036163442873,89.46019010354,196.843738260337));
#31042=CARTESIAN_POINT('Ctrl Pts',(72.7961679254456,87.629492544346,196.937488260337));
#31043=CARTESIAN_POINT('Ctrl Pts',(69.788719506604,85.7987949851521,197.031238260337));
#31044=CARTESIAN_POINT('Ctrl Pts',(68.95663099398,82.3777091557127,197.124988260337));
#31045=CARTESIAN_POINT('Ctrl Pts',(68.1245424813561,78.9566233262733,197.218738260337));
#31046=CARTESIAN_POINT('Ctrl Pts',(69.95524004055,75.9491749074317,197.312488260337));
#31047=CARTESIAN_POINT('Ctrl Pts',(71.785937599744,72.94172648859,197.406238260337));
#31048=CARTESIAN_POINT('Ctrl Pts',(75.2070234291834,72.1096379759661,197.499988260337));
#31049=CARTESIAN_POINT('Ctrl Pts',(78.6281092586227,71.2775494633421,197.593738260337));
#31050=CARTESIAN_POINT('Ctrl Pts',(81.6355576774644,73.108247022536,197.687488260337));
#31051=CARTESIAN_POINT('Ctrl Pts',(84.643006096306,74.93894458173,197.781238260337));
#31052=CARTESIAN_POINT('Ctrl Pts',(85.47509460893,78.3600304111694,197.874988260337));
#31053=CARTESIAN_POINT('Ctrl Pts',(86.3071831215539,81.7811162406088,197.968738260337));
#31054=CARTESIAN_POINT('Ctrl Pts',(84.47648556236,84.7885646594504,198.062488260337));
#31055=CARTESIAN_POINT('Ctrl Pts',(82.645788003166,87.796013078292,198.156238260337));
#31056=CARTESIAN_POINT('Ctrl Pts',(79.2247021737267,88.628101590916,198.249988260337));
#31057=CARTESIAN_POINT('Ctrl Pts',(75.8036163442873,89.46019010354,198.343738260337));
#31058=CARTESIAN_POINT('Ctrl Pts',(72.7961679254456,87.629492544346,198.437488260337));
#31059=CARTESIAN_POINT('Ctrl Pts',(69.788719506604,85.7987949851521,198.531238260337));
#31060=CARTESIAN_POINT('Ctrl Pts',(68.95663099398,82.3777091557127,198.624988260337));
#31061=CARTESIAN_POINT('Ctrl Pts',(68.1245424813561,78.9566233262733,198.718738260337));
#31062=CARTESIAN_POINT('Ctrl Pts',(69.95524004055,75.9491749074317,198.812488260337));
#31063=CARTESIAN_POINT('Ctrl Pts',(71.785937599744,72.94172648859,198.906238260337));
#31064=CARTESIAN_POINT('Ctrl Pts',(75.2070234291834,72.1096379759661,198.999988260337));
#31065=CARTESIAN_POINT('Ctrl Pts',(78.6281092586227,71.2775494633421,199.093738260337));
#31066=CARTESIAN_POINT('Ctrl Pts',(81.6355576774644,73.108247022536,199.187488260337));
#31067=CARTESIAN_POINT('Ctrl Pts',(84.643006096306,74.93894458173,199.281238260337));
#31068=CARTESIAN_POINT('Ctrl Pts',(85.47509460893,78.3600304111694,199.374988260337));
#31069=CARTESIAN_POINT('Ctrl Pts',(86.3071831215539,81.7811162406088,199.468738260337));
#31070=CARTESIAN_POINT('Ctrl Pts',(84.47648556236,84.7885646594504,199.562488260337));
#31071=CARTESIAN_POINT('Ctrl Pts',(82.645788003166,87.796013078292,199.656238260337));
#31072=CARTESIAN_POINT('Ctrl Pts',(79.2247021737267,88.628101590916,199.749988260337));
#31073=CARTESIAN_POINT('Ctrl Pts',(75.8036163442873,89.46019010354,199.843738260337));
#31074=CARTESIAN_POINT('Ctrl Pts',(72.7961679254456,87.629492544346,199.937488260337));
#31075=CARTESIAN_POINT('Ctrl Pts',(69.788719506604,85.7987949851521,200.031238260337));
#31076=CARTESIAN_POINT('Ctrl Pts',(68.95663099398,82.3777091557127,200.124988260337));
#31077=CARTESIAN_POINT('Ctrl Pts',(68.1245424813561,78.9566233262733,200.218738260337));
#31078=CARTESIAN_POINT('Ctrl Pts',(69.95524004055,75.9491749074317,200.312488260337));
#31079=CARTESIAN_POINT('Ctrl Pts',(71.785937599744,72.94172648859,200.406238260337));
#31080=CARTESIAN_POINT('Ctrl Pts',(75.2070234291834,72.1096379759661,200.499988260337));
#31081=CARTESIAN_POINT('Ctrl Pts',(78.6281092586227,71.2775494633421,200.593738260337));
#31082=CARTESIAN_POINT('Ctrl Pts',(81.6355576774644,73.108247022536,200.687488260337));
#31083=CARTESIAN_POINT('Ctrl Pts',(84.643006096306,74.93894458173,200.781238260337));
#31084=CARTESIAN_POINT('Ctrl Pts',(85.47509460893,78.3600304111694,200.874988260337));
#31085=CARTESIAN_POINT('Ctrl Pts',(86.3071831215539,81.7811162406088,200.968738260337));
#31086=CARTESIAN_POINT('Ctrl Pts',(84.47648556236,84.7885646594504,201.062488260337));
#31087=CARTESIAN_POINT('Ctrl Pts',(82.645788003166,87.796013078292,201.156238260337));
#31088=CARTESIAN_POINT('Ctrl Pts',(79.2247021737267,88.628101590916,201.249988260337));
#31089=CARTESIAN_POINT('Ctrl Pts',(75.8036163442873,89.46019010354,201.343738260337));
#31090=CARTESIAN_POINT('Ctrl Pts',(72.7961679254456,87.629492544346,201.437488260337));
#31091=CARTESIAN_POINT('Ctrl Pts',(69.788719506604,85.7987949851521,201.531238260337));
#31092=CARTESIAN_POINT('Ctrl Pts',(68.95663099398,82.3777091557127,201.624988260337));
#31093=CARTESIAN_POINT('Ctrl Pts',(68.1245424813561,78.9566233262733,201.718738260337));
#31094=CARTESIAN_POINT('Ctrl Pts',(69.95524004055,75.9491749074317,201.812488260337));
#31095=CARTESIAN_POINT('Ctrl Pts',(71.785937599744,72.94172648859,201.906238260337));
#31096=CARTESIAN_POINT('Ctrl Pts',(75.2070234291834,72.1096379759661,201.999988260337));
#31097=CARTESIAN_POINT('Ctrl Pts',(78.6281092586227,71.2775494633421,202.093738260337));
#31098=CARTESIAN_POINT('Ctrl Pts',(81.6355576774644,73.108247022536,202.187488260337));
#31099=CARTESIAN_POINT('Ctrl Pts',(84.643006096306,74.93894458173,202.281238260337));
#31100=CARTESIAN_POINT('Ctrl Pts',(85.47509460893,78.3600304111694,202.374988260337));
#31101=CARTESIAN_POINT('Ctrl Pts',(86.3071831215539,81.7811162406088,202.468738260337));
#31102=CARTESIAN_POINT('Ctrl Pts',(84.47648556236,84.7885646594504,202.562488260337));
#31103=CARTESIAN_POINT('Ctrl Pts',(82.645788003166,87.796013078292,202.656238260337));
#31104=CARTESIAN_POINT('Ctrl Pts',(79.2247021737267,88.628101590916,202.749988260337));
#31105=CARTESIAN_POINT('Ctrl Pts',(75.8036163442873,89.46019010354,202.843738260337));
#31106=CARTESIAN_POINT('Ctrl Pts',(72.7961679254456,87.629492544346,202.937488260337));
#31107=CARTESIAN_POINT('Ctrl Pts',(69.788719506604,85.7987949851521,203.031238260337));
#31108=CARTESIAN_POINT('Ctrl Pts',(68.95663099398,82.3777091557127,203.124988260337));
#31109=CARTESIAN_POINT('Ctrl Pts',(68.1245424813561,78.9566233262733,203.218738260337));
#31110=CARTESIAN_POINT('Ctrl Pts',(69.95524004055,75.9491749074317,203.312488260337));
#31111=CARTESIAN_POINT('Ctrl Pts',(71.785937599744,72.94172648859,203.406238260337));
#31112=CARTESIAN_POINT('Ctrl Pts',(75.2070234291834,72.1096379759661,203.499988260337));
#31113=CARTESIAN_POINT('Ctrl Pts',(78.6281092586227,71.2775494633421,203.593738260337));
#31114=CARTESIAN_POINT('Ctrl Pts',(81.6355576774644,73.108247022536,203.687488260337));
#31115=CARTESIAN_POINT('Ctrl Pts',(84.643006096306,74.93894458173,203.781238260337));
#31116=CARTESIAN_POINT('Ctrl Pts',(85.47509460893,78.3600304111694,203.874988260337));
#31117=CARTESIAN_POINT('Ctrl Pts',(86.3071831215539,81.7811162406088,203.968738260337));
#31118=CARTESIAN_POINT('Ctrl Pts',(84.47648556236,84.7885646594504,204.062488260337));
#31119=CARTESIAN_POINT('Ctrl Pts',(82.645788003166,87.796013078292,204.156238260337));
#31120=CARTESIAN_POINT('Ctrl Pts',(79.2247021737267,88.628101590916,204.249988260337));
#31121=CARTESIAN_POINT('Ctrl Pts',(75.8036163442873,89.46019010354,204.343738260337));
#31122=CARTESIAN_POINT('Ctrl Pts',(72.7961679254456,87.629492544346,204.437488260337));
#31123=CARTESIAN_POINT('Ctrl Pts',(69.788719506604,85.7987949851521,204.531238260337));
#31124=CARTESIAN_POINT('Ctrl Pts',(68.95663099398,82.3777091557127,204.624988260337));
#31125=CARTESIAN_POINT('Ctrl Pts',(68.1245424813561,78.9566233262733,204.718738260337));
#31126=CARTESIAN_POINT('Ctrl Pts',(69.95524004055,75.9491749074317,204.812488260337));
#31127=CARTESIAN_POINT('Ctrl Pts',(71.785937599744,72.94172648859,204.906238260337));
#31128=CARTESIAN_POINT('Ctrl Pts',(75.2070234291834,72.1096379759661,204.999988260337));
#31129=CARTESIAN_POINT('Ctrl Pts',(78.6281092586227,71.2775494633421,205.093738260337));
#31130=CARTESIAN_POINT('Ctrl Pts',(81.6355576774644,73.108247022536,205.187488260337));
#31131=CARTESIAN_POINT('Ctrl Pts',(84.643006096306,74.93894458173,205.281238260337));
#31132=CARTESIAN_POINT('Ctrl Pts',(85.47509460893,78.3600304111694,205.374988260337));
#31133=CARTESIAN_POINT('Ctrl Pts',(86.3071831215539,81.7811162406088,205.468738260337));
#31134=CARTESIAN_POINT('Ctrl Pts',(84.47648556236,84.7885646594504,205.562488260337));
#31135=CARTESIAN_POINT('Ctrl Pts',(82.645788003166,87.796013078292,205.656238260337));
#31136=CARTESIAN_POINT('Ctrl Pts',(79.2247021737267,88.628101590916,205.749988260337));
#31137=CARTESIAN_POINT('Ctrl Pts',(75.8036163442873,89.4601901035399,205.843738260337));
#31138=CARTESIAN_POINT('Ctrl Pts',(72.7961679254456,87.629492544346,205.937488260337));
#31139=CARTESIAN_POINT('Ctrl Pts',(69.788719506604,85.7987949851521,206.031238260337));
#31140=CARTESIAN_POINT('Ctrl Pts',(68.95663099398,82.3777091557127,206.124988260337));
#31141=CARTESIAN_POINT('Ctrl Pts',(68.1245424813561,78.9566233262733,206.218738260337));
#31142=CARTESIAN_POINT('Ctrl Pts',(69.95524004055,75.9491749074317,206.312488260337));
#31143=CARTESIAN_POINT('Ctrl Pts',(71.785937599744,72.94172648859,206.406238260337));
#31144=CARTESIAN_POINT('Ctrl Pts',(75.2070234291834,72.109637975966,206.499988260337));
#31145=CARTESIAN_POINT('Ctrl Pts',(78.6281092586227,71.2775494633421,206.593738260337));
#31146=CARTESIAN_POINT('Ctrl Pts',(81.6355576774644,73.108247022536,206.687488260337));
#31147=CARTESIAN_POINT('Ctrl Pts',(84.643006096306,74.93894458173,206.781238260337));
#31148=CARTESIAN_POINT('Ctrl Pts',(85.47509460893,78.3600304111694,206.874988260337));
#31149=CARTESIAN_POINT('Ctrl Pts',(86.3071831215539,81.7811162406088,206.968738260337));
#31150=CARTESIAN_POINT('Ctrl Pts',(84.47648556236,84.7885646594504,207.062488260337));
#31151=CARTESIAN_POINT('Ctrl Pts',(82.645788003166,87.796013078292,207.156238260337));
#31152=CARTESIAN_POINT('Ctrl Pts',(79.2247021737266,88.628101590916,207.249988260337));
#31153=CARTESIAN_POINT('Ctrl Pts',(75.8036163442873,89.4601901035399,207.343738260337));
#31154=CARTESIAN_POINT('Ctrl Pts',(72.7961679254456,87.629492544346,207.437488260337));
#31155=CARTESIAN_POINT('Ctrl Pts',(69.788719506604,85.7987949851521,207.531238260337));
#31156=CARTESIAN_POINT('Ctrl Pts',(68.95663099398,82.3777091557127,207.624988260337));
#31157=CARTESIAN_POINT('Ctrl Pts',(68.1245424813561,78.9566233262733,207.718738260337));
#31158=CARTESIAN_POINT('Ctrl Pts',(69.95524004055,75.9491749074317,207.812488260337));
#31159=CARTESIAN_POINT('Ctrl Pts',(71.785937599744,72.94172648859,207.906238260337));
#31160=CARTESIAN_POINT('Ctrl Pts',(75.2070234291834,72.109637975966,207.999988260337));
#31161=CARTESIAN_POINT('',(75.2070282347158,72.1096577336463,208.));
#31162=CARTESIAN_POINT('Ctrl Pts',(79.2246973785512,88.6280818307166,207.249999999716));
#31163=CARTESIAN_POINT('Ctrl Pts',(79.2165277293079,88.6300688815138,207.25022387789));
#31164=CARTESIAN_POINT('Ctrl Pts',(79.2083545666696,88.6320439481805,207.250447909143));
#31165=CARTESIAN_POINT('Ctrl Pts',(78.0953063455651,88.8992673886528,207.280964955017));
#31166=CARTESIAN_POINT('Ctrl Pts',(76.9484141012642,88.9403006829013,207.313446540827));
#31167=CARTESIAN_POINT('Ctrl Pts',(74.7496089525614,88.5762581883052,207.377678333948));
#31168=CARTESIAN_POINT('Ctrl Pts',(73.7162576426031,88.1916641629506,207.408769405604));
#31169=CARTESIAN_POINT('Ctrl Pts',(71.814354597471,87.0295873468618,207.468157984612));
#31170=CARTESIAN_POINT('Ctrl Pts',(70.9732538750771,86.2485920856208,207.500636005768));
#31171=CARTESIAN_POINT('Ctrl Pts',(69.673455491204,84.4377773413139,207.564876660879));
#31172=CARTESIAN_POINT('Ctrl Pts',(69.2134313752649,83.4355810486969,207.596008021778));
#31173=CARTESIAN_POINT('Ctrl Pts',(68.6876255490353,81.2693907373049,207.655374234711));
#31174=CARTESIAN_POINT('Ctrl Pts',(68.6437671802273,80.1223021883416,207.687848912984));
#31175=CARTESIAN_POINT('Ctrl Pts',(69.0025977101215,77.9221893998447,207.752094889348));
#31176=CARTESIAN_POINT('Ctrl Pts',(69.3848062472608,76.8876831559372,207.783248195099));
#31177=CARTESIAN_POINT('Ctrl Pts',(70.542588686374,74.9829099000098,207.842617588817));
#31178=CARTESIAN_POINT('Ctrl Pts',(71.3215831173499,74.1399909718324,207.875063759399));
#31179=CARTESIAN_POINT('Ctrl Pts',(73.1336685807777,72.8328855994505,207.939458270806));
#31180=CARTESIAN_POINT('Ctrl Pts',(74.140174969224,72.3691415323959,207.970764331008));
#31181=CARTESIAN_POINT('Ctrl Pts',(75.2070282347158,72.1096577336464,208.));
#31182=CARTESIAN_POINT('',(75.3029676699654,72.5041074074942,208.234374998976));
#31183=CARTESIAN_POINT('',(75.3989071052151,72.8985570813421,196.468749997952));
#31184=CARTESIAN_POINT('Ctrl Pts',(75.3989071052151,72.8985570813421,196.468749997952));
#31185=CARTESIAN_POINT('Ctrl Pts',(78.4932119415925,72.1459493897285,196.562499997952));
#31186=CARTESIAN_POINT('Ctrl Pts',(81.2133898767664,73.8017793202762,196.656249997952));
#31187=CARTESIAN_POINT('Ctrl Pts',(83.9335678119403,75.4576092508238,196.749999997952));
#31188=CARTESIAN_POINT('Ctrl Pts',(84.6861755035539,78.5519140872012,196.843749997952));
#31189=CARTESIAN_POINT('Ctrl Pts',(85.4387831951675,81.6462189235786,196.937499997952));
#31190=CARTESIAN_POINT('Ctrl Pts',(83.7829532646199,84.3663968587524,197.031249997952));
#31191=CARTESIAN_POINT('Ctrl Pts',(82.1271233340723,87.0865747939263,197.124999997952));
#31192=CARTESIAN_POINT('Ctrl Pts',(79.0328184976949,87.83918248554,197.218749997952));
#31193=CARTESIAN_POINT('',(75.3029676699654,72.5041074074942,196.234374998976));
#31194=CARTESIAN_POINT('Origin',(75.3029676699654,72.5041074074942,196.234374998976));
#31195=CARTESIAN_POINT('',(75.3989071052151,72.8985570813421,196.656249997952));
#31196=CARTESIAN_POINT('Origin',(77.215862801455,80.3688697834411,196.));
#31197=CARTESIAN_POINT('',(75.7269618872836,74.2473361465344,196.));
#31198=CARTESIAN_POINT('Origin',(77.215862801455,80.3688697834411,196.));
#31199=CARTESIAN_POINT('Origin',(77.215862801455,80.368869783441,212.));
#31200=CARTESIAN_POINT('',(75.7978619308155,74.5388377482919,200.));
#31201=CARTESIAN_POINT('Origin',(77.215862801455,80.3688697834411,200.));
#31202=CARTESIAN_POINT('',(75.7978619308155,74.5388377482919,196.3));
#31203=CARTESIAN_POINT('',(75.7978619308155,74.5388377482918,212.));
#31204=CARTESIAN_POINT('Origin',(77.215862801455,80.3688697834411,196.3));
#31205=CARTESIAN_POINT('Origin',(77.215862801455,80.3688697834411,196.));
#31206=CARTESIAN_POINT('',(75.2070282347158,72.1096577336463,208.656249997952));
#31207=CARTESIAN_POINT('Origin',(77.215862801455,80.368869783441,208.));
#31208=CARTESIAN_POINT('Origin',(77.215862801455,80.368869783441,196.656249997952));
#31209=CARTESIAN_POINT('Origin',(75.3029676699654,72.5041074074942,208.234374998976));
#31210=CARTESIAN_POINT('Origin',(77.215862801455,80.3688697834411,196.3));
#31211=CARTESIAN_POINT('Origin',(75.7269618872836,74.2473361465344,196.3));
#31212=CARTESIAN_POINT('Origin',(77.215862801455,80.368869783441,208.3));
#31213=CARTESIAN_POINT('',(74.9234280605879,70.9436513266165,208.));
#31214=CARTESIAN_POINT('Origin',(77.215862801455,80.368869783441,208.));
#31215=CARTESIAN_POINT('',(74.8525280170559,70.652149724859,208.3));
#31216=CARTESIAN_POINT('Origin',(74.9234280605879,70.9436513266165,208.3));
#31217=CARTESIAN_POINT('',(79.5791975858541,90.085589842023,208.3));
#31218=CARTESIAN_POINT('Origin',(77.215862801455,80.368869783441,208.3));
#31219=CARTESIAN_POINT('Origin',(77.215862801455,80.368869783441,208.3));
#31220=CARTESIAN_POINT('Origin',(77.215862801455,80.368869783441,212.5));
#31221=CARTESIAN_POINT('',(76.0932787788654,75.7534277556146,212.5));
#31222=CARTESIAN_POINT('Origin',(77.215862801455,80.368869783441,212.5));
#31223=CARTESIAN_POINT('',(76.0932787788654,75.7534277556146,212.));
#31224=CARTESIAN_POINT('',(76.0932787788654,75.7534277556146,212.5));
#31225=CARTESIAN_POINT('Origin',(77.215862801455,80.368869783441,212.));
#31226=CARTESIAN_POINT('Origin',(77.215862801455,80.368869783441,212.5));
#31227=CARTESIAN_POINT('',(75.5615284523756,73.5671657424336,212.));
#31228=CARTESIAN_POINT('Origin',(77.215862801455,80.368869783441,212.));
#31229=CARTESIAN_POINT('',(75.5615284523756,73.5671657424336,212.5));
#31230=CARTESIAN_POINT('',(75.5615284523756,73.5671657424336,212.5));
#31231=CARTESIAN_POINT('Origin',(77.215862801455,80.368869783441,212.5));
#31232=CARTESIAN_POINT('Origin',(77.215862801455,80.368869783441,212.5));
#31233=CARTESIAN_POINT('Origin',(77.215862801455,80.368869783441,212.));
#31234=CARTESIAN_POINT('',(75.7978619308155,74.5388377482918,212.));
#31235=CARTESIAN_POINT('Origin',(77.215862801455,80.368869783441,212.));
#31236=CARTESIAN_POINT('Origin',(77.215862801455,80.368869783441,208.));
#31237=CARTESIAN_POINT('',(75.5529660276326,70.5081003246406,210.));
#31238=CARTESIAN_POINT('',(74.1641752411726,70.8458868981042,210.));
#31239=CARTESIAN_POINT('Origin',(77.215862801455,80.368869783441,210.));
#31240=CARTESIAN_POINT('',(67.3550933426544,82.0317665572624,210.));
#31241=CARTESIAN_POINT('Origin',(77.215862801455,80.368869783441,210.));
#31242=CARTESIAN_POINT('',(67.6928799161183,83.4205573437238,210.));
#31243=CARTESIAN_POINT('Origin',(77.215862801455,80.368869783441,210.));
#31244=CARTESIAN_POINT('',(78.8787595752761,90.2296392422416,210.));
#31245=CARTESIAN_POINT('Origin',(77.215862801455,80.368869783441,210.));
#31246=CARTESIAN_POINT('',(79.5791975858541,90.085589842023,210.));
#31247=CARTESIAN_POINT('Origin',(77.215862801455,80.368869783441,210.));
#31248=CARTESIAN_POINT('',(79.5791975858541,90.085589842023,208.));
#31249=CARTESIAN_POINT('',(80.2675503617385,89.8918526687775,210.));
#31250=CARTESIAN_POINT('Origin',(77.215862801455,80.368869783441,210.));
#31251=CARTESIAN_POINT('',(87.0766322602554,78.7059730096184,210.));
#31252=CARTESIAN_POINT('Origin',(77.215862801455,80.368869783441,210.));
#31253=CARTESIAN_POINT('',(86.7388456867917,77.3171822231584,210.));
#31254=CARTESIAN_POINT('Origin',(77.215862801455,80.368869783441,210.));
#31255=CARTESIAN_POINT('Origin',(77.215862801455,80.368869783441,210.));
#31256=CARTESIAN_POINT('Origin',(77.215862801455,80.368869783441,208.));
#31257=CARTESIAN_POINT('Origin',(77.215862801455,80.368869783441,208.));
#31258=CARTESIAN_POINT('Origin',(77.215862801455,80.368869783441,210.));
#31259=CARTESIAN_POINT('',(79.5201142162436,89.8426718405577,210.));
#31260=CARTESIAN_POINT('Origin',(79.8155310642937,91.057261847881,210.));
#31261=CARTESIAN_POINT('Origin',(79.8155310642937,91.057261847881,210.));
#31262=CARTESIAN_POINT('Origin',(77.215862801455,80.368869783441,210.));
#31263=CARTESIAN_POINT('Origin',(66.5274707370145,82.9685380462795,210.));
#31264=CARTESIAN_POINT('Origin',(77.215862801455,80.368869783441,210.));
#31265=CARTESIAN_POINT('Origin',(74.6161945386162,69.6804777190005,210.));
#31266=CARTESIAN_POINT('Origin',(77.215862801455,80.368869783441,210.));
#31267=CARTESIAN_POINT('Origin',(87.9042548658952,77.769201520602,210.));
#31268=CARTESIAN_POINT('Origin',(79.8155310642937,91.057261847881,212.));
#31269=CARTESIAN_POINT('',(79.5201142162436,89.8426718405577,212.));
#31270=CARTESIAN_POINT('Origin',(79.8155310642937,91.057261847881,212.));
#31271=CARTESIAN_POINT('',(79.5201142162436,89.8426718405577,212.));
#31272=CARTESIAN_POINT('Origin',(79.8155310642937,91.057261847881,210.));
#31273=CARTESIAN_POINT('Origin',(66.5274707370145,82.9685380462795,212.));
#31274=CARTESIAN_POINT('',(66.2320538889645,81.7539480389562,212.));
#31275=CARTESIAN_POINT('Origin',(66.5274707370145,82.9685380462795,212.));
#31276=CARTESIAN_POINT('',(66.2320538889645,81.7539480389562,210.));
#31277=CARTESIAN_POINT('',(66.2320538889645,81.7539480389562,212.));
#31278=CARTESIAN_POINT('Origin',(66.5274707370145,82.9685380462795,210.));
#31279=CARTESIAN_POINT('Origin',(66.5274707370145,82.9685380462795,210.));
#31280=CARTESIAN_POINT('Origin',(74.6161945386162,69.6804777190005,212.));
#31281=CARTESIAN_POINT('',(74.3207776905663,68.4658877116775,212.));
#31282=CARTESIAN_POINT('Origin',(74.6161945386162,69.6804777190005,212.));
#31283=CARTESIAN_POINT('',(74.3207776905663,68.4658877116775,210.));
#31284=CARTESIAN_POINT('',(74.3207776905663,68.4658877116775,212.));
#31285=CARTESIAN_POINT('Origin',(74.6161945386162,69.6804777190005,210.));
#31286=CARTESIAN_POINT('Origin',(74.6161945386162,69.6804777190005,210.));
#31287=CARTESIAN_POINT('Origin',(87.9042548658952,77.769201520602,212.));
#31288=CARTESIAN_POINT('',(87.6088380178453,76.5546115132792,212.));
#31289=CARTESIAN_POINT('Origin',(87.9042548658952,77.769201520602,212.));
#31290=CARTESIAN_POINT('',(87.6088380178453,76.5546115132792,210.));
#31291=CARTESIAN_POINT('',(87.6088380178453,76.5546115132792,212.));
#31292=CARTESIAN_POINT('Origin',(87.9042548658952,77.769201520602,210.));
#31293=CARTESIAN_POINT('Origin',(87.9042548658952,77.769201520602,210.));
#31294=CARTESIAN_POINT('Origin',(77.215862801455,80.368869783441,212.));
#31295=CARTESIAN_POINT('',(75.7978619308155,74.5388377482918,210.));
#31296=CARTESIAN_POINT('',(75.7978619308155,74.5388377482918,212.));
#31297=CARTESIAN_POINT('Origin',(77.215862801455,80.368869783441,210.));
#31298=CARTESIAN_POINT('Origin',(92.5196968937216,76.6466174980124,212.));
#31299=CARTESIAN_POINT('',(90.8192708834698,77.0602010852822,210.));
#31300=CARTESIAN_POINT('',(92.5196968937216,76.6466174980124,210.));
#31301=CARTESIAN_POINT('',(92.5196968937216,76.6466174980124,210.));
#31302=CARTESIAN_POINT('',(92.5196968937216,76.6466174980124,212.));
#31303=CARTESIAN_POINT('',(92.5196968937216,76.6466174980124,212.));
#31304=CARTESIAN_POINT('',(90.8192708834698,77.0602010852822,212.));
#31305=CARTESIAN_POINT('',(92.5196968937216,76.6466174980124,212.));
#31306=CARTESIAN_POINT('',(90.8192708834698,77.0602010852822,212.));
#31307=CARTESIAN_POINT('Origin',(91.8627047718599,74.593730778034,212.));
#31308=CARTESIAN_POINT('',(91.8627047718599,74.593730778034,210.));
#31309=CARTESIAN_POINT('',(91.8627047718599,74.593730778034,210.));
#31310=CARTESIAN_POINT('',(91.8627047718599,74.593730778034,212.));
#31311=CARTESIAN_POINT('',(91.8627047718599,74.593730778034,212.));
#31312=CARTESIAN_POINT('',(91.8627047718599,74.593730778034,212.));
#31313=CARTESIAN_POINT('Origin',(90.2363869009964,75.2399429590628,212.));
#31314=CARTESIAN_POINT('',(90.2363869009964,75.2399429590628,210.));
#31315=CARTESIAN_POINT('',(90.2363869009964,75.2399429590628,210.));
#31316=CARTESIAN_POINT('',(90.2363869009964,75.2399429590628,212.));
#31317=CARTESIAN_POINT('',(90.2363869009964,75.2399429590628,212.));
#31318=CARTESIAN_POINT('',(90.2363869009964,75.2399429590628,212.));
#31319=CARTESIAN_POINT('Origin',(90.9263998414264,72.6522582414015,212.));
#31320=CARTESIAN_POINT('',(90.9263998414264,72.6522582414015,210.));
#31321=CARTESIAN_POINT('',(90.9263998414264,72.6522582414015,210.));
#31322=CARTESIAN_POINT('',(90.9263998414264,72.6522582414015,212.));
#31323=CARTESIAN_POINT('',(90.9263998414264,72.6522582414015,212.));
#31324=CARTESIAN_POINT('',(90.9263998414264,72.6522582414015,212.));
#31325=CARTESIAN_POINT('Origin',(89.4058445373984,73.5185212311411,212.));
#31326=CARTESIAN_POINT('',(89.4058445373984,73.5185212311411,210.));
#31327=CARTESIAN_POINT('',(89.4058445373984,73.5185212311411,210.));
#31328=CARTESIAN_POINT('',(89.4058445373984,73.5185212311411,212.));
#31329=CARTESIAN_POINT('',(89.4058445373984,73.5185212311411,212.));
#31330=CARTESIAN_POINT('',(89.4058445373984,73.5185212311411,212.));
#31331=CARTESIAN_POINT('Origin',(89.7290062128608,70.8599884426483,212.));
#31332=CARTESIAN_POINT('',(89.7290062128608,70.8599884426483,210.));
#31333=CARTESIAN_POINT('',(89.7290062128608,70.8599884426483,210.));
#31334=CARTESIAN_POINT('',(89.7290062128608,70.8599884426483,212.));
#31335=CARTESIAN_POINT('',(89.7290062128608,70.8599884426483,212.));
#31336=CARTESIAN_POINT('',(89.7290062128608,70.8599884426483,212.));
#31337=CARTESIAN_POINT('Origin',(88.3438093550553,71.9294414173629,212.));
#31338=CARTESIAN_POINT('',(88.3438093550553,71.9294414173629,210.));
#31339=CARTESIAN_POINT('',(88.3438093550553,71.9294414173629,210.));
#31340=CARTESIAN_POINT('',(88.3438093550553,71.9294414173629,212.));
#31341=CARTESIAN_POINT('',(88.3438093550553,71.9294414173629,212.));
#31342=CARTESIAN_POINT('',(88.3438093550553,71.9294414173629,212.));
#31343=CARTESIAN_POINT('Origin',(88.2938297911282,69.2518058747305,212.));
#31344=CARTESIAN_POINT('',(88.2938297911282,69.2518058747305,210.));
#31345=CARTESIAN_POINT('',(88.2938297911282,69.2518058747305,210.));
#31346=CARTESIAN_POINT('',(88.2938297911282,69.2518058747305,212.));
#31347=CARTESIAN_POINT('',(88.2938297911282,69.2518058747305,212.));
#31348=CARTESIAN_POINT('',(88.2938297911282,69.2518058747305,212.));
#31349=CARTESIAN_POINT('Origin',(87.0709526607442,70.5036331487519,212.));
#31350=CARTESIAN_POINT('',(87.0709526607442,70.5036331487519,210.));
#31351=CARTESIAN_POINT('',(87.0709526607442,70.5036331487519,210.));
#31352=CARTESIAN_POINT('',(87.0709526607442,70.5036331487519,212.));
#31353=CARTESIAN_POINT('',(87.0709526607442,70.5036331487519,212.));
#31354=CARTESIAN_POINT('',(87.0709526607442,70.5036331487519,212.));
#31355=CARTESIAN_POINT('Origin',(86.6488046527885,67.8590119820519,212.));
#31356=CARTESIAN_POINT('',(86.6488046527885,67.8590119820519,210.));
#31357=CARTESIAN_POINT('',(86.6488046527885,67.8590119820519,210.));
#31358=CARTESIAN_POINT('',(86.6488046527885,67.8590119820519,212.));
#31359=CARTESIAN_POINT('',(86.6488046527885,67.8590119820519,212.));
#31360=CARTESIAN_POINT('',(86.6488046527885,67.8590119820519,212.));
#31361=CARTESIAN_POINT('Origin',(85.6120491621669,69.2688481614238,212.));
#31362=CARTESIAN_POINT('',(85.6120491621669,69.2688481614238,210.));
#31363=CARTESIAN_POINT('',(85.6120491621669,69.2688481614238,210.));
#31364=CARTESIAN_POINT('',(85.6120491621669,69.2688481614238,212.));
#31365=CARTESIAN_POINT('',(85.6120491621669,69.2688481614238,212.));
#31366=CARTESIAN_POINT('',(85.6120491621669,69.2688481614238,212.));
#31367=CARTESIAN_POINT('Origin',(84.8259493409712,66.708715913454,212.));
#31368=CARTESIAN_POINT('',(84.8259493409713,66.708715913454,210.));
#31369=CARTESIAN_POINT('',(84.8259493409713,66.708715913454,210.));
#31370=CARTESIAN_POINT('',(84.8259493409712,66.708715913454,212.));
#31371=CARTESIAN_POINT('',(84.8259493409712,66.708715913454,212.));
#31372=CARTESIAN_POINT('',(84.8259493409712,66.708715913454,212.));
#31373=CARTESIAN_POINT('Origin',(83.995494756445,68.2491201406098,212.));
#31374=CARTESIAN_POINT('',(83.995494756445,68.2491201406098,210.));
#31375=CARTESIAN_POINT('',(83.995494756445,68.2491201406098,210.));
#31376=CARTESIAN_POINT('',(83.995494756445,68.2491201406098,212.));
#31377=CARTESIAN_POINT('',(83.995494756445,68.2491201406098,212.));
#31378=CARTESIAN_POINT('',(83.995494756445,68.2491201406098,212.));
#31379=CARTESIAN_POINT('Origin',(82.8607436608537,65.8233068734697,212.));
#31380=CARTESIAN_POINT('',(82.8607436608537,65.8233068734697,210.));
#31381=CARTESIAN_POINT('',(82.8607436608537,65.8233068734697,210.));
#31382=CARTESIAN_POINT('',(82.8607436608537,65.8233068734697,212.));
#31383=CARTESIAN_POINT('',(82.8607436608537,65.8233068734697,212.));
#31384=CARTESIAN_POINT('',(82.8607436608537,65.8233068734697,212.));
#31385=CARTESIAN_POINT('Origin',(82.2527538362826,67.4642969323117,212.));
#31386=CARTESIAN_POINT('',(82.2527538362826,67.4642969323117,210.));
#31387=CARTESIAN_POINT('',(82.2527538362826,67.4642969323117,210.));
#31388=CARTESIAN_POINT('',(82.2527538362826,67.4642969323117,212.));
#31389=CARTESIAN_POINT('',(82.2527538362826,67.4642969323117,212.));
#31390=CARTESIAN_POINT('',(82.2527538362826,67.4642969323117,212.));
#31391=CARTESIAN_POINT('Origin',(80.791438105611,65.2200183419245,212.));
#31392=CARTESIAN_POINT('',(80.7914381056111,65.2200183419245,210.));
#31393=CARTESIAN_POINT('',(80.7914381056111,65.2200183419245,210.));
#31394=CARTESIAN_POINT('',(80.791438105611,65.2200183419245,212.));
#31395=CARTESIAN_POINT('',(80.791438105611,65.2200183419245,212.));
#31396=CARTESIAN_POINT('',(80.791438105611,65.2200183419245,212.));
#31397=CARTESIAN_POINT('Origin',(80.4177468713522,66.9296542275557,212.));
#31398=CARTESIAN_POINT('',(80.4177468713522,66.9296542275557,210.));
#31399=CARTESIAN_POINT('',(80.4177468713522,66.9296542275557,210.));
#31400=CARTESIAN_POINT('',(80.4177468713522,66.9296542275557,212.));
#31401=CARTESIAN_POINT('',(80.4177468713522,66.9296542275557,212.));
#31402=CARTESIAN_POINT('',(80.4177468713522,66.9296542275557,212.));
#31403=CARTESIAN_POINT('Origin',(78.6583093540759,64.9105926438542,212.));
#31404=CARTESIAN_POINT('',(78.6583093540759,64.9105926438542,210.));
#31405=CARTESIAN_POINT('',(78.6583093540759,64.9105926438542,210.));
#31406=CARTESIAN_POINT('',(78.6583093540759,64.9105926438542,212.));
#31407=CARTESIAN_POINT('',(78.6583093540759,64.9105926438542,212.));
#31408=CARTESIAN_POINT('',(78.6583093540759,64.9105926438542,212.));
#31409=CARTESIAN_POINT('Origin',(78.5261901849366,66.6555982384429,212.));
#31410=CARTESIAN_POINT('',(78.5261901849366,66.6555982384429,210.));
#31411=CARTESIAN_POINT('',(78.5261901849366,66.6555982384429,210.));
#31412=CARTESIAN_POINT('',(78.5261901849366,66.6555982384429,212.));
#31413=CARTESIAN_POINT('',(78.5261901849366,66.6555982384429,212.));
#31414=CARTESIAN_POINT('',(78.5261901849366,66.6555982384429,212.));
#31415=CARTESIAN_POINT('Origin',(76.5028763309989,64.9010523985053,212.));
#31416=CARTESIAN_POINT('',(76.5028763309989,64.9010523985053,210.));
#31417=CARTESIAN_POINT('',(76.5028763309989,64.9010523985053,210.));
#31418=CARTESIAN_POINT('',(76.5028763309989,64.9010523985053,212.));
#31419=CARTESIAN_POINT('',(76.5028763309989,64.9010523985053,212.));
#31420=CARTESIAN_POINT('',(76.5028763309989,64.9010523985053,212.));
#31421=CARTESIAN_POINT('Origin',(76.6149007763232,66.6474631530673,212.));
#31422=CARTESIAN_POINT('',(76.6149007763232,66.6474631530673,210.));
#31423=CARTESIAN_POINT('',(76.6149007763232,66.6474631530673,210.));
#31424=CARTESIAN_POINT('',(76.6149007763232,66.6474631530673,212.));
#31425=CARTESIAN_POINT('',(76.6149007763232,66.6474631530673,212.));
#31426=CARTESIAN_POINT('',(76.6149007763232,66.6474631530673,212.));
#31427=CARTESIAN_POINT('Origin',(74.3670920884055,65.1915832959018,212.));
#31428=CARTESIAN_POINT('',(74.3670920884055,65.1915832959018,210.));
#31429=CARTESIAN_POINT('',(74.3670920884055,65.1915832959018,210.));
#31430=CARTESIAN_POINT('',(74.3670920884055,65.1915832959018,212.));
#31431=CARTESIAN_POINT('',(74.3670920884055,65.1915832959018,212.));
#31432=CARTESIAN_POINT('',(74.3670920884055,65.1915832959018,212.));
#31433=CARTESIAN_POINT('Origin',(74.721079719791,66.9054073116123,212.));
#31434=CARTESIAN_POINT('',(74.721079719791,66.9054073116123,210.));
#31435=CARTESIAN_POINT('',(74.721079719791,66.9054073116123,210.));
#31436=CARTESIAN_POINT('',(74.721079719791,66.9054073116123,212.));
#31437=CARTESIAN_POINT('',(74.721079719791,66.9054073116123,212.));
#31438=CARTESIAN_POINT('',(74.721079719791,66.9054073116123,212.));
#31439=CARTESIAN_POINT('Origin',(72.2925272371593,65.7765304825996,212.));
#31440=CARTESIAN_POINT('',(72.2925272371593,65.7765304825996,210.));
#31441=CARTESIAN_POINT('',(72.2925272371593,65.7765304825996,210.));
#31442=CARTESIAN_POINT('',(72.2925272371593,65.7765304825996,212.));
#31443=CARTESIAN_POINT('',(72.2925272371593,65.7765304825996,212.));
#31444=CARTESIAN_POINT('',(72.2925272371593,65.7765304825996,212.));
#31445=CARTESIAN_POINT('Origin',(72.8815880880161,67.4244101244388,212.));
#31446=CARTESIAN_POINT('',(72.8815880880161,67.4244101244388,210.));
#31447=CARTESIAN_POINT('',(72.8815880880161,67.4244101244388,210.));
#31448=CARTESIAN_POINT('',(72.8815880880161,67.4244101244388,212.));
#31449=CARTESIAN_POINT('',(72.8815880880161,67.4244101244388,212.));
#31450=CARTESIAN_POINT('',(72.8815880880161,67.4244101244388,212.));
#31451=CARTESIAN_POINT('Origin',(70.3195608223071,66.6445086269775,212.));
#31452=CARTESIAN_POINT('',(70.3195608223071,66.6445086269775,210.));
#31453=CARTESIAN_POINT('',(70.3195608223071,66.6445086269775,210.));
#31454=CARTESIAN_POINT('',(70.3195608223071,66.6445086269775,212.));
#31455=CARTESIAN_POINT('',(70.3195608223071,66.6445086269775,212.));
#31456=CARTESIAN_POINT('',(70.3195608223071,66.6445086269775,212.));
#31457=CARTESIAN_POINT('Origin',(71.1322294932201,68.1943697921522,212.));
#31458=CARTESIAN_POINT('',(71.1322294932201,68.1943697921522,210.));
#31459=CARTESIAN_POINT('',(71.1322294932201,68.1943697921522,210.));
#31460=CARTESIAN_POINT('',(71.1322294932201,68.1943697921522,212.));
#31461=CARTESIAN_POINT('',(71.1322294932201,68.1943697921522,212.));
#31462=CARTESIAN_POINT('',(71.1322294932201,68.1943697921522,212.));
#31463=CARTESIAN_POINT('Origin',(68.4865943908981,67.7786235217654,212.));
#31464=CARTESIAN_POINT('',(68.4865943908981,67.7786235217654,210.));
#31465=CARTESIAN_POINT('',(68.4865943908981,67.7786235217654,210.));
#31466=CARTESIAN_POINT('',(68.4865943908981,67.7786235217654,212.));
#31467=CARTESIAN_POINT('',(68.4865943908981,67.7786235217654,212.));
#31468=CARTESIAN_POINT('',(68.4865943908981,67.7786235217654,212.));
#31469=CARTESIAN_POINT('Origin',(69.5070532105848,69.2002999256365,212.));
#31470=CARTESIAN_POINT('',(69.5070532105848,69.2002999256365,210.));
#31471=CARTESIAN_POINT('',(69.5070532105848,69.2002999256365,210.));
#31472=CARTESIAN_POINT('',(69.5070532105848,69.2002999256365,212.));
#31473=CARTESIAN_POINT('',(69.5070532105848,69.2002999256365,212.));
#31474=CARTESIAN_POINT('',(69.5070532105848,69.2002999256365,212.));
#31475=CARTESIAN_POINT('Origin',(66.8293045495512,69.156800910573,212.));
#31476=CARTESIAN_POINT('',(66.8293045495512,69.156800910573,210.));
#31477=CARTESIAN_POINT('',(66.8293045495512,69.156800910573,210.));
#31478=CARTESIAN_POINT('',(66.8293045495512,69.156800910573,212.));
#31479=CARTESIAN_POINT('',(66.8293045495512,69.156800910573,212.));
#31480=CARTESIAN_POINT('',(66.8293045495512,69.156800910573,212.));
#31481=CARTESIAN_POINT('Origin',(68.0376914478412,70.422621239072,212.));
#31482=CARTESIAN_POINT('',(68.0376914478412,70.422621239072,210.));
#31483=CARTESIAN_POINT('',(68.0376914478412,70.422621239072,210.));
#31484=CARTESIAN_POINT('',(68.0376914478412,70.422621239072,212.));
#31485=CARTESIAN_POINT('',(68.0376914478412,70.422621239072,212.));
#31486=CARTESIAN_POINT('',(68.0376914478412,70.422621239072,212.));
#31487=CARTESIAN_POINT('Origin',(65.379948559889,70.7522161381807,212.));
#31488=CARTESIAN_POINT('',(65.379948559889,70.7522161381807,210.));
#31489=CARTESIAN_POINT('',(65.379948559889,70.7522161381807,210.));
#31490=CARTESIAN_POINT('',(65.379948559889,70.7522161381807,212.));
#31491=CARTESIAN_POINT('',(65.379948559889,70.7522161381807,212.));
#31492=CARTESIAN_POINT('',(65.379948559889,70.7522161381807,212.));
#31493=CARTESIAN_POINT('Origin',(66.7527436603267,71.8375426384627,212.));
#31494=CARTESIAN_POINT('',(66.7527436603267,71.8375426384627,210.));
#31495=CARTESIAN_POINT('',(66.7527436603267,71.8375426384627,210.));
#31496=CARTESIAN_POINT('',(66.7527436603267,71.8375426384627,212.));
#31497=CARTESIAN_POINT('',(66.7527436603267,71.8375426384627,212.));
#31498=CARTESIAN_POINT('',(66.7527436603267,71.8375426384627,212.));
#31499=CARTESIAN_POINT('Origin',(64.1667364876323,72.533816261941,212.));
#31500=CARTESIAN_POINT('',(64.1667364876323,72.533816261941,210.));
#31501=CARTESIAN_POINT('',(64.1667364876323,72.533816261941,210.));
#31502=CARTESIAN_POINT('',(64.1667364876323,72.533816261941,212.));
#31503=CARTESIAN_POINT('',(64.1667364876323,72.533816261941,212.));
#31504=CARTESIAN_POINT('',(64.1667364876323,72.533816261941,212.));
#31505=CARTESIAN_POINT('Origin',(65.677219895119,73.4175242882186,212.));
#31506=CARTESIAN_POINT('',(65.677219895119,73.4175242882186,210.));
#31507=CARTESIAN_POINT('',(65.677219895119,73.4175242882186,210.));
#31508=CARTESIAN_POINT('',(65.677219895119,73.4175242882186,212.));
#31509=CARTESIAN_POINT('',(65.677219895119,73.4175242882186,212.));
#31510=CARTESIAN_POINT('',(65.677219895119,73.4175242882186,212.));
#31511=CARTESIAN_POINT('Origin',(63.2132821257592,74.466924461985,212.));
#31512=CARTESIAN_POINT('',(63.2132821257592,74.466924461985,210.));
#31513=CARTESIAN_POINT('',(63.2132821257592,74.466924461985,210.));
#31514=CARTESIAN_POINT('',(63.2132821257592,74.466924461985,212.));
#31515=CARTESIAN_POINT('',(63.2132821257592,74.466924461985,212.));
#31516=CARTESIAN_POINT('',(63.2132821257592,74.466924461985,212.));
#31517=CARTESIAN_POINT('Origin',(64.8320539989176,75.1318136427297,212.));
#31518=CARTESIAN_POINT('',(64.8320539989176,75.1318136427297,210.));
#31519=CARTESIAN_POINT('',(64.8320539989176,75.1318136427297,210.));
#31520=CARTESIAN_POINT('',(64.8320539989176,75.1318136427297,212.));
#31521=CARTESIAN_POINT('',(64.8320539989176,75.1318136427297,212.));
#31522=CARTESIAN_POINT('',(64.8320539989176,75.1318136427297,212.));
#31523=CARTESIAN_POINT('Origin',(62.5381433788854,76.5139149860768,212.));
#31524=CARTESIAN_POINT('',(62.5381433788854,76.5139149860768,210.));
#31525=CARTESIAN_POINT('',(62.5381433788854,76.5139149860768,210.));
#31526=CARTESIAN_POINT('',(62.5381433788854,76.5139149860768,212.));
#31527=CARTESIAN_POINT('',(62.5381433788854,76.5139149860768,212.));
#31528=CARTESIAN_POINT('',(62.5381433788854,76.5139149860768,212.));
#31529=CARTESIAN_POINT('Origin',(64.2336961645301,76.9470440096857,212.));
#31530=CARTESIAN_POINT('',(64.2336961645301,76.9470440096857,210.));
#31531=CARTESIAN_POINT('',(64.2336961645301,76.9470440096857,210.));
#31532=CARTESIAN_POINT('',(64.2336961645301,76.9470440096857,212.));
#31533=CARTESIAN_POINT('',(64.2336961645301,76.9470440096857,212.));
#31534=CARTESIAN_POINT('',(64.2336961645301,76.9470440096857,212.));
#31535=CARTESIAN_POINT('Origin',(62.1544610547598,78.6349454920823,212.));
#31536=CARTESIAN_POINT('',(62.1544610547598,78.6349454920823,210.));
#31537=CARTESIAN_POINT('',(62.1544610547598,78.6349454920823,210.));
#31538=CARTESIAN_POINT('',(62.1544610547598,78.6349454920823,212.));
#31539=CARTESIAN_POINT('',(62.1544610547598,78.6349454920823,212.));
#31540=CARTESIAN_POINT('',(62.1544610547598,78.6349454920823,212.));
#31541=CARTESIAN_POINT('Origin',(63.893792746581,78.8278839947877,212.));
#31542=CARTESIAN_POINT('',(63.893792746581,78.8278839947877,210.));
#31543=CARTESIAN_POINT('',(63.893792746581,78.8278839947877,210.));
#31544=CARTESIAN_POINT('',(63.893792746581,78.8278839947877,212.));
#31545=CARTESIAN_POINT('',(63.893792746581,78.8278839947877,212.));
#31546=CARTESIAN_POINT('',(63.893792746581,78.8278839947877,212.));
#31547=CARTESIAN_POINT('Origin',(62.0697030933893,80.7887325338384,212.));
#31548=CARTESIAN_POINT('',(62.0697030933893,80.7887325338384,210.));
#31549=CARTESIAN_POINT('',(62.0697030933893,80.7887325338384,210.));
#31550=CARTESIAN_POINT('',(62.0697030933893,80.7887325338384,212.));
#31551=CARTESIAN_POINT('',(62.0697030933893,80.7887325338384,212.));
#31552=CARTESIAN_POINT('',(62.0697030933893,80.7887325338384,212.));
#31553=CARTESIAN_POINT('Origin',(63.8189595784662,80.7377251871495,212.));
#31554=CARTESIAN_POINT('',(63.8189595784662,80.7377251871495,210.));
#31555=CARTESIAN_POINT('',(63.8189595784662,80.7377251871495,210.));
#31556=CARTESIAN_POINT('',(63.8189595784662,80.7377251871495,212.));
#31557=CARTESIAN_POINT('',(63.8189595784662,80.7377251871495,212.));
#31558=CARTESIAN_POINT('',(63.8189595784662,80.7377251871495,212.));
#31559=CARTESIAN_POINT('Origin',(62.2855192120812,82.9333550964738,212.));
#31560=CARTESIAN_POINT('',(62.2855192120812,82.9333550964738,210.));
#31561=CARTESIAN_POINT('',(62.2855192120812,82.9333550964738,210.));
#31562=CARTESIAN_POINT('',(62.2855192120812,82.9333550964738,212.));
#31563=CARTESIAN_POINT('',(62.2855192120812,82.9333550964738,212.));
#31564=CARTESIAN_POINT('',(62.2855192120812,82.9333550964738,212.));
#31565=CARTESIAN_POINT('Origin',(64.0106532026816,82.6393947003739,212.));
#31566=CARTESIAN_POINT('',(64.0106532026816,82.6393947003739,210.));
#31567=CARTESIAN_POINT('',(64.0106532026816,82.6393947003739,210.));
#31568=CARTESIAN_POINT('',(64.0106532026816,82.6393947003739,212.));
#31569=CARTESIAN_POINT('',(64.0106532026816,82.6393947003739,212.));
#31570=CARTESIAN_POINT('',(64.0106532026816,82.6393947003739,212.));
#31571=CARTESIAN_POINT('Origin',(62.7977087955725,85.0270705412788,212.));
#31572=CARTESIAN_POINT('',(62.7977087955725,85.0270705412788,210.));
#31573=CARTESIAN_POINT('',(62.7977087955725,85.0270705412788,210.));
#31574=CARTESIAN_POINT('',(62.7977087955725,85.0270705412788,212.));
#31575=CARTESIAN_POINT('',(62.7977087955725,85.0270705412788,212.));
#31576=CARTESIAN_POINT('',(62.7977087955725,85.0270705412788,212.));
#31577=CARTESIAN_POINT('Origin',(64.4651425208801,84.495878700503,212.));
#31578=CARTESIAN_POINT('',(64.4651425208801,84.495878700503,210.));
#31579=CARTESIAN_POINT('',(64.4651425208801,84.495878700503,210.));
#31580=CARTESIAN_POINT('',(64.4651425208801,84.495878700503,212.));
#31581=CARTESIAN_POINT('',(64.4651425208801,84.495878700503,212.));
#31582=CARTESIAN_POINT('',(64.4651425208801,84.495878700503,212.));
#31583=CARTESIAN_POINT('Origin',(63.5963026562275,87.0291270786864,212.));
#31584=CARTESIAN_POINT('',(63.5963026562275,87.0291270786864,210.));
#31585=CARTESIAN_POINT('',(63.5963026562275,87.0291270786864,210.));
#31586=CARTESIAN_POINT('',(63.5963026562275,87.0291270786864,212.));
#31587=CARTESIAN_POINT('',(63.5963026562275,87.0291270786864,212.));
#31588=CARTESIAN_POINT('',(63.5963026562275,87.0291270786864,212.));
#31589=CARTESIAN_POINT('Origin',(65.173581415457,86.2710428381936,212.));
#31590=CARTESIAN_POINT('',(65.173581415457,86.2710428381936,210.));
#31591=CARTESIAN_POINT('',(65.173581415457,86.2710428381936,210.));
#31592=CARTESIAN_POINT('',(65.173581415457,86.2710428381936,212.));
#31593=CARTESIAN_POINT('',(65.173581415457,86.2710428381936,212.));
#31594=CARTESIAN_POINT('',(65.173581415457,86.2710428381936,212.));
#31595=CARTESIAN_POINT('Origin',(64.6657570729356,88.9005569555014,212.));
#31596=CARTESIAN_POINT('',(64.6657570729356,88.9005569555014,210.));
#31597=CARTESIAN_POINT('',(64.6657570729356,88.9005569555014,210.));
#31598=CARTESIAN_POINT('',(64.6657570729356,88.9005569555014,212.));
#31599=CARTESIAN_POINT('',(64.6657570729356,88.9005569555014,212.));
#31600=CARTESIAN_POINT('',(64.6657570729356,88.9005569555014,212.));
#31601=CARTESIAN_POINT('Origin',(66.1221809291665,87.9303355627247,212.));
#31602=CARTESIAN_POINT('',(66.1221809291665,87.9303355627247,210.));
#31603=CARTESIAN_POINT('',(66.1221809291665,87.9303355627247,210.));
#31604=CARTESIAN_POINT('',(66.1221809291665,87.9303355627247,212.));
#31605=CARTESIAN_POINT('',(66.1221809291665,87.9303355627247,212.));
#31606=CARTESIAN_POINT('',(66.1221809291665,87.9303355627247,212.));
#31607=CARTESIAN_POINT('Origin',(65.9852563319619,90.6049349178915,212.));
#31608=CARTESIAN_POINT('',(65.9852563319619,90.6049349178915,210.));
#31609=CARTESIAN_POINT('',(65.9852563319619,90.6049349178915,210.));
#31610=CARTESIAN_POINT('',(65.9852563319619,90.6049349178915,212.));
#31611=CARTESIAN_POINT('',(65.9852563319619,90.6049349178915,212.));
#31612=CARTESIAN_POINT('',(65.9852563319619,90.6049349178915,212.));
#31613=CARTESIAN_POINT('Origin',(67.2924776514903,89.441460628631,212.));
#31614=CARTESIAN_POINT('',(67.2924776514903,89.441460628631,210.));
#31615=CARTESIAN_POINT('',(67.2924776514903,89.441460628631,210.));
#31616=CARTESIAN_POINT('',(67.2924776514903,89.441460628631,212.));
#31617=CARTESIAN_POINT('',(67.2924776514903,89.441460628631,212.));
#31618=CARTESIAN_POINT('',(67.2924776514903,89.441460628631,212.));
#31619=CARTESIAN_POINT('Origin',(67.5291178811376,92.1090871875201,212.));
#31620=CARTESIAN_POINT('',(67.5291178811376,92.1090871875201,210.));
#31621=CARTESIAN_POINT('',(67.5291178811376,92.1090871875201,210.));
#31622=CARTESIAN_POINT('',(67.5291178811376,92.1090871875201,212.));
#31623=CARTESIAN_POINT('',(67.5291178811376,92.1090871875201,212.));
#31624=CARTESIAN_POINT('',(67.5291178811376,92.1090871875201,212.));
#31625=CARTESIAN_POINT('Origin',(68.6616930879211,90.7750057053837,212.));
#31626=CARTESIAN_POINT('',(68.6616930879211,90.7750057053837,210.));
#31627=CARTESIAN_POINT('',(68.6616930879211,90.7750057053837,210.));
#31628=CARTESIAN_POINT('',(68.6616930879211,90.7750057053837,212.));
#31629=CARTESIAN_POINT('',(68.6616930879211,90.7750057053837,212.));
#31630=CARTESIAN_POINT('',(68.6616930879211,90.7750057053837,212.));
#31631=CARTESIAN_POINT('Origin',(69.2672922115245,93.3837371514067,212.));
#31632=CARTESIAN_POINT('',(69.2672922115245,93.3837371514067,210.));
#31633=CARTESIAN_POINT('',(69.2672922115245,93.3837371514067,210.));
#31634=CARTESIAN_POINT('',(69.2672922115245,93.3837371514067,212.));
#31635=CARTESIAN_POINT('',(69.2672922115245,93.3837371514067,212.));
#31636=CARTESIAN_POINT('',(69.2672922115245,93.3837371514067,212.));
#31637=CARTESIAN_POINT('Origin',(70.2031770174483,91.905014854949,212.));
#31638=CARTESIAN_POINT('',(70.2031770174483,91.905014854949,210.));
#31639=CARTESIAN_POINT('',(70.2031770174483,91.905014854949,210.));
#31640=CARTESIAN_POINT('',(70.2031770174483,91.905014854949,212.));
#31641=CARTESIAN_POINT('',(70.2031770174483,91.905014854949,212.));
#31642=CARTESIAN_POINT('',(70.2031770174483,91.905014854949,212.));
#31643=CARTESIAN_POINT('Origin',(71.1659477369257,94.404075197897,212.));
#31644=CARTESIAN_POINT('',(71.1659477369257,94.404075197897,210.));
#31645=CARTESIAN_POINT('',(71.1659477369257,94.404075197897,210.));
#31646=CARTESIAN_POINT('',(71.1659477369257,94.404075197897,212.));
#31647=CARTESIAN_POINT('',(71.1659477369257,94.404075197897,212.));
#31648=CARTESIAN_POINT('',(71.1659477369257,94.404075197897,212.));
#31649=CARTESIAN_POINT('Origin',(71.8869262087956,92.809493734597,212.));
#31650=CARTESIAN_POINT('',(71.8869262087956,92.809493734597,210.));
#31651=CARTESIAN_POINT('',(71.8869262087956,92.809493734597,210.));
#31652=CARTESIAN_POINT('',(71.8869262087956,92.809493734597,212.));
#31653=CARTESIAN_POINT('',(71.8869262087956,92.809493734597,212.));
#31654=CARTESIAN_POINT('',(71.8869262087956,92.809493734597,212.));
#31655=CARTESIAN_POINT('Origin',(73.1881292872278,95.1502416075335,212.));
#31656=CARTESIAN_POINT('',(73.1881292872279,95.1502416075335,210.));
#31657=CARTESIAN_POINT('',(73.1881292872279,95.1502416075335,210.));
#31658=CARTESIAN_POINT('',(73.1881292872278,95.1502416075335,212.));
#31659=CARTESIAN_POINT('',(73.1881292872278,95.1502416075335,212.));
#31660=CARTESIAN_POINT('',(73.1881292872278,95.1502416075335,212.));
#31661=CARTESIAN_POINT('Origin',(73.6801683991898,93.4708376917647,212.));
#31662=CARTESIAN_POINT('',(73.6801683991898,93.4708376917647,210.));
#31663=CARTESIAN_POINT('',(73.6801683991898,93.4708376917647,210.));
#31664=CARTESIAN_POINT('',(73.6801683991898,93.4708376917647,212.));
#31665=CARTESIAN_POINT('',(73.6801683991898,93.4708376917647,212.));
#31666=CARTESIAN_POINT('',(73.6801683991898,93.4708376917647,212.));
#31667=CARTESIAN_POINT('Origin',(75.2944773987517,95.6077130999043,212.));
#31668=CARTESIAN_POINT('',(75.2944773987517,95.6077130999043,210.));
#31669=CARTESIAN_POINT('',(75.2944773987517,95.6077130999043,210.));
#31670=CARTESIAN_POINT('',(75.2944773987517,95.6077130999043,212.));
#31671=CARTESIAN_POINT('',(75.2944773987517,95.6077130999043,212.));
#31672=CARTESIAN_POINT('',(75.2944773987517,95.6077130999043,212.));
#31673=CARTESIAN_POINT('Origin',(75.5480001691776,93.8761744185935,212.));
#31674=CARTESIAN_POINT('',(75.5480001691776,93.8761744185935,210.));
#31675=CARTESIAN_POINT('',(75.5480001691776,93.8761744185935,210.));
#31676=CARTESIAN_POINT('',(75.5480001691776,93.8761744185935,212.));
#31677=CARTESIAN_POINT('',(75.5480001691776,93.8761744185935,212.));
#31678=CARTESIAN_POINT('',(75.5480001691776,93.8761744185935,212.));
#31679=CARTESIAN_POINT('Origin',(77.443994401442,95.7675855127764,212.));
#31680=CARTESIAN_POINT('',(77.443994401442,95.7675855127764,210.));
#31681=CARTESIAN_POINT('',(77.443994401442,95.7675855127764,210.));
#31682=CARTESIAN_POINT('',(77.443994401442,95.7675855127764,212.));
#31683=CARTESIAN_POINT('',(77.443994401442,95.7675855127764,212.));
#31684=CARTESIAN_POINT('',(77.443994401442,95.7675855127764,212.));
#31685=CARTESIAN_POINT('Origin',(77.4540662979833,94.0176144967593,212.));
#31686=CARTESIAN_POINT('',(77.4540662979833,94.0176144967593,210.));
#31687=CARTESIAN_POINT('',(77.4540662979833,94.0176144967593,210.));
#31688=CARTESIAN_POINT('',(77.4540662979833,94.0176144967593,212.));
#31689=CARTESIAN_POINT('',(77.4540662979833,94.0176144967593,212.));
#31690=CARTESIAN_POINT('',(77.4540662979833,94.0176144967593,212.));
#31691=CARTESIAN_POINT('Origin',(79.5948423918807,95.6267471114856,212.));
#31692=CARTESIAN_POINT('',(79.5948423918807,95.6267471114856,210.));
#31693=CARTESIAN_POINT('',(79.5948423918807,95.6267471114856,210.));
#31694=CARTESIAN_POINT('',(79.5948423918807,95.6267471114856,212.));
#31695=CARTESIAN_POINT('',(79.5948423918807,95.6267471114856,212.));
#31696=CARTESIAN_POINT('',(79.5948423918807,95.6267471114856,212.));
#31697=CARTESIAN_POINT('Origin',(79.3612673765278,93.8924049560264,212.));
#31698=CARTESIAN_POINT('',(79.3612673765278,93.8924049560264,210.));
#31699=CARTESIAN_POINT('',(79.3612673765278,93.8924049560264,210.));
#31700=CARTESIAN_POINT('',(79.3612673765278,93.8924049560264,212.));
#31701=CARTESIAN_POINT('',(79.3612673765278,93.8924049560264,212.));
#31702=CARTESIAN_POINT('',(79.3612673765278,93.8924049560264,212.));
#31703=CARTESIAN_POINT('Origin',(81.7051575604872,95.1879391553116,212.));
#31704=CARTESIAN_POINT('',(81.7051575604872,95.1879391553116,210.));
#31705=CARTESIAN_POINT('',(81.7051575604872,95.1879391553116,210.));
#31706=CARTESIAN_POINT('',(81.7051575604872,95.1879391553116,212.));
#31707=CARTESIAN_POINT('',(81.7051575604872,95.1879391553116,212.));
#31708=CARTESIAN_POINT('',(81.7051575604872,95.1879391553116,212.));
#31709=CARTESIAN_POINT('Origin',(81.2324819052264,93.5029828576814,212.));
#31710=CARTESIAN_POINT('',(81.2324819052264,93.5029828576814,210.));
#31711=CARTESIAN_POINT('',(81.2324819052264,93.5029828576814,210.));
#31712=CARTESIAN_POINT('',(81.2324819052264,93.5029828576814,212.));
#31713=CARTESIAN_POINT('',(81.2324819052264,93.5029828576814,212.));
#31714=CARTESIAN_POINT('',(81.2324819052264,93.5029828576814,212.));
#31715=CARTESIAN_POINT('Origin',(83.7338650229525,94.4597025419847,212.));
#31716=CARTESIAN_POINT('',(83.7338650229525,94.4597025419847,210.));
#31717=CARTESIAN_POINT('',(83.7338650229525,94.4597025419847,210.));
#31718=CARTESIAN_POINT('',(83.7338650229525,94.4597025419847,212.));
#31719=CARTESIAN_POINT('',(83.7338650229525,94.4597025419847,212.));
#31720=CARTESIAN_POINT('',(83.7338650229525,94.4597025419847,212.));
#31721=CARTESIAN_POINT('Origin',(83.0312888217528,92.8569278599075,212.));
#31722=CARTESIAN_POINT('',(83.0312888217528,92.8569278599075,210.));
#31723=CARTESIAN_POINT('',(83.0312888217528,92.8569278599075,210.));
#31724=CARTESIAN_POINT('',(83.0312888217528,92.8569278599075,212.));
#31725=CARTESIAN_POINT('',(83.0312888217528,92.8569278599075,212.));
#31726=CARTESIAN_POINT('',(83.0312888217528,92.8569278599075,212.));
#31727=CARTESIAN_POINT('Origin',(85.6414782961402,93.4562115688265,212.));
#31728=CARTESIAN_POINT('',(85.6414782961402,93.4562115688265,210.));
#31729=CARTESIAN_POINT('',(85.6414782961402,93.4562115688265,210.));
#31730=CARTESIAN_POINT('',(85.6414782961402,93.4562115688265,212.));
#31731=CARTESIAN_POINT('',(85.6414782961402,93.4562115688265,212.));
#31732=CARTESIAN_POINT('',(85.6414782961402,93.4562115688265,212.));
#31733=CARTESIAN_POINT('Origin',(84.7226763955895,91.9668146883597,212.));
#31734=CARTESIAN_POINT('',(84.7226763955895,91.9668146883597,210.));
#31735=CARTESIAN_POINT('',(84.7226763955895,91.9668146883597,210.));
#31736=CARTESIAN_POINT('',(84.7226763955895,91.9668146883597,212.));
#31737=CARTESIAN_POINT('',(84.7226763955895,91.9668146883597,212.));
#31738=CARTESIAN_POINT('',(84.7226763955895,91.9668146883597,212.));
#31739=CARTESIAN_POINT('Origin',(87.3908678575658,92.1969980461754,212.));
#31740=CARTESIAN_POINT('',(87.3908678575658,92.1969980461754,210.));
#31741=CARTESIAN_POINT('',(87.3908678575658,92.1969980461754,210.));
#31742=CARTESIAN_POINT('',(87.3908678575658,92.1969980461754,212.));
#31743=CARTESIAN_POINT('',(87.3908678575658,92.1969980461754,212.));
#31744=CARTESIAN_POINT('',(87.3908678575658,92.1969980461754,212.));
#31745=CARTESIAN_POINT('Origin',(86.2737236915365,90.8499683834334,212.));
#31746=CARTESIAN_POINT('',(86.2737236915365,90.8499683834334,210.));
#31747=CARTESIAN_POINT('',(86.2737236915365,90.8499683834334,210.));
#31748=CARTESIAN_POINT('',(86.2737236915365,90.8499683834334,212.));
#31749=CARTESIAN_POINT('',(86.2737236915365,90.8499683834334,212.));
#31750=CARTESIAN_POINT('',(86.2737236915365,90.8499683834334,212.));
#31751=CARTESIAN_POINT('Origin',(88.9479838293171,90.7065711329157,212.));
#31752=CARTESIAN_POINT('',(88.9479838293171,90.7065711329157,210.));
#31753=CARTESIAN_POINT('',(88.9479838293171,90.7065711329157,210.));
#31754=CARTESIAN_POINT('',(88.9479838293171,90.7065711329157,212.));
#31755=CARTESIAN_POINT('',(88.9479838293171,90.7065711329157,212.));
#31756=CARTESIAN_POINT('',(88.9479838293171,90.7065711329157,212.));
#31757=CARTESIAN_POINT('Origin',(87.6542413382684,89.5281270880603,212.));
#31758=CARTESIAN_POINT('',(87.6542413382684,89.5281270880603,210.));
#31759=CARTESIAN_POINT('',(87.6542413382684,89.5281270880603,210.));
#31760=CARTESIAN_POINT('',(87.6542413382684,89.5281270880603,212.));
#31761=CARTESIAN_POINT('',(87.6542413382684,89.5281270880603,212.));
#31762=CARTESIAN_POINT('',(87.6542413382684,89.5281270880603,212.));
#31763=CARTESIAN_POINT('Origin',(90.2825187201973,89.0139402935784,212.));
#31764=CARTESIAN_POINT('',(90.2825187201973,89.0139402935784,210.));
#31765=CARTESIAN_POINT('',(90.2825187201973,89.0139402935784,210.));
#31766=CARTESIAN_POINT('',(90.2825187201973,89.0139402935784,212.));
#31767=CARTESIAN_POINT('',(90.2825187201973,89.0139402935784,212.));
#31768=CARTESIAN_POINT('',(90.2825187201973,89.0139402935784,212.));
#31769=CARTESIAN_POINT('Origin',(88.8373591301071,88.0270189394825,212.));
#31770=CARTESIAN_POINT('',(88.8373591301071,88.0270189394825,210.));
#31771=CARTESIAN_POINT('',(88.8373591301071,88.0270189394825,210.));
#31772=CARTESIAN_POINT('',(88.8373591301071,88.0270189394825,212.));
#31773=CARTESIAN_POINT('',(88.8373591301071,88.0270189394825,212.));
#31774=CARTESIAN_POINT('',(88.8373591301071,88.0270189394825,212.));
#31775=CARTESIAN_POINT('Origin',(91.3684973265662,87.1520506621122,212.));
#31776=CARTESIAN_POINT('',(91.3684973265662,87.1520506621122,210.));
#31777=CARTESIAN_POINT('',(91.3684973265662,87.1520506621122,210.));
#31778=CARTESIAN_POINT('',(91.3684973265662,87.1520506621122,212.));
#31779=CARTESIAN_POINT('',(91.3684973265662,87.1520506621122,212.));
#31780=CARTESIAN_POINT('',(91.3684973265662,87.1520506621122,212.));
#31781=CARTESIAN_POINT('Origin',(89.8000490250111,86.3758613003269,212.));
#31782=CARTESIAN_POINT('',(89.8000490250111,86.3758613003269,210.));
#31783=CARTESIAN_POINT('',(89.8000490250111,86.3758613003269,210.));
#31784=CARTESIAN_POINT('',(89.8000490250111,86.3758613003269,212.));
#31785=CARTESIAN_POINT('',(89.8000490250111,86.3758613003269,212.));
#31786=CARTESIAN_POINT('',(89.8000490250111,86.3758613003269,212.));
#31787=CARTESIAN_POINT('Origin',(92.1847823101333,85.1571418023256,212.));
#31788=CARTESIAN_POINT('',(92.1847823101333,85.1571418023257,210.));
#31789=CARTESIAN_POINT('',(92.1847823101333,85.1571418023257,210.));
#31790=CARTESIAN_POINT('',(92.1847823101333,85.1571418023256,212.));
#31791=CARTESIAN_POINT('',(92.1847823101333,85.1571418023256,212.));
#31792=CARTESIAN_POINT('',(92.1847823101333,85.1571418023256,212.));
#31793=CARTESIAN_POINT('Origin',(90.5235733592194,84.6067920758757,212.));
#31794=CARTESIAN_POINT('',(90.5235733592194,84.6067920758757,210.));
#31795=CARTESIAN_POINT('',(90.5235733592194,84.6067920758757,210.));
#31796=CARTESIAN_POINT('',(90.5235733592194,84.6067920758757,212.));
#31797=CARTESIAN_POINT('',(90.5235733592194,84.6067920758757,212.));
#31798=CARTESIAN_POINT('',(90.5235733592194,84.6067920758757,212.));
#31799=CARTESIAN_POINT('Origin',(92.7154856122038,83.0680423459992,212.));
#31800=CARTESIAN_POINT('',(92.7154856122038,83.0680423459992,210.));
#31801=CARTESIAN_POINT('',(92.7154856122038,83.0680423459992,210.));
#31802=CARTESIAN_POINT('',(92.7154856122038,83.0680423459992,212.));
#31803=CARTESIAN_POINT('',(92.7154856122038,83.0680423459992,212.));
#31804=CARTESIAN_POINT('',(92.7154856122038,83.0680423459992,212.));
#31805=CARTESIAN_POINT('Origin',(90.9938495545636,82.7542441862965,212.));
#31806=CARTESIAN_POINT('',(90.9938495545636,82.7542441862965,210.));
#31807=CARTESIAN_POINT('',(90.9938495545636,82.7542441862965,210.));
#31808=CARTESIAN_POINT('',(90.9938495545636,82.7542441862965,212.));
#31809=CARTESIAN_POINT('',(90.9938495545636,82.7542441862965,212.));
#31810=CARTESIAN_POINT('',(90.9938495545636,82.7542441862965,212.));
#31811=CARTESIAN_POINT('Origin',(92.950277696669,80.9254142377348,212.));
#31812=CARTESIAN_POINT('',(92.950277696669,80.9254142377348,210.));
#31813=CARTESIAN_POINT('',(92.950277696669,80.9254142377348,210.));
#31814=CARTESIAN_POINT('',(92.950277696669,80.9254142377348,212.));
#31815=CARTESIAN_POINT('',(92.950277696669,80.9254142377348,212.));
#31816=CARTESIAN_POINT('',(92.950277696669,80.9254142377348,212.));
#31817=CARTESIAN_POINT('Origin',(91.2017242198324,80.8542753690178,212.));
#31818=CARTESIAN_POINT('',(91.2017242198324,80.8542753690178,210.));
#31819=CARTESIAN_POINT('',(91.2017242198324,80.8542753690178,210.));
#31820=CARTESIAN_POINT('',(91.2017242198324,80.8542753690178,212.));
#31821=CARTESIAN_POINT('',(91.2017242198324,80.8542753690178,212.));
#31822=CARTESIAN_POINT('',(91.2017242198324,80.8542753690178,212.));
#31823=CARTESIAN_POINT('Origin',(92.8845886026769,78.7709612964565,212.));
#31824=CARTESIAN_POINT('',(92.8845886026769,78.7709612964565,210.));
#31825=CARTESIAN_POINT('',(92.8845886026769,78.7709612964565,210.));
#31826=CARTESIAN_POINT('',(92.8845886026769,78.7709612964565,212.));
#31827=CARTESIAN_POINT('',(92.8845886026769,78.7709612964565,212.));
#31828=CARTESIAN_POINT('',(92.8845886026769,78.7709612964565,212.));
#31829=CARTESIAN_POINT('Origin',(91.1431513111203,78.9438663558855,212.));
#31830=CARTESIAN_POINT('',(91.1431513111203,78.9438663558855,210.));
#31831=CARTESIAN_POINT('',(91.1431513111203,78.9438663558855,210.));
#31832=CARTESIAN_POINT('',(91.1431513111203,78.9438663558855,212.));
#31833=CARTESIAN_POINT('',(91.1431513111203,78.9438663558855,212.));
#31834=CARTESIAN_POINT('',(91.1431513111203,78.9438663558855,212.));
#31835=CARTESIAN_POINT('Origin',(92.5196968937216,76.6466174980124,212.));
#31836=CARTESIAN_POINT('',(92.5196968937216,76.6466174980124,210.));
#31837=CARTESIAN_POINT('',(92.5196968937216,76.6466174980124,212.));
#31838=CARTESIAN_POINT('Origin',(77.215862801455,80.368869783441,212.));
#31839=CARTESIAN_POINT('Origin',(77.215862801455,80.368869783441,210.));
#31840=CARTESIAN_POINT('Origin',(77.215862801455,80.3688697834411,196.));
#31841=CARTESIAN_POINT('Origin',(77.215862801455,80.368869783441,200.));
#31842=CARTESIAN_POINT('',(76.2705288876953,76.4821817600082,200.));
#31843=CARTESIAN_POINT('Origin',(77.215862801455,80.368869783441,200.));
#31844=CARTESIAN_POINT('Origin',(77.215862801455,80.368869783441,210.));
#31845=CARTESIAN_POINT('',(76.2705288876953,76.4821817600082,210.));
#31846=CARTESIAN_POINT('Origin',(77.215862801455,80.368869783441,210.));
#31847=CARTESIAN_POINT('Origin',(77.215862801455,80.368869783441,212.));
#31848=CARTESIAN_POINT('',(76.2705288876953,76.4821817600082,198.1));
#31849=CARTESIAN_POINT('',(78.1611967152146,84.2555578068738,198.1));
#31850=CARTESIAN_POINT('Origin',(77.215862801455,80.368869783441,198.1));
#31851=CARTESIAN_POINT('Origin',(77.215862801455,80.368869783441,198.1));
#31852=CARTESIAN_POINT('',(76.2705288876953,76.4821817600082,212.));
#31853=CARTESIAN_POINT('Ctrl Pts',(76.8377292359511,78.8141945740679,198.312499998088));
#31854=CARTESIAN_POINT('Ctrl Pts',(77.7353213865851,78.5958790582346,198.370833331422));
#31855=CARTESIAN_POINT('Ctrl Pts',(78.3731842446541,79.2640589050045,198.429166664755));
#31856=CARTESIAN_POINT('Ctrl Pts',(79.011047102723,79.9322387517744,198.487499998088));
#31857=CARTESIAN_POINT('Ctrl Pts',(78.7513178101579,80.8187341143776,198.545833331422));
#31858=CARTESIAN_POINT('Ctrl Pts',(78.4915885175929,81.7052294769809,198.604166664755));
#31859=CARTESIAN_POINT('Ctrl Pts',(77.5939963669589,81.9235449928141,198.662499998088));
#31860=CARTESIAN_POINT('Ctrl Pts',(76.6964042163248,82.1418605086474,198.720833331422));
#31861=CARTESIAN_POINT('Ctrl Pts',(76.0585413582559,81.4736806618775,198.779166664755));
#31862=CARTESIAN_POINT('Ctrl Pts',(75.420678500187,80.8055008151076,198.837499998088));
#31863=CARTESIAN_POINT('Ctrl Pts',(75.6804077927521,79.9190054525044,198.895833331422));
#31864=CARTESIAN_POINT('Ctrl Pts',(75.9401370853171,79.0325100899012,198.954166664755));
#31865=CARTESIAN_POINT('Ctrl Pts',(76.8377292359511,78.8141945740679,199.012499998088));
#31866=CARTESIAN_POINT('Ctrl Pts',(77.7353213865851,78.5958790582346,199.070833331422));
#31867=CARTESIAN_POINT('Ctrl Pts',(78.3731842446541,79.2640589050045,199.129166664755));
#31868=CARTESIAN_POINT('Ctrl Pts',(79.011047102723,79.9322387517744,199.187499998088));
#31869=CARTESIAN_POINT('Ctrl Pts',(78.7513178101579,80.8187341143776,199.245833331422));
#31870=CARTESIAN_POINT('Ctrl Pts',(78.4915885175929,81.7052294769809,199.304166664755));
#31871=CARTESIAN_POINT('Ctrl Pts',(77.5939963669589,81.9235449928141,199.362499998088));
#31872=CARTESIAN_POINT('Ctrl Pts',(76.6964042163248,82.1418605086474,199.420833331422));
#31873=CARTESIAN_POINT('Ctrl Pts',(76.0585413582559,81.4736806618775,199.479166664755));
#31874=CARTESIAN_POINT('Ctrl Pts',(75.420678500187,80.8055008151076,199.537499998088));
#31875=CARTESIAN_POINT('Ctrl Pts',(75.6804077927521,79.9190054525044,199.595833331422));
#31876=CARTESIAN_POINT('Ctrl Pts',(75.9401370853171,79.0325100899012,199.654166664755));
#31877=CARTESIAN_POINT('Ctrl Pts',(76.8377292359511,78.8141945740679,199.712499998088));
#31878=CARTESIAN_POINT('Ctrl Pts',(77.7353213865851,78.5958790582346,199.770833331422));
#31879=CARTESIAN_POINT('Ctrl Pts',(78.3731842446541,79.2640589050045,199.829166664755));
#31880=CARTESIAN_POINT('Ctrl Pts',(79.011047102723,79.9322387517744,199.887499998088));
#31881=CARTESIAN_POINT('Ctrl Pts',(78.7513178101579,80.8187341143776,199.945833331422));
#31882=CARTESIAN_POINT('Ctrl Pts',(78.4915885175929,81.7052294769809,200.004166664755));
#31883=CARTESIAN_POINT('Ctrl Pts',(77.5939963669589,81.9235449928141,200.062499998088));
#31884=CARTESIAN_POINT('Ctrl Pts',(76.6964042163248,82.1418605086474,200.120833331422));
#31885=CARTESIAN_POINT('Ctrl Pts',(76.0585413582559,81.4736806618775,200.179166664755));
#31886=CARTESIAN_POINT('Ctrl Pts',(75.420678500187,80.8055008151076,200.237499998088));
#31887=CARTESIAN_POINT('Ctrl Pts',(75.680407792752,79.9190054525044,200.295833331422));
#31888=CARTESIAN_POINT('Ctrl Pts',(75.9401370853171,79.0325100899012,200.354166664755));
#31889=CARTESIAN_POINT('Ctrl Pts',(76.8377292359511,78.8141945740679,200.412499998088));
#31890=CARTESIAN_POINT('Ctrl Pts',(77.7353213865851,78.5958790582346,200.470833331422));
#31891=CARTESIAN_POINT('Ctrl Pts',(78.3731842446541,79.2640589050045,200.529166664755));
#31892=CARTESIAN_POINT('Ctrl Pts',(79.011047102723,79.9322387517744,200.587499998088));
#31893=CARTESIAN_POINT('Ctrl Pts',(78.7513178101579,80.8187341143776,200.645833331422));
#31894=CARTESIAN_POINT('Ctrl Pts',(78.4915885175929,81.7052294769809,200.704166664755));
#31895=CARTESIAN_POINT('Ctrl Pts',(77.5939963669589,81.9235449928141,200.762499998088));
#31896=CARTESIAN_POINT('Ctrl Pts',(76.6964042163248,82.1418605086474,200.820833331422));
#31897=CARTESIAN_POINT('Ctrl Pts',(76.0585413582559,81.4736806618775,200.879166664755));
#31898=CARTESIAN_POINT('Ctrl Pts',(75.420678500187,80.8055008151076,200.937499998088));
#31899=CARTESIAN_POINT('Ctrl Pts',(75.680407792752,79.9190054525044,200.995833331422));
#31900=CARTESIAN_POINT('Ctrl Pts',(75.9401370853171,79.0325100899012,201.054166664755));
#31901=CARTESIAN_POINT('Ctrl Pts',(76.8377292359511,78.8141945740679,201.112499998088));
#31902=CARTESIAN_POINT('Ctrl Pts',(77.7353213865851,78.5958790582346,201.170833331422));
#31903=CARTESIAN_POINT('Ctrl Pts',(78.3731842446541,79.2640589050045,201.229166664755));
#31904=CARTESIAN_POINT('Ctrl Pts',(79.011047102723,79.9322387517744,201.287499998088));
#31905=CARTESIAN_POINT('Ctrl Pts',(78.7513178101579,80.8187341143776,201.345833331422));
#31906=CARTESIAN_POINT('Ctrl Pts',(78.4915885175929,81.7052294769809,201.404166664755));
#31907=CARTESIAN_POINT('Ctrl Pts',(77.5939963669589,81.9235449928141,201.462499998088));
#31908=CARTESIAN_POINT('Ctrl Pts',(76.6964042163248,82.1418605086474,201.520833331422));
#31909=CARTESIAN_POINT('Ctrl Pts',(76.0585413582559,81.4736806618775,201.579166664755));
#31910=CARTESIAN_POINT('Ctrl Pts',(75.420678500187,80.8055008151076,201.637499998088));
#31911=CARTESIAN_POINT('Ctrl Pts',(75.680407792752,79.9190054525044,201.695833331422));
#31912=CARTESIAN_POINT('Ctrl Pts',(75.9401370853171,79.0325100899012,201.754166664755));
#31913=CARTESIAN_POINT('Ctrl Pts',(76.8377292359511,78.8141945740679,201.812499998088));
#31914=CARTESIAN_POINT('Ctrl Pts',(77.7353213865851,78.5958790582346,201.870833331422));
#31915=CARTESIAN_POINT('Ctrl Pts',(78.3731842446541,79.2640589050045,201.929166664755));
#31916=CARTESIAN_POINT('Ctrl Pts',(79.011047102723,79.9322387517744,201.987499998088));
#31917=CARTESIAN_POINT('Ctrl Pts',(78.7513178101579,80.8187341143776,202.045833331422));
#31918=CARTESIAN_POINT('Ctrl Pts',(78.4915885175929,81.7052294769808,202.104166664755));
#31919=CARTESIAN_POINT('Ctrl Pts',(77.5939963669589,81.9235449928141,202.162499998088));
#31920=CARTESIAN_POINT('Ctrl Pts',(76.6964042163248,82.1418605086474,202.220833331422));
#31921=CARTESIAN_POINT('Ctrl Pts',(76.0585413582559,81.4736806618775,202.279166664755));
#31922=CARTESIAN_POINT('Ctrl Pts',(75.420678500187,80.8055008151076,202.337499998088));
#31923=CARTESIAN_POINT('Ctrl Pts',(75.680407792752,79.9190054525044,202.395833331422));
#31924=CARTESIAN_POINT('Ctrl Pts',(75.9401370853171,79.0325100899012,202.454166664755));
#31925=CARTESIAN_POINT('Ctrl Pts',(76.8377292359511,78.8141945740679,202.512499998088));
#31926=CARTESIAN_POINT('Ctrl Pts',(77.7353213865851,78.5958790582346,202.570833331422));
#31927=CARTESIAN_POINT('Ctrl Pts',(78.3731842446541,79.2640589050045,202.629166664755));
#31928=CARTESIAN_POINT('Ctrl Pts',(79.011047102723,79.9322387517744,202.687499998088));
#31929=CARTESIAN_POINT('Ctrl Pts',(78.7513178101579,80.8187341143776,202.745833331422));
#31930=CARTESIAN_POINT('Ctrl Pts',(78.4915885175929,81.7052294769808,202.804166664755));
#31931=CARTESIAN_POINT('Ctrl Pts',(77.5939963669589,81.9235449928141,202.862499998088));
#31932=CARTESIAN_POINT('Ctrl Pts',(76.6964042163248,82.1418605086474,202.920833331422));
#31933=CARTESIAN_POINT('Ctrl Pts',(76.0585413582559,81.4736806618775,202.979166664755));
#31934=CARTESIAN_POINT('Ctrl Pts',(75.420678500187,80.8055008151076,203.037499998088));
#31935=CARTESIAN_POINT('Ctrl Pts',(75.680407792752,79.9190054525044,203.095833331422));
#31936=CARTESIAN_POINT('Ctrl Pts',(75.9401370853171,79.0325100899012,203.154166664755));
#31937=CARTESIAN_POINT('Ctrl Pts',(76.8377292359511,78.8141945740679,203.212499998088));
#31938=CARTESIAN_POINT('Ctrl Pts',(77.7353213865851,78.5958790582346,203.270833331422));
#31939=CARTESIAN_POINT('Ctrl Pts',(78.3731842446541,79.2640589050045,203.329166664755));
#31940=CARTESIAN_POINT('Ctrl Pts',(79.011047102723,79.9322387517744,203.387499998088));
#31941=CARTESIAN_POINT('Ctrl Pts',(78.7513178101579,80.8187341143776,203.445833331422));
#31942=CARTESIAN_POINT('Ctrl Pts',(78.4915885175929,81.7052294769808,203.504166664755));
#31943=CARTESIAN_POINT('Ctrl Pts',(77.5939963669589,81.9235449928141,203.562499998088));
#31944=CARTESIAN_POINT('Ctrl Pts',(76.6964042163248,82.1418605086474,203.620833331422));
#31945=CARTESIAN_POINT('Ctrl Pts',(76.0585413582559,81.4736806618775,203.679166664755));
#31946=CARTESIAN_POINT('Ctrl Pts',(75.420678500187,80.8055008151076,203.737499998088));
#31947=CARTESIAN_POINT('Ctrl Pts',(75.680407792752,79.9190054525044,203.795833331422));
#31948=CARTESIAN_POINT('Ctrl Pts',(75.9401370853171,79.0325100899012,203.854166664755));
#31949=CARTESIAN_POINT('Ctrl Pts',(76.8377292359511,78.8141945740679,203.912499998088));
#31950=CARTESIAN_POINT('Ctrl Pts',(77.7353213865851,78.5958790582346,203.970833331422));
#31951=CARTESIAN_POINT('Ctrl Pts',(78.3731842446541,79.2640589050045,204.029166664755));
#31952=CARTESIAN_POINT('Ctrl Pts',(79.011047102723,79.9322387517744,204.087499998088));
#31953=CARTESIAN_POINT('Ctrl Pts',(78.7513178101579,80.8187341143776,204.145833331422));
#31954=CARTESIAN_POINT('Ctrl Pts',(78.4915885175929,81.7052294769808,204.204166664755));
#31955=CARTESIAN_POINT('Ctrl Pts',(77.5939963669589,81.9235449928141,204.262499998088));
#31956=CARTESIAN_POINT('Ctrl Pts',(76.6964042163248,82.1418605086474,204.320833331422));
#31957=CARTESIAN_POINT('Ctrl Pts',(76.0585413582559,81.4736806618775,204.379166664755));
#31958=CARTESIAN_POINT('Ctrl Pts',(75.420678500187,80.8055008151076,204.437499998088));
#31959=CARTESIAN_POINT('Ctrl Pts',(75.680407792752,79.9190054525044,204.495833331422));
#31960=CARTESIAN_POINT('Ctrl Pts',(75.9401370853171,79.0325100899012,204.554166664755));
#31961=CARTESIAN_POINT('Ctrl Pts',(76.8377292359511,78.8141945740679,204.612499998088));
#31962=CARTESIAN_POINT('Ctrl Pts',(77.7353213865851,78.5958790582346,204.670833331422));
#31963=CARTESIAN_POINT('Ctrl Pts',(78.3731842446541,79.2640589050045,204.729166664755));
#31964=CARTESIAN_POINT('Ctrl Pts',(79.011047102723,79.9322387517744,204.787499998088));
#31965=CARTESIAN_POINT('Ctrl Pts',(78.7513178101579,80.8187341143776,204.845833331422));
#31966=CARTESIAN_POINT('Ctrl Pts',(78.4915885175929,81.7052294769808,204.904166664755));
#31967=CARTESIAN_POINT('Ctrl Pts',(77.5939963669589,81.9235449928141,204.962499998088));
#31968=CARTESIAN_POINT('Ctrl Pts',(76.6964042163248,82.1418605086474,205.020833331422));
#31969=CARTESIAN_POINT('Ctrl Pts',(76.0585413582559,81.4736806618775,205.079166664755));
#31970=CARTESIAN_POINT('Ctrl Pts',(75.420678500187,80.8055008151076,205.137499998088));
#31971=CARTESIAN_POINT('Ctrl Pts',(75.680407792752,79.9190054525044,205.195833331422));
#31972=CARTESIAN_POINT('Ctrl Pts',(75.9401370853171,79.0325100899011,205.254166664755));
#31973=CARTESIAN_POINT('Ctrl Pts',(76.8377292359511,78.8141945740679,205.312499998088));
#31974=CARTESIAN_POINT('Ctrl Pts',(77.7353213865851,78.5958790582346,205.370833331422));
#31975=CARTESIAN_POINT('Ctrl Pts',(78.3731842446541,79.2640589050045,205.429166664755));
#31976=CARTESIAN_POINT('Ctrl Pts',(79.011047102723,79.9322387517744,205.487499998088));
#31977=CARTESIAN_POINT('Ctrl Pts',(78.7513178101579,80.8187341143776,205.545833331422));
#31978=CARTESIAN_POINT('Ctrl Pts',(78.4915885175928,81.7052294769808,205.604166664755));
#31979=CARTESIAN_POINT('Ctrl Pts',(77.5939963669589,81.9235449928141,205.662499998088));
#31980=CARTESIAN_POINT('Ctrl Pts',(76.6964042163248,82.1418605086474,205.720833331422));
#31981=CARTESIAN_POINT('Ctrl Pts',(76.0585413582559,81.4736806618775,205.779166664755));
#31982=CARTESIAN_POINT('Ctrl Pts',(75.420678500187,80.8055008151076,205.837499998088));
#31983=CARTESIAN_POINT('Ctrl Pts',(75.680407792752,79.9190054525044,205.895833331421));
#31984=CARTESIAN_POINT('Ctrl Pts',(75.9401370853171,79.0325100899011,205.954166664755));
#31985=CARTESIAN_POINT('Ctrl Pts',(76.8377292359511,78.8141945740679,206.012499998088));
#31986=CARTESIAN_POINT('Ctrl Pts',(77.7353213865851,78.5958790582346,206.070833331422));
#31987=CARTESIAN_POINT('Ctrl Pts',(78.3731842446541,79.2640589050045,206.129166664755));
#31988=CARTESIAN_POINT('Ctrl Pts',(79.011047102723,79.9322387517744,206.187499998088));
#31989=CARTESIAN_POINT('Ctrl Pts',(78.7513178101579,80.8187341143776,206.245833331422));
#31990=CARTESIAN_POINT('Ctrl Pts',(78.4915885175928,81.7052294769808,206.304166664755));
#31991=CARTESIAN_POINT('Ctrl Pts',(77.5939963669589,81.9235449928141,206.362499998088));
#31992=CARTESIAN_POINT('Ctrl Pts',(76.6964042163248,82.1418605086474,206.420833331422));
#31993=CARTESIAN_POINT('Ctrl Pts',(76.0585413582559,81.4736806618775,206.479166664755));
#31994=CARTESIAN_POINT('Ctrl Pts',(75.420678500187,80.8055008151076,206.537499998088));
#31995=CARTESIAN_POINT('Ctrl Pts',(75.680407792752,79.9190054525043,206.595833331422));
#31996=CARTESIAN_POINT('Ctrl Pts',(75.9401370853171,79.0325100899011,206.654166664755));
#31997=CARTESIAN_POINT('Ctrl Pts',(76.8377292359511,78.8141945740679,206.712499998088));
#31998=CARTESIAN_POINT('Ctrl Pts',(77.7353213865851,78.5958790582346,206.770833331422));
#31999=CARTESIAN_POINT('Ctrl Pts',(78.3731842446541,79.2640589050045,206.829166664755));
#32000=CARTESIAN_POINT('Ctrl Pts',(79.011047102723,79.9322387517744,206.887499998088));
#32001=CARTESIAN_POINT('Ctrl Pts',(78.7513178101579,80.8187341143776,206.945833331422));
#32002=CARTESIAN_POINT('Ctrl Pts',(78.4915885175928,81.7052294769808,207.004166664755));
#32003=CARTESIAN_POINT('Ctrl Pts',(77.5939963669589,81.9235449928141,207.062499998088));
#32004=CARTESIAN_POINT('Ctrl Pts',(76.6964042163248,82.1418605086474,207.120833331421));
#32005=CARTESIAN_POINT('Ctrl Pts',(76.0585413582559,81.4736806618775,207.179166664755));
#32006=CARTESIAN_POINT('Ctrl Pts',(75.420678500187,80.8055008151075,207.237499998088));
#32007=CARTESIAN_POINT('Ctrl Pts',(75.680407792752,79.9190054525043,207.295833331422));
#32008=CARTESIAN_POINT('Ctrl Pts',(75.9401370853171,79.0325100899011,207.354166664755));
#32009=CARTESIAN_POINT('Ctrl Pts',(76.8377292359511,78.8141945740679,207.412499998088));
#32010=CARTESIAN_POINT('Ctrl Pts',(77.7353213865851,78.5958790582346,207.470833331422));
#32011=CARTESIAN_POINT('Ctrl Pts',(78.3731842446541,79.2640589050045,207.529166664755));
#32012=CARTESIAN_POINT('Ctrl Pts',(79.011047102723,79.9322387517744,207.587499998088));
#32013=CARTESIAN_POINT('Ctrl Pts',(78.7513178101579,80.8187341143776,207.645833331422));
#32014=CARTESIAN_POINT('Ctrl Pts',(78.4915885175928,81.7052294769808,207.704166664755));
#32015=CARTESIAN_POINT('Ctrl Pts',(77.5939963669589,81.9235449928141,207.762499998088));
#32016=CARTESIAN_POINT('Ctrl Pts',(76.6964042163248,82.1418605086474,207.820833331422));
#32017=CARTESIAN_POINT('Ctrl Pts',(76.0585413582559,81.4736806618775,207.879166664755));
#32018=CARTESIAN_POINT('Ctrl Pts',(75.420678500187,80.8055008151075,207.937499998088));
#32019=CARTESIAN_POINT('Ctrl Pts',(75.680407792752,79.9190054525043,207.995833331422));
#32020=CARTESIAN_POINT('Ctrl Pts',(75.9401370853171,79.0325100899011,208.054166664755));
#32021=CARTESIAN_POINT('Ctrl Pts',(76.8377292359511,78.8141945740679,208.112499998088));
#32022=CARTESIAN_POINT('Ctrl Pts',(77.7353213865851,78.5958790582346,208.170833331422));
#32023=CARTESIAN_POINT('Ctrl Pts',(78.3731842446541,79.2640589050045,208.229166664755));
#32024=CARTESIAN_POINT('Ctrl Pts',(79.011047102723,79.9322387517744,208.287499998088));
#32025=CARTESIAN_POINT('Ctrl Pts',(78.7513178101579,80.8187341143776,208.345833331422));
#32026=CARTESIAN_POINT('Ctrl Pts',(78.4915885175928,81.7052294769808,208.404166664755));
#32027=CARTESIAN_POINT('Ctrl Pts',(77.5939963669589,81.9235449928141,208.462499998088));
#32028=CARTESIAN_POINT('Ctrl Pts',(76.6964042163248,82.1418605086474,208.520833331422));
#32029=CARTESIAN_POINT('Ctrl Pts',(76.0585413582559,81.4736806618775,208.579166664755));
#32030=CARTESIAN_POINT('Ctrl Pts',(75.420678500187,80.8055008151075,208.637499998088));
#32031=CARTESIAN_POINT('Ctrl Pts',(75.680407792752,79.9190054525043,208.695833331422));
#32032=CARTESIAN_POINT('Ctrl Pts',(75.9401370853171,79.0325100899011,208.754166664755));
#32033=CARTESIAN_POINT('Ctrl Pts',(76.8377292359511,78.8141945740679,208.812499998088));
#32034=CARTESIAN_POINT('Ctrl Pts',(77.7353213865851,78.5958790582346,208.870833331422));
#32035=CARTESIAN_POINT('Ctrl Pts',(78.3731842446541,79.2640589050045,208.929166664755));
#32036=CARTESIAN_POINT('Ctrl Pts',(79.011047102723,79.9322387517744,208.987499998088));
#32037=CARTESIAN_POINT('Ctrl Pts',(78.7513178101579,80.8187341143776,209.045833331422));
#32038=CARTESIAN_POINT('Ctrl Pts',(78.4915885175928,81.7052294769808,209.104166664755));
#32039=CARTESIAN_POINT('Ctrl Pts',(77.5939963669589,81.9235449928141,209.162499998088));
#32040=CARTESIAN_POINT('Ctrl Pts',(76.6964042163248,82.1418605086474,209.220833331422));
#32041=CARTESIAN_POINT('Ctrl Pts',(76.0585413582559,81.4736806618775,209.279166664755));
#32042=CARTESIAN_POINT('Ctrl Pts',(75.420678500187,80.8055008151075,209.337499998088));
#32043=CARTESIAN_POINT('Ctrl Pts',(75.680407792752,79.9190054525043,209.395833331422));
#32044=CARTESIAN_POINT('Ctrl Pts',(75.9401370853171,79.0325100899011,209.454166664755));
#32045=CARTESIAN_POINT('Ctrl Pts',(76.8377292359511,78.8141945740679,209.512499998088));
#32046=CARTESIAN_POINT('Ctrl Pts',(77.7353213865851,78.5958790582346,209.570833331422));
#32047=CARTESIAN_POINT('Ctrl Pts',(78.3731842446541,79.2640589050045,209.629166664755));
#32048=CARTESIAN_POINT('Ctrl Pts',(79.011047102723,79.9322387517744,209.687499998088));
#32049=CARTESIAN_POINT('Ctrl Pts',(78.7513178101579,80.8187341143776,209.745833331422));
#32050=CARTESIAN_POINT('Ctrl Pts',(78.4915885175928,81.7052294769808,209.804166664755));
#32051=CARTESIAN_POINT('Ctrl Pts',(77.5939963669589,81.9235449928141,209.862499998088));
#32052=CARTESIAN_POINT('Ctrl Pts',(76.6964042163248,82.1418605086474,209.920833331422));
#32053=CARTESIAN_POINT('Ctrl Pts',(76.0585413582559,81.4736806618775,209.979166664755));
#32054=CARTESIAN_POINT('Ctrl Pts',(75.420678500187,80.8055008151075,210.037499998088));
#32055=CARTESIAN_POINT('Ctrl Pts',(75.680407792752,79.9190054525043,210.095833331422));
#32056=CARTESIAN_POINT('Ctrl Pts',(75.9401370853171,79.0325100899011,210.154166664755));
#32057=CARTESIAN_POINT('Ctrl Pts',(76.8377292359511,78.8141945740679,210.212499998088));
#32058=CARTESIAN_POINT('Ctrl Pts',(77.7353213865851,78.5958790582346,210.270833331422));
#32059=CARTESIAN_POINT('Ctrl Pts',(78.3731842446541,79.2640589050045,210.329166664755));
#32060=CARTESIAN_POINT('Ctrl Pts',(79.011047102723,79.9322387517744,210.387499998088));
#32061=CARTESIAN_POINT('Ctrl Pts',(78.7513178101579,80.8187341143776,210.445833331422));
#32062=CARTESIAN_POINT('Ctrl Pts',(78.4915885175928,81.7052294769808,210.504166664755));
#32063=CARTESIAN_POINT('Ctrl Pts',(77.5939963669589,81.9235449928141,210.562499998088));
#32064=CARTESIAN_POINT('Ctrl Pts',(76.6964042163248,82.1418605086474,210.620833331422));
#32065=CARTESIAN_POINT('Ctrl Pts',(76.0585413582559,81.4736806618775,210.679166664755));
#32066=CARTESIAN_POINT('Ctrl Pts',(75.420678500187,80.8055008151075,210.737499998088));
#32067=CARTESIAN_POINT('Ctrl Pts',(75.680407792752,79.9190054525043,210.795833331422));
#32068=CARTESIAN_POINT('Ctrl Pts',(75.9401370853171,79.0325100899011,210.854166664755));
#32069=CARTESIAN_POINT('Ctrl Pts',(76.8377292359511,78.8141945740679,210.912499998088));
#32070=CARTESIAN_POINT('Ctrl Pts',(77.7353213865851,78.5958790582346,210.970833331422));
#32071=CARTESIAN_POINT('Ctrl Pts',(78.3731842446541,79.2640589050045,211.029166664755));
#32072=CARTESIAN_POINT('Ctrl Pts',(79.011047102723,79.9322387517744,211.087499998088));
#32073=CARTESIAN_POINT('Ctrl Pts',(78.7513178101579,80.8187341143776,211.145833331421));
#32074=CARTESIAN_POINT('Ctrl Pts',(78.4915885175928,81.7052294769808,211.204166664755));
#32075=CARTESIAN_POINT('Ctrl Pts',(77.5939963669589,81.9235449928141,211.262499998088));
#32076=CARTESIAN_POINT('Ctrl Pts',(76.6964042163248,82.1418605086474,211.320833331422));
#32077=CARTESIAN_POINT('Ctrl Pts',(76.0585413582559,81.4736806618775,211.379166664755));
#32078=CARTESIAN_POINT('Ctrl Pts',(75.420678500187,80.8055008151075,211.437499998088));
#32079=CARTESIAN_POINT('Ctrl Pts',(75.680407792752,79.9190054525043,211.495833331422));
#32080=CARTESIAN_POINT('Ctrl Pts',(75.9401370853171,79.0325100899011,211.554166664755));
#32081=CARTESIAN_POINT('Ctrl Pts',(76.8377292359511,78.8141945740679,211.612499998088));
#32082=CARTESIAN_POINT('Ctrl Pts',(77.7353213865851,78.5958790582346,211.670833331422));
#32083=CARTESIAN_POINT('Ctrl Pts',(78.3731842446541,79.2640589050045,211.729166664755));
#32084=CARTESIAN_POINT('Ctrl Pts',(79.011047102723,79.9322387517744,211.787499998088));
#32085=CARTESIAN_POINT('Ctrl Pts',(78.7513178101579,80.8187341143776,211.845833331422));
#32086=CARTESIAN_POINT('Ctrl Pts',(78.4915885175928,81.7052294769808,211.904166664755));
#32087=CARTESIAN_POINT('Ctrl Pts',(77.5939963669588,81.9235449928141,211.962499998088));
#32088=CARTESIAN_POINT('Ctrl Pts',(76.6964042163248,82.1418605086474,212.020833331422));
#32089=CARTESIAN_POINT('Ctrl Pts',(76.0585413582559,81.4736806618775,212.079166664755));
#32090=CARTESIAN_POINT('Ctrl Pts',(75.420678500187,80.8055008151075,212.137499998088));
#32091=CARTESIAN_POINT('Ctrl Pts',(75.680407792752,79.9190054525043,212.195833331422));
#32092=CARTESIAN_POINT('Ctrl Pts',(75.9401370853171,79.0325100899011,212.254166664755));
#32093=CARTESIAN_POINT('Ctrl Pts',(76.8377292359511,78.8141945740678,212.312499998088));
#32094=CARTESIAN_POINT('Ctrl Pts',(76.9272727088509,79.1823476029926,198.093749999044));
#32095=CARTESIAN_POINT('Ctrl Pts',(77.6123116091322,79.0157300353421,198.152083332377));
#32096=CARTESIAN_POINT('Ctrl Pts',(78.099126105575,79.5256823417411,198.210416665711));
#32097=CARTESIAN_POINT('Ctrl Pts',(78.5859406020177,80.0356346481401,198.268749999044));
#32098=CARTESIAN_POINT('Ctrl Pts',(78.3877161981791,80.7122045221895,198.327083332377));
#32099=CARTESIAN_POINT('Ctrl Pts',(78.1894917943405,81.388774396239,198.385416665711));
#32100=CARTESIAN_POINT('Ctrl Pts',(77.5044528940591,81.5553919638894,198.443749999044));
#32101=CARTESIAN_POINT('Ctrl Pts',(76.8194139937778,81.7220095315399,198.502083332377));
#32102=CARTESIAN_POINT('Ctrl Pts',(76.332599497335,81.2120572251409,198.560416665711));
#32103=CARTESIAN_POINT('Ctrl Pts',(75.8457850008923,80.702104918742,198.618749999044));
#32104=CARTESIAN_POINT('Ctrl Pts',(76.0440094047309,80.0255350446925,198.677083332377));
#32105=CARTESIAN_POINT('Ctrl Pts',(76.2422338085695,79.348965170643,198.735416665711));
#32106=CARTESIAN_POINT('Ctrl Pts',(76.9272727088509,79.1823476029926,198.793749999044));
#32107=CARTESIAN_POINT('Ctrl Pts',(77.6123116091322,79.0157300353421,198.852083332378));
#32108=CARTESIAN_POINT('Ctrl Pts',(78.099126105575,79.5256823417411,198.910416665711));
#32109=CARTESIAN_POINT('Ctrl Pts',(78.5859406020177,80.0356346481401,198.968749999044));
#32110=CARTESIAN_POINT('Ctrl Pts',(78.3877161981791,80.7122045221895,199.027083332377));
#32111=CARTESIAN_POINT('Ctrl Pts',(78.1894917943405,81.388774396239,199.085416665711));
#32112=CARTESIAN_POINT('Ctrl Pts',(77.5044528940591,81.5553919638894,199.143749999044));
#32113=CARTESIAN_POINT('Ctrl Pts',(76.8194139937778,81.7220095315399,199.202083332377));
#32114=CARTESIAN_POINT('Ctrl Pts',(76.332599497335,81.2120572251409,199.260416665711));
#32115=CARTESIAN_POINT('Ctrl Pts',(75.8457850008923,80.702104918742,199.318749999044));
#32116=CARTESIAN_POINT('Ctrl Pts',(76.0440094047309,80.0255350446925,199.377083332377));
#32117=CARTESIAN_POINT('Ctrl Pts',(76.2422338085695,79.348965170643,199.435416665711));
#32118=CARTESIAN_POINT('Ctrl Pts',(76.9272727088509,79.1823476029926,199.493749999044));
#32119=CARTESIAN_POINT('Ctrl Pts',(77.6123116091322,79.0157300353421,199.552083332377));
#32120=CARTESIAN_POINT('Ctrl Pts',(78.099126105575,79.5256823417411,199.610416665711));
#32121=CARTESIAN_POINT('Ctrl Pts',(78.5859406020177,80.0356346481401,199.668749999044));
#32122=CARTESIAN_POINT('Ctrl Pts',(78.3877161981791,80.7122045221895,199.727083332377));
#32123=CARTESIAN_POINT('Ctrl Pts',(78.1894917943405,81.388774396239,199.785416665711));
#32124=CARTESIAN_POINT('Ctrl Pts',(77.5044528940591,81.5553919638894,199.843749999044));
#32125=CARTESIAN_POINT('Ctrl Pts',(76.8194139937778,81.7220095315399,199.902083332377));
#32126=CARTESIAN_POINT('Ctrl Pts',(76.332599497335,81.2120572251409,199.960416665711));
#32127=CARTESIAN_POINT('Ctrl Pts',(75.8457850008923,80.702104918742,200.018749999044));
#32128=CARTESIAN_POINT('Ctrl Pts',(76.0440094047309,80.0255350446925,200.077083332377));
#32129=CARTESIAN_POINT('Ctrl Pts',(76.2422338085695,79.348965170643,200.135416665711));
#32130=CARTESIAN_POINT('Ctrl Pts',(76.9272727088508,79.1823476029926,200.193749999044));
#32131=CARTESIAN_POINT('Ctrl Pts',(77.6123116091322,79.0157300353421,200.252083332377));
#32132=CARTESIAN_POINT('Ctrl Pts',(78.099126105575,79.5256823417411,200.310416665711));
#32133=CARTESIAN_POINT('Ctrl Pts',(78.5859406020177,80.0356346481401,200.368749999044));
#32134=CARTESIAN_POINT('Ctrl Pts',(78.3877161981791,80.7122045221895,200.427083332377));
#32135=CARTESIAN_POINT('Ctrl Pts',(78.1894917943405,81.388774396239,200.485416665711));
#32136=CARTESIAN_POINT('Ctrl Pts',(77.5044528940591,81.5553919638894,200.543749999044));
#32137=CARTESIAN_POINT('Ctrl Pts',(76.8194139937778,81.7220095315399,200.602083332377));
#32138=CARTESIAN_POINT('Ctrl Pts',(76.332599497335,81.2120572251409,200.660416665711));
#32139=CARTESIAN_POINT('Ctrl Pts',(75.8457850008923,80.702104918742,200.718749999044));
#32140=CARTESIAN_POINT('Ctrl Pts',(76.0440094047309,80.0255350446925,200.777083332377));
#32141=CARTESIAN_POINT('Ctrl Pts',(76.2422338085695,79.348965170643,200.835416665711));
#32142=CARTESIAN_POINT('Ctrl Pts',(76.9272727088508,79.1823476029926,200.893749999044));
#32143=CARTESIAN_POINT('Ctrl Pts',(77.6123116091322,79.0157300353421,200.952083332377));
#32144=CARTESIAN_POINT('Ctrl Pts',(78.099126105575,79.5256823417411,201.010416665711));
#32145=CARTESIAN_POINT('Ctrl Pts',(78.5859406020177,80.0356346481401,201.068749999044));
#32146=CARTESIAN_POINT('Ctrl Pts',(78.3877161981791,80.7122045221895,201.127083332377));
#32147=CARTESIAN_POINT('Ctrl Pts',(78.1894917943405,81.388774396239,201.185416665711));
#32148=CARTESIAN_POINT('Ctrl Pts',(77.5044528940591,81.5553919638894,201.243749999044));
#32149=CARTESIAN_POINT('Ctrl Pts',(76.8194139937778,81.7220095315399,201.302083332377));
#32150=CARTESIAN_POINT('Ctrl Pts',(76.332599497335,81.2120572251409,201.360416665711));
#32151=CARTESIAN_POINT('Ctrl Pts',(75.8457850008923,80.702104918742,201.418749999044));
#32152=CARTESIAN_POINT('Ctrl Pts',(76.0440094047309,80.0255350446925,201.477083332377));
#32153=CARTESIAN_POINT('Ctrl Pts',(76.2422338085695,79.348965170643,201.535416665711));
#32154=CARTESIAN_POINT('Ctrl Pts',(76.9272727088508,79.1823476029926,201.593749999044));
#32155=CARTESIAN_POINT('Ctrl Pts',(77.6123116091322,79.0157300353421,201.652083332377));
#32156=CARTESIAN_POINT('Ctrl Pts',(78.099126105575,79.5256823417411,201.710416665711));
#32157=CARTESIAN_POINT('Ctrl Pts',(78.5859406020177,80.0356346481401,201.768749999044));
#32158=CARTESIAN_POINT('Ctrl Pts',(78.3877161981791,80.7122045221895,201.827083332377));
#32159=CARTESIAN_POINT('Ctrl Pts',(78.1894917943405,81.388774396239,201.885416665711));
#32160=CARTESIAN_POINT('Ctrl Pts',(77.5044528940591,81.5553919638894,201.943749999044));
#32161=CARTESIAN_POINT('Ctrl Pts',(76.8194139937778,81.7220095315399,202.002083332377));
#32162=CARTESIAN_POINT('Ctrl Pts',(76.332599497335,81.2120572251409,202.060416665711));
#32163=CARTESIAN_POINT('Ctrl Pts',(75.8457850008923,80.702104918742,202.118749999044));
#32164=CARTESIAN_POINT('Ctrl Pts',(76.0440094047309,80.0255350446925,202.177083332377));
#32165=CARTESIAN_POINT('Ctrl Pts',(76.2422338085695,79.348965170643,202.235416665711));
#32166=CARTESIAN_POINT('Ctrl Pts',(76.9272727088508,79.1823476029926,202.293749999044));
#32167=CARTESIAN_POINT('Ctrl Pts',(77.6123116091322,79.0157300353421,202.352083332377));
#32168=CARTESIAN_POINT('Ctrl Pts',(78.099126105575,79.5256823417411,202.410416665711));
#32169=CARTESIAN_POINT('Ctrl Pts',(78.5859406020177,80.0356346481401,202.468749999044));
#32170=CARTESIAN_POINT('Ctrl Pts',(78.3877161981791,80.7122045221895,202.527083332377));
#32171=CARTESIAN_POINT('Ctrl Pts',(78.1894917943405,81.388774396239,202.585416665711));
#32172=CARTESIAN_POINT('Ctrl Pts',(77.5044528940591,81.5553919638894,202.643749999044));
#32173=CARTESIAN_POINT('Ctrl Pts',(76.8194139937778,81.7220095315399,202.702083332377));
#32174=CARTESIAN_POINT('Ctrl Pts',(76.332599497335,81.2120572251409,202.760416665711));
#32175=CARTESIAN_POINT('Ctrl Pts',(75.8457850008923,80.7021049187419,202.818749999044));
#32176=CARTESIAN_POINT('Ctrl Pts',(76.0440094047309,80.0255350446925,202.877083332377));
#32177=CARTESIAN_POINT('Ctrl Pts',(76.2422338085695,79.348965170643,202.935416665711));
#32178=CARTESIAN_POINT('Ctrl Pts',(76.9272727088508,79.1823476029926,202.993749999044));
#32179=CARTESIAN_POINT('Ctrl Pts',(77.6123116091322,79.0157300353421,203.052083332377));
#32180=CARTESIAN_POINT('Ctrl Pts',(78.099126105575,79.5256823417411,203.110416665711));
#32181=CARTESIAN_POINT('Ctrl Pts',(78.5859406020177,80.0356346481401,203.168749999044));
#32182=CARTESIAN_POINT('Ctrl Pts',(78.3877161981791,80.7122045221895,203.227083332377));
#32183=CARTESIAN_POINT('Ctrl Pts',(78.1894917943405,81.388774396239,203.285416665711));
#32184=CARTESIAN_POINT('Ctrl Pts',(77.5044528940591,81.5553919638894,203.343749999044));
#32185=CARTESIAN_POINT('Ctrl Pts',(76.8194139937778,81.7220095315399,203.402083332378));
#32186=CARTESIAN_POINT('Ctrl Pts',(76.332599497335,81.2120572251409,203.460416665711));
#32187=CARTESIAN_POINT('Ctrl Pts',(75.8457850008923,80.7021049187419,203.518749999044));
#32188=CARTESIAN_POINT('Ctrl Pts',(76.0440094047309,80.0255350446925,203.577083332377));
#32189=CARTESIAN_POINT('Ctrl Pts',(76.2422338085695,79.348965170643,203.635416665711));
#32190=CARTESIAN_POINT('Ctrl Pts',(76.9272727088508,79.1823476029926,203.693749999044));
#32191=CARTESIAN_POINT('Ctrl Pts',(77.6123116091322,79.0157300353421,203.752083332377));
#32192=CARTESIAN_POINT('Ctrl Pts',(78.099126105575,79.5256823417411,203.810416665711));
#32193=CARTESIAN_POINT('Ctrl Pts',(78.5859406020177,80.03563464814,203.868749999044));
#32194=CARTESIAN_POINT('Ctrl Pts',(78.3877161981791,80.7122045221895,203.927083332377));
#32195=CARTESIAN_POINT('Ctrl Pts',(78.1894917943405,81.388774396239,203.985416665711));
#32196=CARTESIAN_POINT('Ctrl Pts',(77.5044528940591,81.5553919638894,204.043749999044));
#32197=CARTESIAN_POINT('Ctrl Pts',(76.8194139937778,81.7220095315399,204.102083332377));
#32198=CARTESIAN_POINT('Ctrl Pts',(76.332599497335,81.2120572251409,204.160416665711));
#32199=CARTESIAN_POINT('Ctrl Pts',(75.8457850008923,80.7021049187419,204.218749999044));
#32200=CARTESIAN_POINT('Ctrl Pts',(76.0440094047309,80.0255350446925,204.277083332377));
#32201=CARTESIAN_POINT('Ctrl Pts',(76.2422338085695,79.348965170643,204.335416665711));
#32202=CARTESIAN_POINT('Ctrl Pts',(76.9272727088508,79.1823476029926,204.393749999044));
#32203=CARTESIAN_POINT('Ctrl Pts',(77.6123116091322,79.0157300353421,204.452083332377));
#32204=CARTESIAN_POINT('Ctrl Pts',(78.099126105575,79.5256823417411,204.510416665711));
#32205=CARTESIAN_POINT('Ctrl Pts',(78.5859406020177,80.03563464814,204.568749999044));
#32206=CARTESIAN_POINT('Ctrl Pts',(78.3877161981791,80.7122045221895,204.627083332377));
#32207=CARTESIAN_POINT('Ctrl Pts',(78.1894917943405,81.388774396239,204.685416665711));
#32208=CARTESIAN_POINT('Ctrl Pts',(77.5044528940591,81.5553919638894,204.743749999044));
#32209=CARTESIAN_POINT('Ctrl Pts',(76.8194139937778,81.7220095315399,204.802083332378));
#32210=CARTESIAN_POINT('Ctrl Pts',(76.332599497335,81.2120572251409,204.860416665711));
#32211=CARTESIAN_POINT('Ctrl Pts',(75.8457850008923,80.7021049187419,204.918749999044));
#32212=CARTESIAN_POINT('Ctrl Pts',(76.0440094047309,80.0255350446925,204.977083332377));
#32213=CARTESIAN_POINT('Ctrl Pts',(76.2422338085695,79.348965170643,205.035416665711));
#32214=CARTESIAN_POINT('Ctrl Pts',(76.9272727088508,79.1823476029926,205.093749999044));
#32215=CARTESIAN_POINT('Ctrl Pts',(77.6123116091322,79.0157300353421,205.152083332377));
#32216=CARTESIAN_POINT('Ctrl Pts',(78.099126105575,79.5256823417411,205.210416665711));
#32217=CARTESIAN_POINT('Ctrl Pts',(78.5859406020177,80.03563464814,205.268749999044));
#32218=CARTESIAN_POINT('Ctrl Pts',(78.3877161981791,80.7122045221895,205.327083332377));
#32219=CARTESIAN_POINT('Ctrl Pts',(78.1894917943405,81.388774396239,205.385416665711));
#32220=CARTESIAN_POINT('Ctrl Pts',(77.5044528940591,81.5553919638894,205.443749999044));
#32221=CARTESIAN_POINT('Ctrl Pts',(76.8194139937778,81.7220095315399,205.502083332377));
#32222=CARTESIAN_POINT('Ctrl Pts',(76.332599497335,81.2120572251409,205.560416665711));
#32223=CARTESIAN_POINT('Ctrl Pts',(75.8457850008923,80.7021049187419,205.618749999044));
#32224=CARTESIAN_POINT('Ctrl Pts',(76.0440094047309,80.0255350446925,205.677083332377));
#32225=CARTESIAN_POINT('Ctrl Pts',(76.2422338085695,79.348965170643,205.735416665711));
#32226=CARTESIAN_POINT('Ctrl Pts',(76.9272727088508,79.1823476029926,205.793749999044));
#32227=CARTESIAN_POINT('Ctrl Pts',(77.6123116091322,79.0157300353421,205.852083332377));
#32228=CARTESIAN_POINT('Ctrl Pts',(78.099126105575,79.5256823417411,205.910416665711));
#32229=CARTESIAN_POINT('Ctrl Pts',(78.5859406020177,80.03563464814,205.968749999044));
#32230=CARTESIAN_POINT('Ctrl Pts',(78.3877161981791,80.7122045221895,206.027083332377));
#32231=CARTESIAN_POINT('Ctrl Pts',(78.1894917943405,81.3887743962389,206.085416665711));
#32232=CARTESIAN_POINT('Ctrl Pts',(77.5044528940591,81.5553919638894,206.143749999044));
#32233=CARTESIAN_POINT('Ctrl Pts',(76.8194139937778,81.7220095315399,206.202083332377));
#32234=CARTESIAN_POINT('Ctrl Pts',(76.332599497335,81.2120572251409,206.260416665711));
#32235=CARTESIAN_POINT('Ctrl Pts',(75.8457850008923,80.7021049187419,206.318749999044));
#32236=CARTESIAN_POINT('Ctrl Pts',(76.0440094047309,80.0255350446925,206.377083332377));
#32237=CARTESIAN_POINT('Ctrl Pts',(76.2422338085695,79.348965170643,206.435416665711));
#32238=CARTESIAN_POINT('Ctrl Pts',(76.9272727088508,79.1823476029926,206.493749999044));
#32239=CARTESIAN_POINT('Ctrl Pts',(77.6123116091322,79.0157300353421,206.552083332377));
#32240=CARTESIAN_POINT('Ctrl Pts',(78.099126105575,79.5256823417411,206.610416665711));
#32241=CARTESIAN_POINT('Ctrl Pts',(78.5859406020177,80.03563464814,206.668749999044));
#32242=CARTESIAN_POINT('Ctrl Pts',(78.3877161981791,80.7122045221895,206.727083332377));
#32243=CARTESIAN_POINT('Ctrl Pts',(78.1894917943405,81.3887743962389,206.785416665711));
#32244=CARTESIAN_POINT('Ctrl Pts',(77.5044528940591,81.5553919638894,206.843749999044));
#32245=CARTESIAN_POINT('Ctrl Pts',(76.8194139937778,81.7220095315399,206.902083332377));
#32246=CARTESIAN_POINT('Ctrl Pts',(76.332599497335,81.2120572251409,206.960416665711));
#32247=CARTESIAN_POINT('Ctrl Pts',(75.8457850008923,80.7021049187419,207.018749999044));
#32248=CARTESIAN_POINT('Ctrl Pts',(76.0440094047309,80.0255350446925,207.077083332377));
#32249=CARTESIAN_POINT('Ctrl Pts',(76.2422338085695,79.348965170643,207.135416665711));
#32250=CARTESIAN_POINT('Ctrl Pts',(76.9272727088508,79.1823476029926,207.193749999044));
#32251=CARTESIAN_POINT('Ctrl Pts',(77.6123116091322,79.0157300353421,207.252083332377));
#32252=CARTESIAN_POINT('Ctrl Pts',(78.099126105575,79.5256823417411,207.310416665711));
#32253=CARTESIAN_POINT('Ctrl Pts',(78.5859406020177,80.03563464814,207.368749999044));
#32254=CARTESIAN_POINT('Ctrl Pts',(78.3877161981791,80.7122045221895,207.427083332377));
#32255=CARTESIAN_POINT('Ctrl Pts',(78.1894917943405,81.3887743962389,207.485416665711));
#32256=CARTESIAN_POINT('Ctrl Pts',(77.5044528940591,81.5553919638894,207.543749999044));
#32257=CARTESIAN_POINT('Ctrl Pts',(76.8194139937778,81.7220095315399,207.602083332378));
#32258=CARTESIAN_POINT('Ctrl Pts',(76.332599497335,81.2120572251409,207.660416665711));
#32259=CARTESIAN_POINT('Ctrl Pts',(75.8457850008923,80.7021049187419,207.718749999044));
#32260=CARTESIAN_POINT('Ctrl Pts',(76.0440094047309,80.0255350446925,207.777083332377));
#32261=CARTESIAN_POINT('Ctrl Pts',(76.2422338085695,79.348965170643,207.835416665711));
#32262=CARTESIAN_POINT('Ctrl Pts',(76.9272727088508,79.1823476029926,207.893749999044));
#32263=CARTESIAN_POINT('Ctrl Pts',(77.6123116091322,79.0157300353421,207.952083332377));
#32264=CARTESIAN_POINT('Ctrl Pts',(78.0991261055749,79.5256823417411,208.010416665711));
#32265=CARTESIAN_POINT('Ctrl Pts',(78.5859406020177,80.03563464814,208.068749999044));
#32266=CARTESIAN_POINT('Ctrl Pts',(78.3877161981791,80.7122045221895,208.127083332377));
#32267=CARTESIAN_POINT('Ctrl Pts',(78.1894917943405,81.3887743962389,208.185416665711));
#32268=CARTESIAN_POINT('Ctrl Pts',(77.5044528940591,81.5553919638894,208.243749999044));
#32269=CARTESIAN_POINT('Ctrl Pts',(76.8194139937778,81.7220095315399,208.302083332377));
#32270=CARTESIAN_POINT('Ctrl Pts',(76.332599497335,81.2120572251409,208.360416665711));
#32271=CARTESIAN_POINT('Ctrl Pts',(75.8457850008923,80.7021049187419,208.418749999044));
#32272=CARTESIAN_POINT('Ctrl Pts',(76.0440094047309,80.0255350446925,208.477083332377));
#32273=CARTESIAN_POINT('Ctrl Pts',(76.2422338085695,79.348965170643,208.535416665711));
#32274=CARTESIAN_POINT('Ctrl Pts',(76.9272727088508,79.1823476029926,208.593749999044));
#32275=CARTESIAN_POINT('Ctrl Pts',(77.6123116091322,79.0157300353421,208.652083332377));
#32276=CARTESIAN_POINT('Ctrl Pts',(78.0991261055749,79.5256823417411,208.710416665711));
#32277=CARTESIAN_POINT('Ctrl Pts',(78.5859406020177,80.03563464814,208.768749999044));
#32278=CARTESIAN_POINT('Ctrl Pts',(78.3877161981791,80.7122045221895,208.827083332377));
#32279=CARTESIAN_POINT('Ctrl Pts',(78.1894917943405,81.3887743962389,208.885416665711));
#32280=CARTESIAN_POINT('Ctrl Pts',(77.5044528940591,81.5553919638894,208.943749999044));
#32281=CARTESIAN_POINT('Ctrl Pts',(76.8194139937778,81.7220095315399,209.002083332377));
#32282=CARTESIAN_POINT('Ctrl Pts',(76.332599497335,81.2120572251409,209.060416665711));
#32283=CARTESIAN_POINT('Ctrl Pts',(75.8457850008923,80.7021049187419,209.118749999044));
#32284=CARTESIAN_POINT('Ctrl Pts',(76.0440094047309,80.0255350446925,209.177083332377));
#32285=CARTESIAN_POINT('Ctrl Pts',(76.2422338085695,79.348965170643,209.235416665711));
#32286=CARTESIAN_POINT('Ctrl Pts',(76.9272727088508,79.1823476029926,209.293749999044));
#32287=CARTESIAN_POINT('Ctrl Pts',(77.6123116091322,79.0157300353421,209.352083332377));
#32288=CARTESIAN_POINT('Ctrl Pts',(78.0991261055749,79.5256823417411,209.410416665711));
#32289=CARTESIAN_POINT('Ctrl Pts',(78.5859406020177,80.03563464814,209.468749999044));
#32290=CARTESIAN_POINT('Ctrl Pts',(78.3877161981791,80.7122045221895,209.527083332377));
#32291=CARTESIAN_POINT('Ctrl Pts',(78.1894917943405,81.3887743962389,209.585416665711));
#32292=CARTESIAN_POINT('Ctrl Pts',(77.5044528940591,81.5553919638894,209.643749999044));
#32293=CARTESIAN_POINT('Ctrl Pts',(76.8194139937778,81.7220095315399,209.702083332377));
#32294=CARTESIAN_POINT('Ctrl Pts',(76.332599497335,81.2120572251409,209.760416665711));
#32295=CARTESIAN_POINT('Ctrl Pts',(75.8457850008923,80.7021049187419,209.818749999044));
#32296=CARTESIAN_POINT('Ctrl Pts',(76.0440094047309,80.0255350446925,209.877083332377));
#32297=CARTESIAN_POINT('Ctrl Pts',(76.2422338085695,79.348965170643,209.935416665711));
#32298=CARTESIAN_POINT('Ctrl Pts',(76.9272727088508,79.1823476029926,209.993749999044));
#32299=CARTESIAN_POINT('Ctrl Pts',(77.6123116091322,79.0157300353421,210.052083332377));
#32300=CARTESIAN_POINT('Ctrl Pts',(78.0991261055749,79.5256823417411,210.110416665711));
#32301=CARTESIAN_POINT('Ctrl Pts',(78.5859406020177,80.03563464814,210.168749999044));
#32302=CARTESIAN_POINT('Ctrl Pts',(78.3877161981791,80.7122045221895,210.227083332377));
#32303=CARTESIAN_POINT('Ctrl Pts',(78.1894917943405,81.3887743962389,210.285416665711));
#32304=CARTESIAN_POINT('Ctrl Pts',(77.5044528940591,81.5553919638894,210.343749999044));
#32305=CARTESIAN_POINT('Ctrl Pts',(76.8194139937778,81.7220095315399,210.402083332377));
#32306=CARTESIAN_POINT('Ctrl Pts',(76.332599497335,81.2120572251409,210.460416665711));
#32307=CARTESIAN_POINT('Ctrl Pts',(75.8457850008923,80.7021049187419,210.518749999044));
#32308=CARTESIAN_POINT('Ctrl Pts',(76.0440094047309,80.0255350446925,210.577083332377));
#32309=CARTESIAN_POINT('Ctrl Pts',(76.2422338085695,79.348965170643,210.635416665711));
#32310=CARTESIAN_POINT('Ctrl Pts',(76.9272727088508,79.1823476029926,210.693749999044));
#32311=CARTESIAN_POINT('Ctrl Pts',(77.6123116091322,79.0157300353421,210.752083332377));
#32312=CARTESIAN_POINT('Ctrl Pts',(78.0991261055749,79.5256823417411,210.810416665711));
#32313=CARTESIAN_POINT('Ctrl Pts',(78.5859406020177,80.03563464814,210.868749999044));
#32314=CARTESIAN_POINT('Ctrl Pts',(78.3877161981791,80.7122045221895,210.927083332377));
#32315=CARTESIAN_POINT('Ctrl Pts',(78.1894917943405,81.3887743962389,210.985416665711));
#32316=CARTESIAN_POINT('Ctrl Pts',(77.5044528940591,81.5553919638894,211.043749999044));
#32317=CARTESIAN_POINT('Ctrl Pts',(76.8194139937778,81.7220095315399,211.102083332377));
#32318=CARTESIAN_POINT('Ctrl Pts',(76.332599497335,81.2120572251409,211.160416665711));
#32319=CARTESIAN_POINT('Ctrl Pts',(75.8457850008923,80.7021049187419,211.218749999044));
#32320=CARTESIAN_POINT('Ctrl Pts',(76.0440094047309,80.0255350446925,211.277083332377));
#32321=CARTESIAN_POINT('Ctrl Pts',(76.2422338085695,79.348965170643,211.335416665711));
#32322=CARTESIAN_POINT('Ctrl Pts',(76.9272727088508,79.1823476029925,211.393749999044));
#32323=CARTESIAN_POINT('Ctrl Pts',(77.6123116091322,79.0157300353421,211.452083332377));
#32324=CARTESIAN_POINT('Ctrl Pts',(78.0991261055749,79.525682341741,211.510416665711));
#32325=CARTESIAN_POINT('Ctrl Pts',(78.5859406020177,80.03563464814,211.568749999044));
#32326=CARTESIAN_POINT('Ctrl Pts',(78.3877161981791,80.7122045221895,211.627083332377));
#32327=CARTESIAN_POINT('Ctrl Pts',(78.1894917943405,81.3887743962389,211.685416665711));
#32328=CARTESIAN_POINT('Ctrl Pts',(77.5044528940591,81.5553919638894,211.743749999044));
#32329=CARTESIAN_POINT('Ctrl Pts',(76.8194139937778,81.7220095315399,211.802083332377));
#32330=CARTESIAN_POINT('Ctrl Pts',(76.332599497335,81.2120572251409,211.860416665711));
#32331=CARTESIAN_POINT('Ctrl Pts',(75.8457850008923,80.7021049187419,211.918749999044));
#32332=CARTESIAN_POINT('Ctrl Pts',(76.0440094047309,80.0255350446925,211.977083332377));
#32333=CARTESIAN_POINT('Ctrl Pts',(76.2422338085695,79.348965170643,212.035416665711));
#32334=CARTESIAN_POINT('Ctrl Pts',(76.9272727088508,79.1823476029925,212.093749999044));
#32335=CARTESIAN_POINT('',(76.882500972401,78.9982710885302,198.203124998566));
#32336=CARTESIAN_POINT('Ctrl Pts',(76.8377292359513,78.8141945740678,210.212499998088));
#32337=CARTESIAN_POINT('Ctrl Pts',(76.8592837264637,78.8089520151713,210.213900796078));
#32338=CARTESIAN_POINT('Ctrl Pts',(76.880961717515,78.8041541885631,210.215319353774));
#32339=CARTESIAN_POINT('Ctrl Pts',(77.1109710529602,78.7582549040848,210.230473284417));
#32340=CARTESIAN_POINT('Ctrl Pts',(77.3253356333712,78.7585744965251,210.245480033072));
#32341=CARTESIAN_POINT('Ctrl Pts',(77.737156513034,78.8419446966982,210.276006491287));
#32342=CARTESIAN_POINT('Ctrl Pts',(77.9310168188607,78.9225572032128,210.291224585572));
#32343=CARTESIAN_POINT('Ctrl Pts',(78.2736586329449,79.1512256470014,210.319889078168));
#32344=CARTESIAN_POINT('Ctrl Pts',(78.4200352333683,79.2957652859252,210.332220462871));
#32345=CARTESIAN_POINT('Ctrl Pts',(78.6562261084613,79.6401624127909,210.360691567112));
#32346=CARTESIAN_POINT('Ctrl Pts',(78.7405435897384,79.8387937024458,210.376217822852));
#32347=CARTESIAN_POINT('Ctrl Pts',(78.8245801400631,80.2494216513298,210.406759430467));
#32348=CARTESIAN_POINT('Ctrl Pts',(78.8266170207136,80.4568794737522,210.42149314287));
#32349=CARTESIAN_POINT('Ctrl Pts',(78.7514066787451,80.8646581040814,210.449088627304));
#32350=CARTESIAN_POINT('Ctrl Pts',(78.6735850260427,81.0608017958442,210.462121129468));
#32351=CARTESIAN_POINT('Ctrl Pts',(78.4457682921329,81.4137915170909,210.49190959644));
#32352=CARTESIAN_POINT('Ctrl Pts',(78.2973923216281,81.5667079258093,210.507434575797));
#32353=CARTESIAN_POINT('Ctrl Pts',(77.9562152832965,81.8017739525743,210.537264556535));
#32354=CARTESIAN_POINT('Ctrl Pts',(77.7684344389729,81.8840950144953,210.551102454384));
#32355=CARTESIAN_POINT('Ctrl Pts',(77.3633866713352,81.9761357117601,210.577558753721));
#32356=CARTESIAN_POINT('Ctrl Pts',(77.1491313794517,81.9814958308773,210.592441411551));
#32357=CARTESIAN_POINT('Ctrl Pts',(76.7347602170159,81.9090030673567,210.622923321041));
#32358=CARTESIAN_POINT('Ctrl Pts',(76.538357199793,81.8332707638251,210.638219289857));
#32359=CARTESIAN_POINT('Ctrl Pts',(76.1900091522267,81.6134527075351,210.667101629704));
#32360=CARTESIAN_POINT('Ctrl Pts',(76.0403356127154,81.4731739150612,210.679516301547));
#32361=CARTESIAN_POINT('Ctrl Pts',(75.7950649908508,81.1351846320785,210.707689871198));
#32362=CARTESIAN_POINT('Ctrl Pts',(75.7053556877558,80.9382903200132,210.723185975568));
#32363=CARTESIAN_POINT('Ctrl Pts',(75.610609672748,80.5289041559014,210.753824153838));
#32364=CARTESIAN_POINT('Ctrl Pts',(75.6033512671848,80.3210446090024,210.768676309564));
#32365=CARTESIAN_POINT('Ctrl Pts',(75.6683527121138,79.9124473561696,210.796505720633));
#32366=CARTESIAN_POINT('Ctrl Pts',(75.7405496446513,79.7157440358032,210.809239465238));
#32367=CARTESIAN_POINT('Ctrl Pts',(75.958191918574,79.3574194143084,210.838759914931));
#32368=CARTESIAN_POINT('Ctrl Pts',(76.1028124562074,79.2001630186463,210.854305339291));
#32369=CARTESIAN_POINT('Ctrl Pts',(76.4383986735495,78.9557132669801,210.884312911503));
#32370=CARTESIAN_POINT('Ctrl Pts',(76.6244149216965,78.8683037668432,210.898524896631));
#32371=CARTESIAN_POINT('Ctrl Pts',(76.8271568598205,78.8167946101776,210.911811473997));
#32372=CARTESIAN_POINT('Ctrl Pts',(76.8324403040916,78.8154809666531,210.912156277363));
#32373=CARTESIAN_POINT('Ctrl Pts',(76.8377292359511,78.8141945740678,210.912499998088));
#32374=CARTESIAN_POINT('Ctrl Pts',(76.6545412773313,78.870564692161,211.6));
#32375=CARTESIAN_POINT('Ctrl Pts',(76.7444440687127,78.8368837201247,211.60643751776));
#32376=CARTESIAN_POINT('Ctrl Pts',(76.8377292359511,78.8141945740679,211.612499998088));
#32377=CARTESIAN_POINT('Ctrl Pts',(77.7353213865851,78.5958790582345,211.670833331422));
#32378=CARTESIAN_POINT('Ctrl Pts',(78.3731842446541,79.2640589050045,211.729166664755));
#32379=CARTESIAN_POINT('Ctrl Pts',(79.011047102723,79.9322387517744,211.787499998088));
#32380=CARTESIAN_POINT('Ctrl Pts',(78.7513178101579,80.8187341143776,211.845833331422));
#32381=CARTESIAN_POINT('Ctrl Pts',(78.4915885175929,81.7052294769808,211.904166664755));
#32382=CARTESIAN_POINT('Ctrl Pts',(77.5939963669588,81.9235449928141,211.962499998088));
#32383=CARTESIAN_POINT('',(76.882500972401,78.9982710885302,212.203124998566));
#32384=CARTESIAN_POINT('Ctrl Pts',(77.5044528940591,81.5553919638894,198.443749999044));
#32385=CARTESIAN_POINT('Ctrl Pts',(76.8194139937778,81.7220095315399,198.502083332377));
#32386=CARTESIAN_POINT('Ctrl Pts',(76.332599497335,81.2120572251409,198.560416665711));
#32387=CARTESIAN_POINT('Ctrl Pts',(75.8457850008923,80.702104918742,198.618749999044));
#32388=CARTESIAN_POINT('Ctrl Pts',(76.0440094047309,80.0255350446925,198.677083332377));
#32389=CARTESIAN_POINT('Ctrl Pts',(76.2422338085695,79.3489651706431,198.735416665711));
#32390=CARTESIAN_POINT('Ctrl Pts',(76.9272727088509,79.1823476029926,198.793749999044));
#32391=CARTESIAN_POINT('Ctrl Pts',(77.6123116091322,79.0157300353421,198.852083332378));
#32392=CARTESIAN_POINT('Ctrl Pts',(78.099126105575,79.5256823417411,198.910416665711));
#32393=CARTESIAN_POINT('Ctrl Pts',(78.5859406020177,80.0356346481401,198.968749999044));
#32394=CARTESIAN_POINT('Ctrl Pts',(78.3877161981791,80.7122045221895,199.027083332377));
#32395=CARTESIAN_POINT('Ctrl Pts',(78.1894917943405,81.388774396239,199.085416665711));
#32396=CARTESIAN_POINT('Ctrl Pts',(77.5044528940591,81.5553919638894,199.143749999044));
#32397=CARTESIAN_POINT('Origin',(77.2158628014549,80.3688697834408,198.006249999044));
#32398=CARTESIAN_POINT('Ctrl Pts',(77.5044528940591,81.5553919638894,198.268749999044));
#32399=CARTESIAN_POINT('Ctrl Pts',(76.8194139937778,81.7220095315399,198.327083332377));
#32400=CARTESIAN_POINT('Ctrl Pts',(76.332599497335,81.2120572251409,198.385416665711));
#32401=CARTESIAN_POINT('Ctrl Pts',(75.8457850008923,80.702104918742,198.443749999044));
#32402=CARTESIAN_POINT('Ctrl Pts',(76.0440094047309,80.0255350446925,198.502083332377));
#32403=CARTESIAN_POINT('Ctrl Pts',(76.2422338085695,79.3489651706431,198.560416665711));
#32404=CARTESIAN_POINT('Ctrl Pts',(76.9272727088509,79.1823476029926,198.618749999044));
#32405=CARTESIAN_POINT('Ctrl Pts',(77.6123116091322,79.0157300353421,198.677083332377));
#32406=CARTESIAN_POINT('Ctrl Pts',(78.099126105575,79.5256823417411,198.735416665711));
#32407=CARTESIAN_POINT('Ctrl Pts',(78.5859406020177,80.0356346481401,198.793749999044));
#32408=CARTESIAN_POINT('Ctrl Pts',(78.3877161981791,80.7122045221895,198.852083332377));
#32409=CARTESIAN_POINT('Ctrl Pts',(78.1894917943405,81.388774396239,198.910416665711));
#32410=CARTESIAN_POINT('Ctrl Pts',(77.5044528940591,81.5553919638894,198.968749999044));
#32411=CARTESIAN_POINT('Ctrl Pts',(76.9272727088509,79.1823476029926,197.918749999044));
#32412=CARTESIAN_POINT('Ctrl Pts',(77.6123116091322,79.0157300353421,197.977083332377));
#32413=CARTESIAN_POINT('Ctrl Pts',(78.099126105575,79.5256823417411,198.035416665711));
#32414=CARTESIAN_POINT('Ctrl Pts',(78.5859406020177,80.0356346481401,198.093749999044));
#32415=CARTESIAN_POINT('Ctrl Pts',(78.3877161981791,80.7122045221895,198.152083332377));
#32416=CARTESIAN_POINT('Ctrl Pts',(78.1894917943405,81.388774396239,198.210416665711));
#32417=CARTESIAN_POINT('Ctrl Pts',(77.5044528940591,81.5553919638894,198.268749999044));
#32418=CARTESIAN_POINT('Ctrl Pts',(76.8194139937778,81.7220095315399,198.327083332377));
#32419=CARTESIAN_POINT('Ctrl Pts',(76.332599497335,81.2120572251409,198.385416665711));
#32420=CARTESIAN_POINT('Ctrl Pts',(75.8457850008923,80.702104918742,198.443749999044));
#32421=CARTESIAN_POINT('Ctrl Pts',(76.0440094047309,80.0255350446925,198.502083332377));
#32422=CARTESIAN_POINT('Ctrl Pts',(76.2422338085695,79.348965170643,198.560416665711));
#32423=CARTESIAN_POINT('Ctrl Pts',(76.9272727088509,79.1823476029926,198.618749999044));
#32424=CARTESIAN_POINT('Ctrl Pts',(77.6123116091322,79.0157300353421,198.677083332377));
#32425=CARTESIAN_POINT('Ctrl Pts',(78.099126105575,79.5256823417411,198.735416665711));
#32426=CARTESIAN_POINT('Ctrl Pts',(78.5859406020177,80.0356346481401,198.793749999044));
#32427=CARTESIAN_POINT('Ctrl Pts',(78.3877161981791,80.7122045221895,198.852083332377));
#32428=CARTESIAN_POINT('Ctrl Pts',(78.1894917943405,81.388774396239,198.910416665711));
#32429=CARTESIAN_POINT('Ctrl Pts',(77.5044528940591,81.5553919638894,198.968749999044));
#32430=CARTESIAN_POINT('Ctrl Pts',(76.8194139937778,81.7220095315399,199.027083332377));
#32431=CARTESIAN_POINT('Ctrl Pts',(76.332599497335,81.2120572251409,199.085416665711));
#32432=CARTESIAN_POINT('Ctrl Pts',(75.8457850008923,80.702104918742,199.143749999044));
#32433=CARTESIAN_POINT('Ctrl Pts',(76.0440094047309,80.0255350446925,199.202083332377));
#32434=CARTESIAN_POINT('Ctrl Pts',(76.2422338085695,79.348965170643,199.260416665711));
#32435=CARTESIAN_POINT('Ctrl Pts',(76.9272727088509,79.1823476029926,199.318749999044));
#32436=CARTESIAN_POINT('Ctrl Pts',(77.6123116091322,79.0157300353421,199.377083332377));
#32437=CARTESIAN_POINT('Ctrl Pts',(78.099126105575,79.5256823417411,199.435416665711));
#32438=CARTESIAN_POINT('Ctrl Pts',(78.5859406020177,80.0356346481401,199.493749999044));
#32439=CARTESIAN_POINT('Ctrl Pts',(78.3877161981791,80.7122045221895,199.552083332377));
#32440=CARTESIAN_POINT('Ctrl Pts',(78.1894917943405,81.388774396239,199.610416665711));
#32441=CARTESIAN_POINT('Ctrl Pts',(77.5044528940591,81.5553919638894,199.668749999044));
#32442=CARTESIAN_POINT('Ctrl Pts',(76.8194139937778,81.7220095315399,199.727083332377));
#32443=CARTESIAN_POINT('Ctrl Pts',(76.332599497335,81.2120572251409,199.785416665711));
#32444=CARTESIAN_POINT('Ctrl Pts',(75.8457850008923,80.702104918742,199.843749999044));
#32445=CARTESIAN_POINT('Ctrl Pts',(76.0440094047309,80.0255350446925,199.902083332377));
#32446=CARTESIAN_POINT('Ctrl Pts',(76.2422338085695,79.348965170643,199.960416665711));
#32447=CARTESIAN_POINT('Ctrl Pts',(76.9272727088508,79.1823476029926,200.018749999044));
#32448=CARTESIAN_POINT('Ctrl Pts',(77.6123116091322,79.0157300353421,200.077083332377));
#32449=CARTESIAN_POINT('Ctrl Pts',(78.099126105575,79.5256823417411,200.135416665711));
#32450=CARTESIAN_POINT('Ctrl Pts',(78.5859406020177,80.0356346481401,200.193749999044));
#32451=CARTESIAN_POINT('Ctrl Pts',(78.3877161981791,80.7122045221895,200.252083332377));
#32452=CARTESIAN_POINT('Ctrl Pts',(78.1894917943405,81.388774396239,200.310416665711));
#32453=CARTESIAN_POINT('Ctrl Pts',(77.5044528940591,81.5553919638894,200.368749999044));
#32454=CARTESIAN_POINT('Ctrl Pts',(76.8194139937778,81.7220095315399,200.427083332377));
#32455=CARTESIAN_POINT('Ctrl Pts',(76.332599497335,81.2120572251409,200.485416665711));
#32456=CARTESIAN_POINT('Ctrl Pts',(75.8457850008923,80.702104918742,200.543749999044));
#32457=CARTESIAN_POINT('Ctrl Pts',(76.0440094047309,80.0255350446925,200.602083332377));
#32458=CARTESIAN_POINT('Ctrl Pts',(76.2422338085695,79.348965170643,200.660416665711));
#32459=CARTESIAN_POINT('Ctrl Pts',(76.9272727088508,79.1823476029926,200.718749999044));
#32460=CARTESIAN_POINT('Ctrl Pts',(77.6123116091322,79.0157300353421,200.777083332377));
#32461=CARTESIAN_POINT('Ctrl Pts',(78.099126105575,79.5256823417411,200.835416665711));
#32462=CARTESIAN_POINT('Ctrl Pts',(78.5859406020177,80.0356346481401,200.893749999044));
#32463=CARTESIAN_POINT('Ctrl Pts',(78.3877161981791,80.7122045221895,200.952083332377));
#32464=CARTESIAN_POINT('Ctrl Pts',(78.1894917943405,81.388774396239,201.010416665711));
#32465=CARTESIAN_POINT('Ctrl Pts',(77.5044528940591,81.5553919638894,201.068749999044));
#32466=CARTESIAN_POINT('Ctrl Pts',(76.8194139937778,81.7220095315399,201.127083332377));
#32467=CARTESIAN_POINT('Ctrl Pts',(76.332599497335,81.2120572251409,201.185416665711));
#32468=CARTESIAN_POINT('Ctrl Pts',(75.8457850008923,80.702104918742,201.243749999044));
#32469=CARTESIAN_POINT('Ctrl Pts',(76.0440094047309,80.0255350446925,201.302083332377));
#32470=CARTESIAN_POINT('Ctrl Pts',(76.2422338085695,79.348965170643,201.360416665711));
#32471=CARTESIAN_POINT('Ctrl Pts',(76.9272727088508,79.1823476029926,201.418749999044));
#32472=CARTESIAN_POINT('Ctrl Pts',(77.6123116091322,79.0157300353421,201.477083332377));
#32473=CARTESIAN_POINT('Ctrl Pts',(78.099126105575,79.5256823417411,201.535416665711));
#32474=CARTESIAN_POINT('Ctrl Pts',(78.5859406020177,80.0356346481401,201.593749999044));
#32475=CARTESIAN_POINT('Ctrl Pts',(78.3877161981791,80.7122045221895,201.652083332377));
#32476=CARTESIAN_POINT('Ctrl Pts',(78.1894917943405,81.388774396239,201.710416665711));
#32477=CARTESIAN_POINT('Ctrl Pts',(77.5044528940591,81.5553919638894,201.768749999044));
#32478=CARTESIAN_POINT('Ctrl Pts',(76.8194139937778,81.7220095315399,201.827083332377));
#32479=CARTESIAN_POINT('Ctrl Pts',(76.332599497335,81.2120572251409,201.885416665711));
#32480=CARTESIAN_POINT('Ctrl Pts',(75.8457850008923,80.702104918742,201.943749999044));
#32481=CARTESIAN_POINT('Ctrl Pts',(76.0440094047309,80.0255350446925,202.002083332377));
#32482=CARTESIAN_POINT('Ctrl Pts',(76.2422338085695,79.348965170643,202.060416665711));
#32483=CARTESIAN_POINT('Ctrl Pts',(76.9272727088508,79.1823476029926,202.118749999044));
#32484=CARTESIAN_POINT('Ctrl Pts',(77.6123116091322,79.0157300353421,202.177083332377));
#32485=CARTESIAN_POINT('Ctrl Pts',(78.099126105575,79.5256823417411,202.235416665711));
#32486=CARTESIAN_POINT('Ctrl Pts',(78.5859406020177,80.0356346481401,202.293749999044));
#32487=CARTESIAN_POINT('Ctrl Pts',(78.3877161981791,80.7122045221895,202.352083332377));
#32488=CARTESIAN_POINT('Ctrl Pts',(78.1894917943405,81.388774396239,202.410416665711));
#32489=CARTESIAN_POINT('Ctrl Pts',(77.5044528940591,81.5553919638894,202.468749999044));
#32490=CARTESIAN_POINT('Ctrl Pts',(76.8194139937778,81.7220095315399,202.527083332377));
#32491=CARTESIAN_POINT('Ctrl Pts',(76.332599497335,81.2120572251409,202.585416665711));
#32492=CARTESIAN_POINT('Ctrl Pts',(75.8457850008923,80.702104918742,202.643749999044));
#32493=CARTESIAN_POINT('Ctrl Pts',(76.0440094047309,80.0255350446925,202.702083332377));
#32494=CARTESIAN_POINT('Ctrl Pts',(76.2422338085695,79.348965170643,202.760416665711));
#32495=CARTESIAN_POINT('Ctrl Pts',(76.9272727088508,79.1823476029926,202.818749999044));
#32496=CARTESIAN_POINT('Ctrl Pts',(77.6123116091322,79.0157300353421,202.877083332377));
#32497=CARTESIAN_POINT('Ctrl Pts',(78.099126105575,79.5256823417411,202.935416665711));
#32498=CARTESIAN_POINT('Ctrl Pts',(78.5859406020177,80.0356346481401,202.993749999044));
#32499=CARTESIAN_POINT('Ctrl Pts',(78.3877161981791,80.7122045221895,203.052083332377));
#32500=CARTESIAN_POINT('Ctrl Pts',(78.1894917943405,81.388774396239,203.110416665711));
#32501=CARTESIAN_POINT('Ctrl Pts',(77.5044528940591,81.5553919638894,203.168749999044));
#32502=CARTESIAN_POINT('Ctrl Pts',(76.8194139937778,81.7220095315399,203.227083332378));
#32503=CARTESIAN_POINT('Ctrl Pts',(76.332599497335,81.2120572251409,203.285416665711));
#32504=CARTESIAN_POINT('Ctrl Pts',(75.8457850008923,80.7021049187419,203.343749999044));
#32505=CARTESIAN_POINT('Ctrl Pts',(76.0440094047309,80.0255350446925,203.402083332377));
#32506=CARTESIAN_POINT('Ctrl Pts',(76.2422338085695,79.348965170643,203.460416665711));
#32507=CARTESIAN_POINT('Ctrl Pts',(76.9272727088508,79.1823476029926,203.518749999044));
#32508=CARTESIAN_POINT('Ctrl Pts',(77.6123116091322,79.0157300353421,203.577083332377));
#32509=CARTESIAN_POINT('Ctrl Pts',(78.099126105575,79.5256823417411,203.635416665711));
#32510=CARTESIAN_POINT('Ctrl Pts',(78.5859406020177,80.0356346481401,203.693749999044));
#32511=CARTESIAN_POINT('Ctrl Pts',(78.3877161981791,80.7122045221895,203.752083332377));
#32512=CARTESIAN_POINT('Ctrl Pts',(78.1894917943405,81.388774396239,203.810416665711));
#32513=CARTESIAN_POINT('Ctrl Pts',(77.5044528940591,81.5553919638894,203.868749999044));
#32514=CARTESIAN_POINT('Ctrl Pts',(76.8194139937778,81.7220095315399,203.927083332377));
#32515=CARTESIAN_POINT('Ctrl Pts',(76.332599497335,81.2120572251409,203.985416665711));
#32516=CARTESIAN_POINT('Ctrl Pts',(75.8457850008923,80.7021049187419,204.043749999044));
#32517=CARTESIAN_POINT('Ctrl Pts',(76.0440094047309,80.0255350446925,204.102083332377));
#32518=CARTESIAN_POINT('Ctrl Pts',(76.2422338085695,79.348965170643,204.160416665711));
#32519=CARTESIAN_POINT('Ctrl Pts',(76.9272727088508,79.1823476029926,204.218749999044));
#32520=CARTESIAN_POINT('Ctrl Pts',(77.6123116091322,79.0157300353421,204.277083332377));
#32521=CARTESIAN_POINT('Ctrl Pts',(78.099126105575,79.5256823417411,204.335416665711));
#32522=CARTESIAN_POINT('Ctrl Pts',(78.5859406020177,80.03563464814,204.393749999044));
#32523=CARTESIAN_POINT('Ctrl Pts',(78.3877161981791,80.7122045221895,204.452083332377));
#32524=CARTESIAN_POINT('Ctrl Pts',(78.1894917943405,81.388774396239,204.510416665711));
#32525=CARTESIAN_POINT('Ctrl Pts',(77.5044528940591,81.5553919638894,204.568749999044));
#32526=CARTESIAN_POINT('Ctrl Pts',(76.8194139937778,81.7220095315399,204.627083332377));
#32527=CARTESIAN_POINT('Ctrl Pts',(76.332599497335,81.2120572251409,204.685416665711));
#32528=CARTESIAN_POINT('Ctrl Pts',(75.8457850008923,80.7021049187419,204.743749999044));
#32529=CARTESIAN_POINT('Ctrl Pts',(76.0440094047309,80.0255350446925,204.802083332377));
#32530=CARTESIAN_POINT('Ctrl Pts',(76.2422338085695,79.348965170643,204.860416665711));
#32531=CARTESIAN_POINT('Ctrl Pts',(76.9272727088508,79.1823476029926,204.918749999044));
#32532=CARTESIAN_POINT('Ctrl Pts',(77.6123116091322,79.0157300353421,204.977083332377));
#32533=CARTESIAN_POINT('Ctrl Pts',(78.099126105575,79.5256823417411,205.035416665711));
#32534=CARTESIAN_POINT('Ctrl Pts',(78.5859406020177,80.03563464814,205.093749999044));
#32535=CARTESIAN_POINT('Ctrl Pts',(78.3877161981791,80.7122045221895,205.152083332377));
#32536=CARTESIAN_POINT('Ctrl Pts',(78.1894917943405,81.388774396239,205.210416665711));
#32537=CARTESIAN_POINT('Ctrl Pts',(77.5044528940591,81.5553919638894,205.268749999044));
#32538=CARTESIAN_POINT('Ctrl Pts',(76.8194139937778,81.7220095315399,205.327083332377));
#32539=CARTESIAN_POINT('Ctrl Pts',(76.332599497335,81.2120572251409,205.385416665711));
#32540=CARTESIAN_POINT('Ctrl Pts',(75.8457850008923,80.7021049187419,205.443749999044));
#32541=CARTESIAN_POINT('Ctrl Pts',(76.0440094047309,80.0255350446925,205.502083332377));
#32542=CARTESIAN_POINT('Ctrl Pts',(76.2422338085695,79.348965170643,205.560416665711));
#32543=CARTESIAN_POINT('Ctrl Pts',(76.9272727088508,79.1823476029926,205.618749999044));
#32544=CARTESIAN_POINT('Ctrl Pts',(77.6123116091322,79.0157300353421,205.677083332377));
#32545=CARTESIAN_POINT('Ctrl Pts',(78.099126105575,79.5256823417411,205.735416665711));
#32546=CARTESIAN_POINT('Ctrl Pts',(78.5859406020177,80.03563464814,205.793749999044));
#32547=CARTESIAN_POINT('Ctrl Pts',(78.3877161981791,80.7122045221895,205.852083332377));
#32548=CARTESIAN_POINT('Ctrl Pts',(78.1894917943405,81.388774396239,205.910416665711));
#32549=CARTESIAN_POINT('Ctrl Pts',(77.5044528940591,81.5553919638894,205.968749999044));
#32550=CARTESIAN_POINT('Ctrl Pts',(76.8194139937778,81.7220095315399,206.027083332377));
#32551=CARTESIAN_POINT('Ctrl Pts',(76.332599497335,81.2120572251409,206.085416665711));
#32552=CARTESIAN_POINT('Ctrl Pts',(75.8457850008923,80.7021049187419,206.143749999044));
#32553=CARTESIAN_POINT('Ctrl Pts',(76.0440094047309,80.0255350446925,206.202083332377));
#32554=CARTESIAN_POINT('Ctrl Pts',(76.2422338085695,79.348965170643,206.260416665711));
#32555=CARTESIAN_POINT('Ctrl Pts',(76.9272727088508,79.1823476029926,206.318749999044));
#32556=CARTESIAN_POINT('Ctrl Pts',(77.6123116091322,79.0157300353421,206.377083332377));
#32557=CARTESIAN_POINT('Ctrl Pts',(78.099126105575,79.5256823417411,206.435416665711));
#32558=CARTESIAN_POINT('Ctrl Pts',(78.5859406020177,80.03563464814,206.493749999044));
#32559=CARTESIAN_POINT('Ctrl Pts',(78.3877161981791,80.7122045221895,206.552083332377));
#32560=CARTESIAN_POINT('Ctrl Pts',(78.1894917943405,81.3887743962389,206.610416665711));
#32561=CARTESIAN_POINT('Ctrl Pts',(77.5044528940591,81.5553919638894,206.668749999044));
#32562=CARTESIAN_POINT('Ctrl Pts',(76.8194139937778,81.7220095315399,206.727083332378));
#32563=CARTESIAN_POINT('Ctrl Pts',(76.332599497335,81.2120572251409,206.785416665711));
#32564=CARTESIAN_POINT('Ctrl Pts',(75.8457850008923,80.7021049187419,206.843749999044));
#32565=CARTESIAN_POINT('Ctrl Pts',(76.0440094047309,80.0255350446925,206.902083332377));
#32566=CARTESIAN_POINT('Ctrl Pts',(76.2422338085695,79.348965170643,206.960416665711));
#32567=CARTESIAN_POINT('Ctrl Pts',(76.9272727088508,79.1823476029926,207.018749999044));
#32568=CARTESIAN_POINT('Ctrl Pts',(77.6123116091322,79.0157300353421,207.077083332377));
#32569=CARTESIAN_POINT('Ctrl Pts',(78.099126105575,79.5256823417411,207.135416665711));
#32570=CARTESIAN_POINT('Ctrl Pts',(78.5859406020177,80.03563464814,207.193749999044));
#32571=CARTESIAN_POINT('Ctrl Pts',(78.3877161981791,80.7122045221895,207.252083332377));
#32572=CARTESIAN_POINT('Ctrl Pts',(78.1894917943405,81.3887743962389,207.310416665711));
#32573=CARTESIAN_POINT('Ctrl Pts',(77.5044528940591,81.5553919638894,207.368749999044));
#32574=CARTESIAN_POINT('Ctrl Pts',(76.8194139937778,81.7220095315399,207.427083332377));
#32575=CARTESIAN_POINT('Ctrl Pts',(76.332599497335,81.2120572251409,207.485416665711));
#32576=CARTESIAN_POINT('Ctrl Pts',(75.8457850008923,80.7021049187419,207.543749999044));
#32577=CARTESIAN_POINT('Ctrl Pts',(76.0440094047309,80.0255350446925,207.602083332377));
#32578=CARTESIAN_POINT('Ctrl Pts',(76.2422338085695,79.348965170643,207.660416665711));
#32579=CARTESIAN_POINT('Ctrl Pts',(76.9272727088508,79.1823476029926,207.718749999044));
#32580=CARTESIAN_POINT('Ctrl Pts',(77.6123116091322,79.0157300353421,207.777083332377));
#32581=CARTESIAN_POINT('Ctrl Pts',(78.0991261055749,79.5256823417411,207.835416665711));
#32582=CARTESIAN_POINT('Ctrl Pts',(78.5859406020177,80.03563464814,207.893749999044));
#32583=CARTESIAN_POINT('Ctrl Pts',(78.3877161981791,80.7122045221895,207.952083332377));
#32584=CARTESIAN_POINT('Ctrl Pts',(78.1894917943405,81.3887743962389,208.010416665711));
#32585=CARTESIAN_POINT('Ctrl Pts',(77.5044528940591,81.5553919638894,208.068749999044));
#32586=CARTESIAN_POINT('Ctrl Pts',(76.8194139937778,81.7220095315399,208.127083332377));
#32587=CARTESIAN_POINT('Ctrl Pts',(76.332599497335,81.2120572251409,208.185416665711));
#32588=CARTESIAN_POINT('Ctrl Pts',(75.8457850008923,80.7021049187419,208.243749999044));
#32589=CARTESIAN_POINT('Ctrl Pts',(76.0440094047309,80.0255350446925,208.302083332377));
#32590=CARTESIAN_POINT('Ctrl Pts',(76.2422338085695,79.348965170643,208.360416665711));
#32591=CARTESIAN_POINT('Ctrl Pts',(76.9272727088508,79.1823476029926,208.418749999044));
#32592=CARTESIAN_POINT('Ctrl Pts',(77.6123116091322,79.0157300353421,208.477083332377));
#32593=CARTESIAN_POINT('Ctrl Pts',(78.0991261055749,79.5256823417411,208.535416665711));
#32594=CARTESIAN_POINT('Ctrl Pts',(78.5859406020177,80.03563464814,208.593749999044));
#32595=CARTESIAN_POINT('Ctrl Pts',(78.3877161981791,80.7122045221895,208.652083332377));
#32596=CARTESIAN_POINT('Ctrl Pts',(78.1894917943405,81.3887743962389,208.710416665711));
#32597=CARTESIAN_POINT('Ctrl Pts',(77.5044528940591,81.5553919638894,208.768749999044));
#32598=CARTESIAN_POINT('Ctrl Pts',(76.8194139937778,81.7220095315399,208.827083332377));
#32599=CARTESIAN_POINT('Ctrl Pts',(76.332599497335,81.2120572251409,208.885416665711));
#32600=CARTESIAN_POINT('Ctrl Pts',(75.8457850008923,80.7021049187419,208.943749999044));
#32601=CARTESIAN_POINT('Ctrl Pts',(76.0440094047309,80.0255350446925,209.002083332377));
#32602=CARTESIAN_POINT('Ctrl Pts',(76.2422338085695,79.348965170643,209.060416665711));
#32603=CARTESIAN_POINT('Ctrl Pts',(76.9272727088508,79.1823476029926,209.118749999044));
#32604=CARTESIAN_POINT('Ctrl Pts',(77.6123116091322,79.0157300353421,209.177083332377));
#32605=CARTESIAN_POINT('Ctrl Pts',(78.0991261055749,79.5256823417411,209.235416665711));
#32606=CARTESIAN_POINT('Ctrl Pts',(78.5859406020177,80.03563464814,209.293749999044));
#32607=CARTESIAN_POINT('Ctrl Pts',(78.3877161981791,80.7122045221895,209.352083332377));
#32608=CARTESIAN_POINT('Ctrl Pts',(78.1894917943405,81.3887743962389,209.410416665711));
#32609=CARTESIAN_POINT('Ctrl Pts',(77.5044528940591,81.5553919638894,209.468749999044));
#32610=CARTESIAN_POINT('Ctrl Pts',(76.8194139937778,81.7220095315399,209.527083332378));
#32611=CARTESIAN_POINT('Ctrl Pts',(76.332599497335,81.2120572251409,209.585416665711));
#32612=CARTESIAN_POINT('Ctrl Pts',(75.8457850008923,80.7021049187419,209.643749999044));
#32613=CARTESIAN_POINT('Ctrl Pts',(76.0440094047309,80.0255350446925,209.702083332377));
#32614=CARTESIAN_POINT('Ctrl Pts',(76.2422338085695,79.348965170643,209.760416665711));
#32615=CARTESIAN_POINT('Ctrl Pts',(76.9272727088508,79.1823476029926,209.818749999044));
#32616=CARTESIAN_POINT('Ctrl Pts',(77.6123116091322,79.0157300353421,209.877083332377));
#32617=CARTESIAN_POINT('Ctrl Pts',(78.0991261055749,79.5256823417411,209.935416665711));
#32618=CARTESIAN_POINT('Ctrl Pts',(78.5859406020177,80.03563464814,209.993749999044));
#32619=CARTESIAN_POINT('Ctrl Pts',(78.3877161981791,80.7122045221895,210.052083332377));
#32620=CARTESIAN_POINT('Ctrl Pts',(78.1894917943405,81.3887743962389,210.110416665711));
#32621=CARTESIAN_POINT('Ctrl Pts',(77.5044528940591,81.5553919638894,210.168749999044));
#32622=CARTESIAN_POINT('Ctrl Pts',(76.8194139937778,81.7220095315399,210.227083332377));
#32623=CARTESIAN_POINT('Ctrl Pts',(76.332599497335,81.2120572251409,210.285416665711));
#32624=CARTESIAN_POINT('Ctrl Pts',(75.8457850008923,80.7021049187419,210.343749999044));
#32625=CARTESIAN_POINT('Ctrl Pts',(76.0440094047309,80.0255350446925,210.402083332377));
#32626=CARTESIAN_POINT('Ctrl Pts',(76.2422338085695,79.348965170643,210.460416665711));
#32627=CARTESIAN_POINT('Ctrl Pts',(76.9272727088508,79.1823476029926,210.518749999044));
#32628=CARTESIAN_POINT('Ctrl Pts',(77.6123116091322,79.0157300353421,210.577083332377));
#32629=CARTESIAN_POINT('Ctrl Pts',(78.0991261055749,79.5256823417411,210.635416665711));
#32630=CARTESIAN_POINT('Ctrl Pts',(78.5859406020177,80.03563464814,210.693749999044));
#32631=CARTESIAN_POINT('Ctrl Pts',(78.3877161981791,80.7122045221895,210.752083332377));
#32632=CARTESIAN_POINT('Ctrl Pts',(78.1894917943405,81.3887743962389,210.810416665711));
#32633=CARTESIAN_POINT('Ctrl Pts',(77.5044528940591,81.5553919638894,210.868749999044));
#32634=CARTESIAN_POINT('Ctrl Pts',(76.8194139937778,81.7220095315399,210.927083332377));
#32635=CARTESIAN_POINT('Ctrl Pts',(76.332599497335,81.2120572251409,210.985416665711));
#32636=CARTESIAN_POINT('Ctrl Pts',(75.8457850008923,80.7021049187419,211.043749999044));
#32637=CARTESIAN_POINT('Ctrl Pts',(76.0440094047309,80.0255350446925,211.102083332377));
#32638=CARTESIAN_POINT('Ctrl Pts',(76.2422338085695,79.348965170643,211.160416665711));
#32639=CARTESIAN_POINT('Ctrl Pts',(76.9272727088508,79.1823476029925,211.218749999044));
#32640=CARTESIAN_POINT('Ctrl Pts',(77.6123116091322,79.0157300353421,211.277083332377));
#32641=CARTESIAN_POINT('Ctrl Pts',(78.0991261055749,79.5256823417411,211.335416665711));
#32642=CARTESIAN_POINT('Ctrl Pts',(78.5859406020177,80.03563464814,211.393749999044));
#32643=CARTESIAN_POINT('Ctrl Pts',(78.3877161981791,80.7122045221895,211.452083332377));
#32644=CARTESIAN_POINT('Ctrl Pts',(78.1894917943405,81.3887743962389,211.510416665711));
#32645=CARTESIAN_POINT('Ctrl Pts',(77.5044528940591,81.5553919638894,211.568749999044));
#32646=CARTESIAN_POINT('Ctrl Pts',(76.8194139937778,81.7220095315399,211.627083332377));
#32647=CARTESIAN_POINT('Ctrl Pts',(76.332599497335,81.2120572251409,211.685416665711));
#32648=CARTESIAN_POINT('Ctrl Pts',(75.8457850008923,80.7021049187419,211.743749999044));
#32649=CARTESIAN_POINT('Ctrl Pts',(76.0440094047309,80.0255350446925,211.802083332377));
#32650=CARTESIAN_POINT('Ctrl Pts',(76.2422338085695,79.348965170643,211.860416665711));
#32651=CARTESIAN_POINT('Ctrl Pts',(76.9272727088508,79.1823476029925,211.918749999044));
#32652=CARTESIAN_POINT('Ctrl Pts',(76.8377292359511,78.8141945740679,197.7));
#32653=CARTESIAN_POINT('Ctrl Pts',(77.7353213865851,78.5958790582346,197.758333333333));
#32654=CARTESIAN_POINT('Ctrl Pts',(78.3731842446541,79.2640589050045,197.816666666667));
#32655=CARTESIAN_POINT('Ctrl Pts',(79.011047102723,79.9322387517744,197.875));
#32656=CARTESIAN_POINT('Ctrl Pts',(78.7513178101579,80.8187341143776,197.933333333333));
#32657=CARTESIAN_POINT('Ctrl Pts',(78.4915885175929,81.7052294769809,197.991666666667));
#32658=CARTESIAN_POINT('Ctrl Pts',(77.5939963669589,81.9235449928141,198.05));
#32659=CARTESIAN_POINT('Ctrl Pts',(76.6964042163248,82.1418605086474,198.108333333333));
#32660=CARTESIAN_POINT('Ctrl Pts',(76.0585413582559,81.4736806618775,198.166666666667));
#32661=CARTESIAN_POINT('Ctrl Pts',(75.420678500187,80.8055008151076,198.225));
#32662=CARTESIAN_POINT('Ctrl Pts',(75.6804077927521,79.9190054525044,198.283333333333));
#32663=CARTESIAN_POINT('Ctrl Pts',(75.9401370853171,79.0325100899012,198.341666666667));
#32664=CARTESIAN_POINT('Ctrl Pts',(76.8377292359511,78.8141945740679,198.4));
#32665=CARTESIAN_POINT('Ctrl Pts',(77.7353213865851,78.5958790582346,198.458333333333));
#32666=CARTESIAN_POINT('Ctrl Pts',(78.3731842446541,79.2640589050045,198.516666666667));
#32667=CARTESIAN_POINT('Ctrl Pts',(79.011047102723,79.9322387517744,198.575));
#32668=CARTESIAN_POINT('Ctrl Pts',(78.7513178101579,80.8187341143776,198.633333333333));
#32669=CARTESIAN_POINT('Ctrl Pts',(78.4915885175929,81.7052294769809,198.691666666667));
#32670=CARTESIAN_POINT('Ctrl Pts',(77.5939963669589,81.9235449928141,198.75));
#32671=CARTESIAN_POINT('Ctrl Pts',(76.6964042163248,82.1418605086474,198.808333333333));
#32672=CARTESIAN_POINT('Ctrl Pts',(76.0585413582559,81.4736806618775,198.866666666667));
#32673=CARTESIAN_POINT('Ctrl Pts',(75.420678500187,80.8055008151076,198.925));
#32674=CARTESIAN_POINT('Ctrl Pts',(75.6804077927521,79.9190054525044,198.983333333333));
#32675=CARTESIAN_POINT('Ctrl Pts',(75.9401370853171,79.0325100899012,199.041666666667));
#32676=CARTESIAN_POINT('Ctrl Pts',(76.8377292359511,78.8141945740679,199.1));
#32677=CARTESIAN_POINT('Ctrl Pts',(77.7353213865851,78.5958790582346,199.158333333333));
#32678=CARTESIAN_POINT('Ctrl Pts',(78.3731842446541,79.2640589050045,199.216666666667));
#32679=CARTESIAN_POINT('Ctrl Pts',(79.011047102723,79.9322387517744,199.275));
#32680=CARTESIAN_POINT('Ctrl Pts',(78.7513178101579,80.8187341143776,199.333333333333));
#32681=CARTESIAN_POINT('Ctrl Pts',(78.4915885175929,81.7052294769809,199.391666666667));
#32682=CARTESIAN_POINT('Ctrl Pts',(77.5939963669589,81.9235449928141,199.45));
#32683=CARTESIAN_POINT('Ctrl Pts',(76.6964042163248,82.1418605086474,199.508333333333));
#32684=CARTESIAN_POINT('Ctrl Pts',(76.0585413582559,81.4736806618775,199.566666666667));
#32685=CARTESIAN_POINT('Ctrl Pts',(75.420678500187,80.8055008151076,199.625));
#32686=CARTESIAN_POINT('Ctrl Pts',(75.6804077927521,79.9190054525044,199.683333333333));
#32687=CARTESIAN_POINT('Ctrl Pts',(75.9401370853171,79.0325100899012,199.741666666667));
#32688=CARTESIAN_POINT('Ctrl Pts',(76.8377292359511,78.8141945740679,199.8));
#32689=CARTESIAN_POINT('Ctrl Pts',(77.7353213865851,78.5958790582346,199.858333333333));
#32690=CARTESIAN_POINT('Ctrl Pts',(78.3731842446541,79.2640589050045,199.916666666667));
#32691=CARTESIAN_POINT('Ctrl Pts',(79.011047102723,79.9322387517744,199.975));
#32692=CARTESIAN_POINT('Ctrl Pts',(78.7513178101579,80.8187341143776,200.033333333333));
#32693=CARTESIAN_POINT('Ctrl Pts',(78.4915885175929,81.7052294769809,200.091666666667));
#32694=CARTESIAN_POINT('Ctrl Pts',(77.5939963669589,81.9235449928141,200.15));
#32695=CARTESIAN_POINT('Ctrl Pts',(76.6964042163248,82.1418605086474,200.208333333333));
#32696=CARTESIAN_POINT('Ctrl Pts',(76.0585413582559,81.4736806618775,200.266666666667));
#32697=CARTESIAN_POINT('Ctrl Pts',(75.420678500187,80.8055008151076,200.325));
#32698=CARTESIAN_POINT('Ctrl Pts',(75.680407792752,79.9190054525044,200.383333333333));
#32699=CARTESIAN_POINT('Ctrl Pts',(75.9401370853171,79.0325100899012,200.441666666667));
#32700=CARTESIAN_POINT('Ctrl Pts',(76.8377292359511,78.8141945740679,200.5));
#32701=CARTESIAN_POINT('Ctrl Pts',(77.7353213865851,78.5958790582346,200.558333333333));
#32702=CARTESIAN_POINT('Ctrl Pts',(78.3731842446541,79.2640589050045,200.616666666667));
#32703=CARTESIAN_POINT('Ctrl Pts',(79.011047102723,79.9322387517744,200.675));
#32704=CARTESIAN_POINT('Ctrl Pts',(78.7513178101579,80.8187341143776,200.733333333333));
#32705=CARTESIAN_POINT('Ctrl Pts',(78.4915885175929,81.7052294769809,200.791666666667));
#32706=CARTESIAN_POINT('Ctrl Pts',(77.5939963669589,81.9235449928141,200.85));
#32707=CARTESIAN_POINT('Ctrl Pts',(76.6964042163248,82.1418605086474,200.908333333333));
#32708=CARTESIAN_POINT('Ctrl Pts',(76.0585413582559,81.4736806618775,200.966666666667));
#32709=CARTESIAN_POINT('Ctrl Pts',(75.420678500187,80.8055008151076,201.025));
#32710=CARTESIAN_POINT('Ctrl Pts',(75.680407792752,79.9190054525044,201.083333333333));
#32711=CARTESIAN_POINT('Ctrl Pts',(75.9401370853171,79.0325100899012,201.141666666667));
#32712=CARTESIAN_POINT('Ctrl Pts',(76.8377292359511,78.8141945740679,201.2));
#32713=CARTESIAN_POINT('Ctrl Pts',(77.7353213865851,78.5958790582346,201.258333333333));
#32714=CARTESIAN_POINT('Ctrl Pts',(78.3731842446541,79.2640589050045,201.316666666667));
#32715=CARTESIAN_POINT('Ctrl Pts',(79.011047102723,79.9322387517744,201.375));
#32716=CARTESIAN_POINT('Ctrl Pts',(78.7513178101579,80.8187341143776,201.433333333333));
#32717=CARTESIAN_POINT('Ctrl Pts',(78.4915885175929,81.7052294769809,201.491666666667));
#32718=CARTESIAN_POINT('Ctrl Pts',(77.5939963669589,81.9235449928141,201.55));
#32719=CARTESIAN_POINT('Ctrl Pts',(76.6964042163248,82.1418605086474,201.608333333333));
#32720=CARTESIAN_POINT('Ctrl Pts',(76.0585413582559,81.4736806618775,201.666666666667));
#32721=CARTESIAN_POINT('Ctrl Pts',(75.420678500187,80.8055008151076,201.725));
#32722=CARTESIAN_POINT('Ctrl Pts',(75.680407792752,79.9190054525044,201.783333333333));
#32723=CARTESIAN_POINT('Ctrl Pts',(75.9401370853171,79.0325100899012,201.841666666667));
#32724=CARTESIAN_POINT('Ctrl Pts',(76.8377292359511,78.8141945740679,201.9));
#32725=CARTESIAN_POINT('Ctrl Pts',(77.7353213865851,78.5958790582346,201.958333333333));
#32726=CARTESIAN_POINT('Ctrl Pts',(78.3731842446541,79.2640589050045,202.016666666667));
#32727=CARTESIAN_POINT('Ctrl Pts',(79.011047102723,79.9322387517744,202.075));
#32728=CARTESIAN_POINT('Ctrl Pts',(78.7513178101579,80.8187341143776,202.133333333333));
#32729=CARTESIAN_POINT('Ctrl Pts',(78.4915885175929,81.7052294769808,202.191666666667));
#32730=CARTESIAN_POINT('Ctrl Pts',(77.5939963669589,81.9235449928141,202.25));
#32731=CARTESIAN_POINT('Ctrl Pts',(76.6964042163248,82.1418605086474,202.308333333333));
#32732=CARTESIAN_POINT('Ctrl Pts',(76.0585413582559,81.4736806618775,202.366666666667));
#32733=CARTESIAN_POINT('Ctrl Pts',(75.420678500187,80.8055008151076,202.425));
#32734=CARTESIAN_POINT('Ctrl Pts',(75.680407792752,79.9190054525044,202.483333333333));
#32735=CARTESIAN_POINT('Ctrl Pts',(75.9401370853171,79.0325100899012,202.541666666667));
#32736=CARTESIAN_POINT('Ctrl Pts',(76.8377292359511,78.8141945740679,202.6));
#32737=CARTESIAN_POINT('Ctrl Pts',(77.7353213865851,78.5958790582346,202.658333333333));
#32738=CARTESIAN_POINT('Ctrl Pts',(78.3731842446541,79.2640589050045,202.716666666667));
#32739=CARTESIAN_POINT('Ctrl Pts',(79.011047102723,79.9322387517744,202.775));
#32740=CARTESIAN_POINT('Ctrl Pts',(78.7513178101579,80.8187341143776,202.833333333333));
#32741=CARTESIAN_POINT('Ctrl Pts',(78.4915885175929,81.7052294769808,202.891666666667));
#32742=CARTESIAN_POINT('Ctrl Pts',(77.5939963669589,81.9235449928141,202.95));
#32743=CARTESIAN_POINT('Ctrl Pts',(76.6964042163248,82.1418605086474,203.008333333333));
#32744=CARTESIAN_POINT('Ctrl Pts',(76.0585413582559,81.4736806618775,203.066666666667));
#32745=CARTESIAN_POINT('Ctrl Pts',(75.420678500187,80.8055008151076,203.125));
#32746=CARTESIAN_POINT('Ctrl Pts',(75.680407792752,79.9190054525044,203.183333333333));
#32747=CARTESIAN_POINT('Ctrl Pts',(75.9401370853171,79.0325100899012,203.241666666667));
#32748=CARTESIAN_POINT('Ctrl Pts',(76.8377292359511,78.8141945740679,203.3));
#32749=CARTESIAN_POINT('Ctrl Pts',(77.7353213865851,78.5958790582346,203.358333333333));
#32750=CARTESIAN_POINT('Ctrl Pts',(78.3731842446541,79.2640589050045,203.416666666667));
#32751=CARTESIAN_POINT('Ctrl Pts',(79.011047102723,79.9322387517744,203.475));
#32752=CARTESIAN_POINT('Ctrl Pts',(78.7513178101579,80.8187341143776,203.533333333333));
#32753=CARTESIAN_POINT('Ctrl Pts',(78.4915885175929,81.7052294769808,203.591666666667));
#32754=CARTESIAN_POINT('Ctrl Pts',(77.5939963669589,81.9235449928141,203.65));
#32755=CARTESIAN_POINT('Ctrl Pts',(76.6964042163248,82.1418605086474,203.708333333333));
#32756=CARTESIAN_POINT('Ctrl Pts',(76.0585413582559,81.4736806618775,203.766666666667));
#32757=CARTESIAN_POINT('Ctrl Pts',(75.420678500187,80.8055008151076,203.825));
#32758=CARTESIAN_POINT('Ctrl Pts',(75.680407792752,79.9190054525044,203.883333333333));
#32759=CARTESIAN_POINT('Ctrl Pts',(75.9401370853171,79.0325100899012,203.941666666667));
#32760=CARTESIAN_POINT('Ctrl Pts',(76.8377292359511,78.8141945740679,204.));
#32761=CARTESIAN_POINT('Ctrl Pts',(77.7353213865851,78.5958790582346,204.058333333333));
#32762=CARTESIAN_POINT('Ctrl Pts',(78.3731842446541,79.2640589050045,204.116666666667));
#32763=CARTESIAN_POINT('Ctrl Pts',(79.011047102723,79.9322387517744,204.175));
#32764=CARTESIAN_POINT('Ctrl Pts',(78.7513178101579,80.8187341143776,204.233333333333));
#32765=CARTESIAN_POINT('Ctrl Pts',(78.4915885175929,81.7052294769808,204.291666666667));
#32766=CARTESIAN_POINT('Ctrl Pts',(77.5939963669589,81.9235449928141,204.35));
#32767=CARTESIAN_POINT('Ctrl Pts',(76.6964042163248,82.1418605086474,204.408333333333));
#32768=CARTESIAN_POINT('Ctrl Pts',(76.0585413582559,81.4736806618775,204.466666666667));
#32769=CARTESIAN_POINT('Ctrl Pts',(75.420678500187,80.8055008151076,204.525));
#32770=CARTESIAN_POINT('Ctrl Pts',(75.680407792752,79.9190054525044,204.583333333333));
#32771=CARTESIAN_POINT('Ctrl Pts',(75.9401370853171,79.0325100899012,204.641666666667));
#32772=CARTESIAN_POINT('Ctrl Pts',(76.8377292359511,78.8141945740679,204.7));
#32773=CARTESIAN_POINT('Ctrl Pts',(77.7353213865851,78.5958790582346,204.758333333333));
#32774=CARTESIAN_POINT('Ctrl Pts',(78.3731842446541,79.2640589050045,204.816666666667));
#32775=CARTESIAN_POINT('Ctrl Pts',(79.011047102723,79.9322387517744,204.875));
#32776=CARTESIAN_POINT('Ctrl Pts',(78.7513178101579,80.8187341143776,204.933333333333));
#32777=CARTESIAN_POINT('Ctrl Pts',(78.4915885175928,81.7052294769808,204.991666666667));
#32778=CARTESIAN_POINT('Ctrl Pts',(77.5939963669589,81.9235449928141,205.05));
#32779=CARTESIAN_POINT('Ctrl Pts',(76.6964042163248,82.1418605086474,205.108333333333));
#32780=CARTESIAN_POINT('Ctrl Pts',(76.0585413582559,81.4736806618775,205.166666666667));
#32781=CARTESIAN_POINT('Ctrl Pts',(75.420678500187,80.8055008151076,205.225));
#32782=CARTESIAN_POINT('Ctrl Pts',(75.680407792752,79.9190054525044,205.283333333333));
#32783=CARTESIAN_POINT('Ctrl Pts',(75.9401370853171,79.0325100899011,205.341666666667));
#32784=CARTESIAN_POINT('Ctrl Pts',(76.8377292359511,78.8141945740679,205.4));
#32785=CARTESIAN_POINT('Ctrl Pts',(77.7353213865851,78.5958790582346,205.458333333333));
#32786=CARTESIAN_POINT('Ctrl Pts',(78.3731842446541,79.2640589050045,205.516666666667));
#32787=CARTESIAN_POINT('Ctrl Pts',(79.011047102723,79.9322387517744,205.575));
#32788=CARTESIAN_POINT('Ctrl Pts',(78.7513178101579,80.8187341143776,205.633333333333));
#32789=CARTESIAN_POINT('Ctrl Pts',(78.4915885175928,81.7052294769808,205.691666666667));
#32790=CARTESIAN_POINT('Ctrl Pts',(77.5939963669589,81.9235449928141,205.75));
#32791=CARTESIAN_POINT('Ctrl Pts',(76.6964042163248,82.1418605086474,205.808333333333));
#32792=CARTESIAN_POINT('Ctrl Pts',(76.0585413582559,81.4736806618775,205.866666666667));
#32793=CARTESIAN_POINT('Ctrl Pts',(75.420678500187,80.8055008151076,205.925));
#32794=CARTESIAN_POINT('Ctrl Pts',(75.680407792752,79.9190054525044,205.983333333333));
#32795=CARTESIAN_POINT('Ctrl Pts',(75.9401370853171,79.0325100899011,206.041666666667));
#32796=CARTESIAN_POINT('Ctrl Pts',(76.8377292359511,78.8141945740679,206.1));
#32797=CARTESIAN_POINT('Ctrl Pts',(77.7353213865851,78.5958790582346,206.158333333333));
#32798=CARTESIAN_POINT('Ctrl Pts',(78.3731842446541,79.2640589050045,206.216666666667));
#32799=CARTESIAN_POINT('Ctrl Pts',(79.011047102723,79.9322387517744,206.275));
#32800=CARTESIAN_POINT('Ctrl Pts',(78.7513178101579,80.8187341143776,206.333333333333));
#32801=CARTESIAN_POINT('Ctrl Pts',(78.4915885175928,81.7052294769808,206.391666666667));
#32802=CARTESIAN_POINT('Ctrl Pts',(77.5939963669589,81.9235449928141,206.45));
#32803=CARTESIAN_POINT('Ctrl Pts',(76.6964042163248,82.1418605086474,206.508333333333));
#32804=CARTESIAN_POINT('Ctrl Pts',(76.0585413582559,81.4736806618775,206.566666666667));
#32805=CARTESIAN_POINT('Ctrl Pts',(75.420678500187,80.8055008151076,206.625));
#32806=CARTESIAN_POINT('Ctrl Pts',(75.680407792752,79.9190054525043,206.683333333333));
#32807=CARTESIAN_POINT('Ctrl Pts',(75.9401370853171,79.0325100899011,206.741666666667));
#32808=CARTESIAN_POINT('Ctrl Pts',(76.8377292359511,78.8141945740679,206.8));
#32809=CARTESIAN_POINT('Ctrl Pts',(77.7353213865851,78.5958790582346,206.858333333333));
#32810=CARTESIAN_POINT('Ctrl Pts',(78.3731842446541,79.2640589050045,206.916666666667));
#32811=CARTESIAN_POINT('Ctrl Pts',(79.011047102723,79.9322387517744,206.975));
#32812=CARTESIAN_POINT('Ctrl Pts',(78.7513178101579,80.8187341143776,207.033333333333));
#32813=CARTESIAN_POINT('Ctrl Pts',(78.4915885175928,81.7052294769808,207.091666666667));
#32814=CARTESIAN_POINT('Ctrl Pts',(77.5939963669589,81.9235449928141,207.15));
#32815=CARTESIAN_POINT('Ctrl Pts',(76.6964042163248,82.1418605086474,207.208333333333));
#32816=CARTESIAN_POINT('Ctrl Pts',(76.0585413582559,81.4736806618775,207.266666666667));
#32817=CARTESIAN_POINT('Ctrl Pts',(75.420678500187,80.8055008151075,207.325));
#32818=CARTESIAN_POINT('Ctrl Pts',(75.680407792752,79.9190054525043,207.383333333333));
#32819=CARTESIAN_POINT('Ctrl Pts',(75.9401370853171,79.0325100899011,207.441666666667));
#32820=CARTESIAN_POINT('Ctrl Pts',(76.8377292359511,78.8141945740679,207.5));
#32821=CARTESIAN_POINT('Ctrl Pts',(77.7353213865851,78.5958790582346,207.558333333333));
#32822=CARTESIAN_POINT('Ctrl Pts',(78.3731842446541,79.2640589050045,207.616666666667));
#32823=CARTESIAN_POINT('Ctrl Pts',(79.011047102723,79.9322387517744,207.675));
#32824=CARTESIAN_POINT('Ctrl Pts',(78.7513178101579,80.8187341143776,207.733333333333));
#32825=CARTESIAN_POINT('Ctrl Pts',(78.4915885175928,81.7052294769808,207.791666666667));
#32826=CARTESIAN_POINT('Ctrl Pts',(77.5939963669589,81.9235449928141,207.85));
#32827=CARTESIAN_POINT('Ctrl Pts',(76.6964042163248,82.1418605086474,207.908333333333));
#32828=CARTESIAN_POINT('Ctrl Pts',(76.0585413582559,81.4736806618775,207.966666666667));
#32829=CARTESIAN_POINT('Ctrl Pts',(75.420678500187,80.8055008151075,208.025));
#32830=CARTESIAN_POINT('Ctrl Pts',(75.680407792752,79.9190054525043,208.083333333333));
#32831=CARTESIAN_POINT('Ctrl Pts',(75.9401370853171,79.0325100899011,208.141666666667));
#32832=CARTESIAN_POINT('Ctrl Pts',(76.8377292359511,78.8141945740679,208.2));
#32833=CARTESIAN_POINT('Ctrl Pts',(77.7353213865851,78.5958790582346,208.258333333333));
#32834=CARTESIAN_POINT('Ctrl Pts',(78.3731842446541,79.2640589050045,208.316666666667));
#32835=CARTESIAN_POINT('Ctrl Pts',(79.011047102723,79.9322387517744,208.375));
#32836=CARTESIAN_POINT('Ctrl Pts',(78.7513178101579,80.8187341143776,208.433333333333));
#32837=CARTESIAN_POINT('Ctrl Pts',(78.4915885175928,81.7052294769808,208.491666666667));
#32838=CARTESIAN_POINT('Ctrl Pts',(77.5939963669589,81.9235449928141,208.55));
#32839=CARTESIAN_POINT('Ctrl Pts',(76.6964042163248,82.1418605086474,208.608333333333));
#32840=CARTESIAN_POINT('Ctrl Pts',(76.0585413582559,81.4736806618775,208.666666666667));
#32841=CARTESIAN_POINT('Ctrl Pts',(75.420678500187,80.8055008151075,208.725));
#32842=CARTESIAN_POINT('Ctrl Pts',(75.680407792752,79.9190054525043,208.783333333333));
#32843=CARTESIAN_POINT('Ctrl Pts',(75.9401370853171,79.0325100899011,208.841666666667));
#32844=CARTESIAN_POINT('Ctrl Pts',(76.8377292359511,78.8141945740679,208.9));
#32845=CARTESIAN_POINT('Ctrl Pts',(77.7353213865851,78.5958790582346,208.958333333333));
#32846=CARTESIAN_POINT('Ctrl Pts',(78.3731842446541,79.2640589050045,209.016666666667));
#32847=CARTESIAN_POINT('Ctrl Pts',(79.011047102723,79.9322387517744,209.075));
#32848=CARTESIAN_POINT('Ctrl Pts',(78.7513178101579,80.8187341143776,209.133333333333));
#32849=CARTESIAN_POINT('Ctrl Pts',(78.4915885175928,81.7052294769808,209.191666666667));
#32850=CARTESIAN_POINT('Ctrl Pts',(77.5939963669589,81.9235449928141,209.25));
#32851=CARTESIAN_POINT('Ctrl Pts',(76.6964042163248,82.1418605086474,209.308333333333));
#32852=CARTESIAN_POINT('Ctrl Pts',(76.0585413582559,81.4736806618775,209.366666666667));
#32853=CARTESIAN_POINT('Ctrl Pts',(75.420678500187,80.8055008151075,209.425));
#32854=CARTESIAN_POINT('Ctrl Pts',(75.680407792752,79.9190054525043,209.483333333333));
#32855=CARTESIAN_POINT('Ctrl Pts',(75.9401370853171,79.0325100899011,209.541666666667));
#32856=CARTESIAN_POINT('Ctrl Pts',(76.8377292359511,78.8141945740679,209.6));
#32857=CARTESIAN_POINT('Ctrl Pts',(77.7353213865851,78.5958790582346,209.658333333333));
#32858=CARTESIAN_POINT('Ctrl Pts',(78.3731842446541,79.2640589050045,209.716666666667));
#32859=CARTESIAN_POINT('Ctrl Pts',(79.011047102723,79.9322387517744,209.775));
#32860=CARTESIAN_POINT('Ctrl Pts',(78.7513178101579,80.8187341143776,209.833333333333));
#32861=CARTESIAN_POINT('Ctrl Pts',(78.4915885175928,81.7052294769808,209.891666666667));
#32862=CARTESIAN_POINT('Ctrl Pts',(77.5939963669589,81.9235449928141,209.95));
#32863=CARTESIAN_POINT('Ctrl Pts',(76.6964042163248,82.1418605086474,210.008333333333));
#32864=CARTESIAN_POINT('Ctrl Pts',(76.0585413582559,81.4736806618775,210.066666666667));
#32865=CARTESIAN_POINT('Ctrl Pts',(75.420678500187,80.8055008151075,210.125));
#32866=CARTESIAN_POINT('Ctrl Pts',(75.680407792752,79.9190054525043,210.183333333333));
#32867=CARTESIAN_POINT('Ctrl Pts',(75.9401370853171,79.0325100899011,210.241666666667));
#32868=CARTESIAN_POINT('Ctrl Pts',(76.8377292359511,78.8141945740679,210.3));
#32869=CARTESIAN_POINT('Ctrl Pts',(77.7353213865851,78.5958790582346,210.358333333333));
#32870=CARTESIAN_POINT('Ctrl Pts',(78.3731842446541,79.2640589050045,210.416666666667));
#32871=CARTESIAN_POINT('Ctrl Pts',(79.011047102723,79.9322387517744,210.475));
#32872=CARTESIAN_POINT('Ctrl Pts',(78.7513178101579,80.8187341143776,210.533333333333));
#32873=CARTESIAN_POINT('Ctrl Pts',(78.4915885175928,81.7052294769808,210.591666666667));
#32874=CARTESIAN_POINT('Ctrl Pts',(77.5939963669589,81.9235449928141,210.65));
#32875=CARTESIAN_POINT('Ctrl Pts',(76.6964042163248,82.1418605086474,210.708333333333));
#32876=CARTESIAN_POINT('Ctrl Pts',(76.0585413582559,81.4736806618775,210.766666666667));
#32877=CARTESIAN_POINT('Ctrl Pts',(75.420678500187,80.8055008151075,210.825));
#32878=CARTESIAN_POINT('Ctrl Pts',(75.680407792752,79.9190054525043,210.883333333333));
#32879=CARTESIAN_POINT('Ctrl Pts',(75.9401370853171,79.0325100899011,210.941666666667));
#32880=CARTESIAN_POINT('Ctrl Pts',(76.8377292359511,78.8141945740679,211.));
#32881=CARTESIAN_POINT('Ctrl Pts',(77.7353213865851,78.5958790582346,211.058333333333));
#32882=CARTESIAN_POINT('Ctrl Pts',(78.3731842446541,79.2640589050045,211.116666666667));
#32883=CARTESIAN_POINT('Ctrl Pts',(79.011047102723,79.9322387517744,211.175));
#32884=CARTESIAN_POINT('Ctrl Pts',(78.7513178101579,80.8187341143776,211.233333333333));
#32885=CARTESIAN_POINT('Ctrl Pts',(78.4915885175928,81.7052294769808,211.291666666667));
#32886=CARTESIAN_POINT('Ctrl Pts',(77.5939963669589,81.9235449928141,211.35));
#32887=CARTESIAN_POINT('Ctrl Pts',(76.6964042163248,82.1418605086474,211.408333333333));
#32888=CARTESIAN_POINT('Ctrl Pts',(76.0585413582559,81.4736806618775,211.466666666667));
#32889=CARTESIAN_POINT('Ctrl Pts',(75.420678500187,80.8055008151075,211.525));
#32890=CARTESIAN_POINT('Ctrl Pts',(75.680407792752,79.9190054525043,211.583333333333));
#32891=CARTESIAN_POINT('Ctrl Pts',(75.9401370853171,79.0325100899011,211.641666666667));
#32892=CARTESIAN_POINT('Ctrl Pts',(76.8377292359511,78.8141945740679,211.7));
#32893=CARTESIAN_POINT('',(76.8377292359511,78.8141945740679,197.7));
#32894=CARTESIAN_POINT('',(76.882500972401,78.9982710885302,197.809374999522));
#32895=CARTESIAN_POINT('',(76.882500972401,78.9982710885302,211.809374999522));
#32896=CARTESIAN_POINT('Ctrl Pts',(76.8377292359511,78.8141945740678,211.));
#32897=CARTESIAN_POINT('Ctrl Pts',(76.7421956368437,78.837430591622,210.993791397042));
#32898=CARTESIAN_POINT('Ctrl Pts',(76.6488078291848,78.8694683758089,210.987252804374));
#32899=CARTESIAN_POINT('Ctrl Pts',(76.3697606459006,78.9951613331449,210.966206582705));
#32900=CARTESIAN_POINT('Ctrl Pts',(76.1991296043222,79.1161951267954,210.951113087222));
#32901=CARTESIAN_POINT('Ctrl Pts',(75.9100735650893,79.4202005198414,210.920561039534));
#32902=CARTESIAN_POINT('Ctrl Pts',(75.7958364286097,79.6016502668059,210.905399990094));
#32903=CARTESIAN_POINT('Ctrl Pts',(75.6482827813348,79.9896598075252,210.878081571274));
#32904=CARTESIAN_POINT('Ctrl Pts',(75.6128796701455,80.191143614408,210.865215738096));
#32905=CARTESIAN_POINT('Ctrl Pts',(75.6193462602684,80.6035916812702,210.835881909083));
#32906=CARTESIAN_POINT('Ctrl Pts',(75.6638079674599,80.8105491249732,210.82045255689));
#32907=CARTESIAN_POINT('Ctrl Pts',(75.8314666514945,81.1989094692805,210.790047602273));
#32908=CARTESIAN_POINT('Ctrl Pts',(75.9543114774069,81.3758154595951,210.775966565719));
#32909=CARTESIAN_POINT('Ctrl Pts',(76.255656315336,81.6649371807569,210.748952445063));
#32910=CARTESIAN_POINT('Ctrl Pts',(76.4288855612612,81.7768509112186,210.73453628646));
#32911=CARTESIAN_POINT('Ctrl Pts',(76.8153671419507,81.9324155231772,210.70430284673));
#32912=CARTESIAN_POINT('Ctrl Pts',(77.0261552911063,81.9717112472583,210.688747285219));
#32913=CARTESIAN_POINT('Ctrl Pts',(77.4444681194566,81.9657981638116,210.659597004652));
#32914=CARTESIAN_POINT('Ctrl Pts',(77.6478918569701,81.9231498342464,210.647137520362));
#32915=CARTESIAN_POINT('Ctrl Pts',(78.0282269886831,81.762722375082,210.619000254481));
#32916=CARTESIAN_POINT('Ctrl Pts',(78.2013501921092,81.6461904160994,210.604001981035));
#32917=CARTESIAN_POINT('Ctrl Pts',(78.4975778231958,81.3498282284663,210.573456516786));
#32918=CARTESIAN_POINT('Ctrl Pts',(78.6163205365602,81.1712592597555,210.558202877509));
#32919=CARTESIAN_POINT('Ctrl Pts',(78.7735690054945,80.7868720228714,210.530555510445));
#32920=CARTESIAN_POINT('Ctrl Pts',(78.8139767093485,80.5861890491931,210.517937042288));
#32921=CARTESIAN_POINT('Ctrl Pts',(78.8176755362887,80.1740840495194,210.488802697026));
#32922=CARTESIAN_POINT('Ctrl Pts',(78.7785249852346,79.9665967007589,210.473427325777));
#32923=CARTESIAN_POINT('Ctrl Pts',(78.6214269969712,79.5754662289674,210.443008093394));
#32924=CARTESIAN_POINT('Ctrl Pts',(78.503876463604,79.3962335317332,210.428521671259));
#32925=CARTESIAN_POINT('Ctrl Pts',(78.2117293575683,79.1000869433297,210.402007142167));
#32926=CARTESIAN_POINT('Ctrl Pts',(78.0421770439422,78.9836916635366,210.387756398436));
#32927=CARTESIAN_POINT('Ctrl Pts',(77.6613663356015,78.817631266407,210.357704598224));
#32928=CARTESIAN_POINT('Ctrl Pts',(77.4524279876431,78.7723536599372,210.342155838516));
#32929=CARTESIAN_POINT('Ctrl Pts',(77.1047144563197,78.7669488199961,210.317713719403));
#32930=CARTESIAN_POINT('Ctrl Pts',(76.9693379669327,78.7821842362188,210.308553078331));
#32931=CARTESIAN_POINT('Ctrl Pts',(76.8377292359507,78.814194574068,210.3));
#32932=CARTESIAN_POINT('Ctrl Pts',(76.8377292359511,78.8141945740679,197.7));
#32933=CARTESIAN_POINT('Ctrl Pts',(77.7353213865851,78.5958790582346,197.758333333333));
#32934=CARTESIAN_POINT('Ctrl Pts',(78.3731842446541,79.2640589050045,197.816666666667));
#32935=CARTESIAN_POINT('Ctrl Pts',(79.011047102723,79.9322387517744,197.875));
#32936=CARTESIAN_POINT('Ctrl Pts',(78.7513178101579,80.8187341143776,197.933333333333));
#32937=CARTESIAN_POINT('Ctrl Pts',(78.4915885175929,81.7052294769808,197.991666666667));
#32938=CARTESIAN_POINT('Ctrl Pts',(77.5939963669589,81.9235449928141,198.05));
#32939=CARTESIAN_POINT('Ctrl Pts',(77.2364435356502,82.0105102484145,198.073236888244));
#32940=CARTESIAN_POINT('Ctrl Pts',(76.8768229089103,81.9325359726461,198.1));
#32941=CARTESIAN_POINT('Origin',(76.882500972401,78.9982710885302,211.809374999522));
#32942=CARTESIAN_POINT('Origin',(76.882500972401,78.9982710885302,197.809374999522));
#32943=CARTESIAN_POINT('',(76.8377292359511,78.8141945740679,198.006249999044));
#32944=CARTESIAN_POINT('Origin',(77.2158628014545,80.368869783439,198.006249999044));
#32945=CARTESIAN_POINT('Origin',(77.215862801455,80.368869783441,211.6));
#32946=CARTESIAN_POINT('Origin',(77.2158628014545,80.368869783439,198.006249999044));
#32947=CARTESIAN_POINT('Origin',(77.215862801455,80.368869783441,198.1));
#32948=CARTESIAN_POINT('Origin',(77.215862801455,80.368869783441,211.6));
#32949=CARTESIAN_POINT('',(77.6885297583348,82.3122137951574,212.));
#32950=CARTESIAN_POINT('',(77.5939963669588,81.9235449928141,211.6));
#32951=CARTESIAN_POINT('Origin',(77.215862801455,80.368869783441,212.));
#32952=CARTESIAN_POINT('Origin',(77.215862801455,80.368869783441,197.7));
#32953=CARTESIAN_POINT('',(76.7431958445752,78.4255257717246,197.7));
#32954=CARTESIAN_POINT('',(76.7431958445752,78.4255257717246,197.7));
#32955=CARTESIAN_POINT('Origin',(77.215862801455,80.368869783441,197.7));
#32956=CARTESIAN_POINT('Origin',(77.215862801455,80.368869783441,198.1));
#32957=CARTESIAN_POINT('',(78.0666633238387,83.8668890045305,197.7));
#32958=CARTESIAN_POINT('',(78.1611967152146,84.2555578068738,198.1));
#32959=CARTESIAN_POINT('Origin',(77.215862801455,80.368869783441,197.7));
#32960=CARTESIAN_POINT('Origin',(77.215862801455,80.368869783441,212.));
#32961=CARTESIAN_POINT('',(76.2705288876953,76.4821817600082,211.6));
#32962=CARTESIAN_POINT('Origin',(77.215862801455,80.368869783441,211.6));
#32963=CARTESIAN_POINT('',(76.3650622790713,76.8708505623514,212.));
#32964=CARTESIAN_POINT('',(76.3650622790713,76.8708505623514,212.));
#32965=CARTESIAN_POINT('Origin',(77.215862801455,80.368869783441,212.));
#32966=CARTESIAN_POINT('Origin',(77.215862801455,80.368869783441,212.));
#32967=CARTESIAN_POINT('',(76.2705288876953,76.4821817600082,212.));
#32968=CARTESIAN_POINT('Origin',(77.215862801455,80.368869783441,197.7));
#32969=CARTESIAN_POINT('Origin',(77.215862801455,80.368869783441,212.));
#32970=CARTESIAN_POINT('Origin',(77.215862801455,80.368869783441,212.));
#36652=UNCERTAINTY_MEASURE_WITH_UNIT(LENGTH_MEASURE(0.01),#36669,
'DISTANCE_ACCURACY_VALUE',
'Maximum model space distance between geometric entities at asserted c
onnectivities');
#36656=UNCERTAINTY_MEASURE_WITH_UNIT(LENGTH_MEASURE(0.01),#36669,
'DISTANCE_ACCURACY_VALUE',
'Maximum model space distance between geometric entities at asserted c
onnectivities');
#36664=(
GEOMETRIC_REPRESENTATION_CONTEXT(3)
GLOBAL_UNCERTAINTY_ASSIGNED_CONTEXT((#36652))
GLOBAL_UNIT_ASSIGNED_CONTEXT((#36669,#36671,#36672))
REPRESENTATION_CONTEXT('','3D')
);
#36668=(
GEOMETRIC_REPRESENTATION_CONTEXT(3)
GLOBAL_UNCERTAINTY_ASSIGNED_CONTEXT((#36656))
GLOBAL_UNIT_ASSIGNED_CONTEXT((#36669,#36671,#36672))
REPRESENTATION_CONTEXT('','3D')
);
#36669=(
LENGTH_UNIT()
NAMED_UNIT(*)
SI_UNIT(.MILLI.,.METRE.)
);
#36671=(
NAMED_UNIT(*)
PLANE_ANGLE_UNIT()
SI_UNIT($,.RADIAN.)
);
#36672=(
NAMED_UNIT(*)
SI_UNIT($,.STERADIAN.)
SOLID_ANGLE_UNIT()
);
#36680=SHAPE_DEFINITION_REPRESENTATION(#36691,#36712);
#36691=PRODUCT_DEFINITION_SHAPE('',$,#36724);
#36712=SHAPE_REPRESENTATION('',(#18787),#36664);
#36716=PRODUCT_DEFINITION_CONTEXT('part definition',#36751,'design');
#36724=PRODUCT_DEFINITION('Sprocket Tape Drive Gear',
'Sprocket Tape Drive Gear',#36735,#36716);
#36735=PRODUCT_DEFINITION_FORMATION('',$,#36760);
#36751=APPLICATION_CONTEXT(
'Core Data for Automotive Mechanical Design Process');
#36752=PRODUCT_CONTEXT('part definition',#36751,'mechanical');
#36760=PRODUCT('Sprocket Tape Drive Gear','Sprocket Tape Drive Gear',$,
(#36752));
#36765=PRESENTATION_STYLE_ASSIGNMENT((#36772));
#36772=SURFACE_STYLE_USAGE(.BOTH.,#36779);
#36779=SURFACE_SIDE_STYLE('',(#36786));
#36786=SURFACE_STYLE_FILL_AREA(#36793);
#36793=FILL_AREA_STYLE('Opaque(23,69,131)',(#36800));
#36800=FILL_AREA_STYLE_COLOUR('Opaque(23,69,131)',#36807);
#36807=COLOUR_RGB('Opaque(23,69,131)',0.0901960784313725,0.270588235294118,
0.513725490196078);
ENDSEC;
END-ISO-10303-21;
